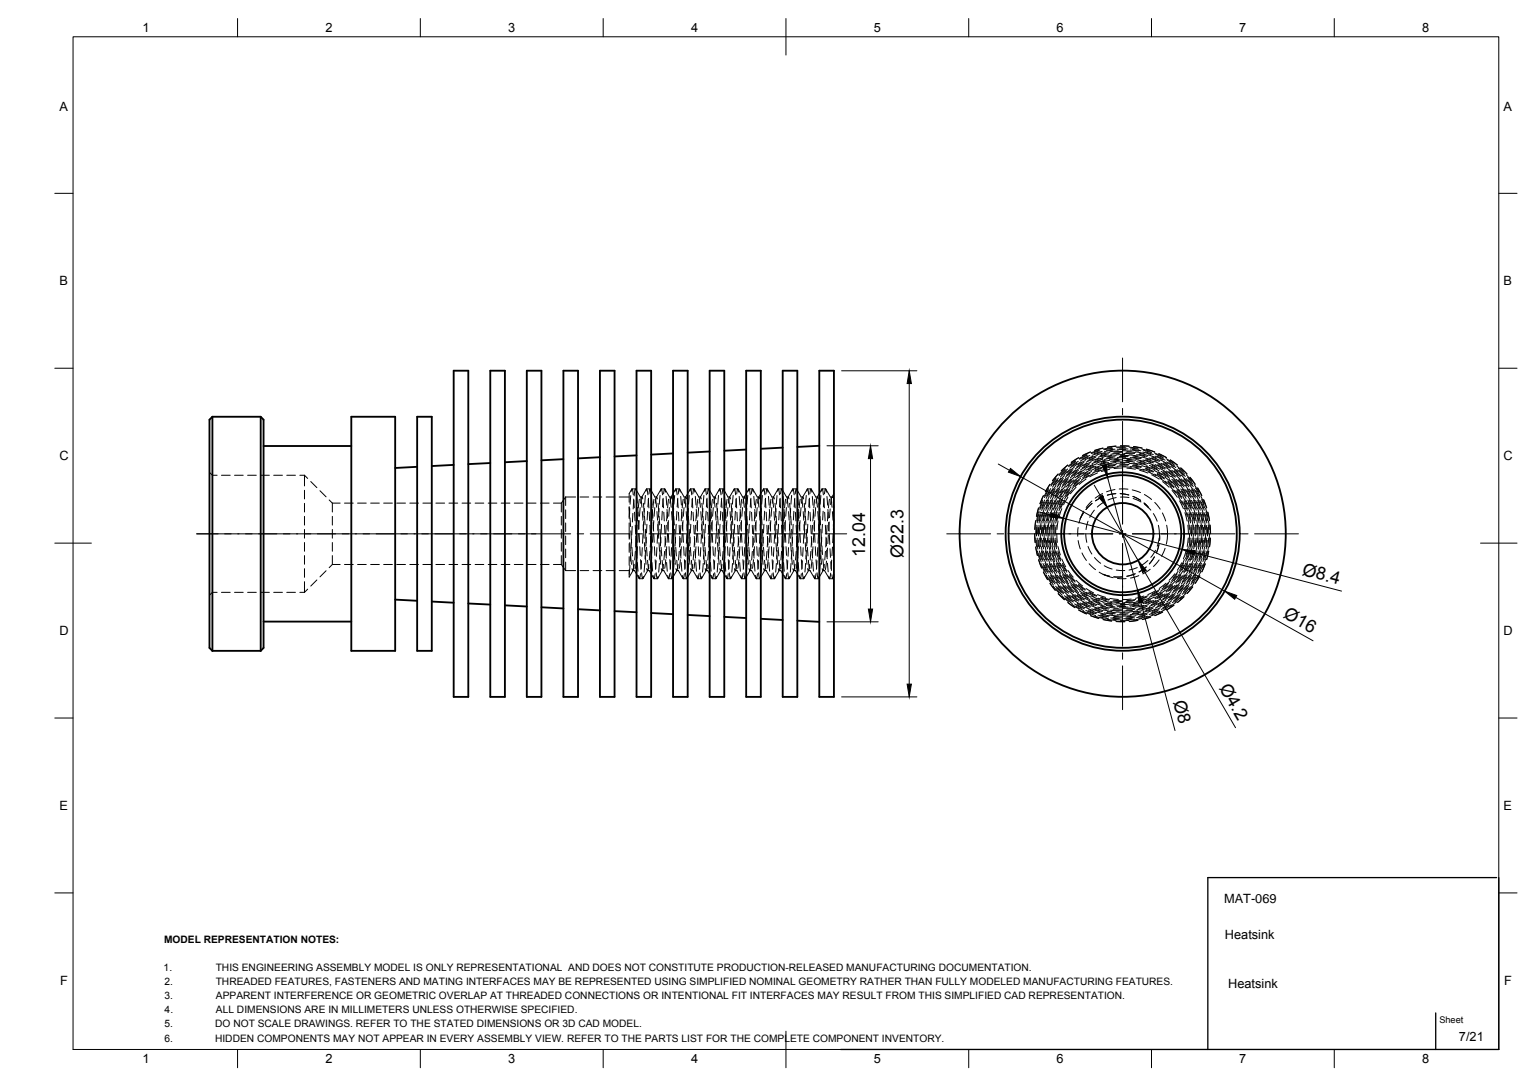
ISO-10303-21;
HEADER;
/* Generated by software containing ST-Developer
 * from STEP Tools, Inc. (www.steptools.com) 
 */

FILE_DESCRIPTION(
/* description */ ('CAx-IF Rec.Pracs.---Representation and Presentation of Product Manufa
cturing Information (PMI)---4.0---2014-10-13'),
/* implementation_level */ '2;1');

FILE_NAME(
/* name */ 'Heatsink.step',
/* time_stamp */ '2026-10-24T15:08:39-07:00',
/* author */ (''),
/* organization */ (''),
/* preprocessor_version */ 'ST-DEVELOPER v20.2',
/* originating_system */ 'Autodesk Translation Framework v15.17.0.0',
/* authorisation */ '');

FILE_SCHEMA (('AP242_MANAGED_MODEL_BASED_3D_ENGINEERING_MIM_LF { 1 0 10303 442 2 1 4 }'));
ENDSEC;

DATA;
#10=MECHANICAL_DESIGN_GEOMETRIC_PRESENTATION_REPRESENTATION('',(#824),#50081);
#94=B_SPLINE_SURFACE_WITH_KNOTS('',3,3,((#16932,#16933,#16934,#16935,#16936,
#16937,#16938,#16939,#16940,#16941,#16942,#16943,#16944,#16945,#16946,#16947,
#16948,#16949,#16950,#16951,#16952,#16953,#16954,#16955,#16956,#16957,#16958,
#16959,#16960,#16961,#16962,#16963,#16964,#16965,#16966,#16967,#16968,#16969,
#16970,#16971,#16972,#16973,#16974,#16975,#16976,#16977,#16978,#16979,#16980,
#16981,#16982,#16983,#16984,#16985,#16986,#16987,#16988,#16989,#16990,#16991,
#16992,#16993,#16994,#16995,#16996,#16997,#16998,#16999,#17000,#17001,#17002,
#17003,#17004,#17005,#17006,#17007,#17008,#17009,#17010,#17011,#17012,#17013,
#17014,#17015,#17016,#17017,#17018,#17019,#17020,#17021,#17022,#17023,#17024),
(#17025,#17026,#17027,#17028,#17029,#17030,#17031,#17032,#17033,#17034,
#17035,#17036,#17037,#17038,#17039,#17040,#17041,#17042,#17043,#17044,#17045,
#17046,#17047,#17048,#17049,#17050,#17051,#17052,#17053,#17054,#17055,#17056,
#17057,#17058,#17059,#17060,#17061,#17062,#17063,#17064,#17065,#17066,#17067,
#17068,#17069,#17070,#17071,#17072,#17073,#17074,#17075,#17076,#17077,#17078,
#17079,#17080,#17081,#17082,#17083,#17084,#17085,#17086,#17087,#17088,#17089,
#17090,#17091,#17092,#17093,#17094,#17095,#17096,#17097,#17098,#17099,#17100,
#17101,#17102,#17103,#17104,#17105,#17106,#17107,#17108,#17109,#17110,#17111,
#17112,#17113,#17114,#17115,#17116,#17117),(#17118,#17119,#17120,#17121,
#17122,#17123,#17124,#17125,#17126,#17127,#17128,#17129,#17130,#17131,#17132,
#17133,#17134,#17135,#17136,#17137,#17138,#17139,#17140,#17141,#17142,#17143,
#17144,#17145,#17146,#17147,#17148,#17149,#17150,#17151,#17152,#17153,#17154,
#17155,#17156,#17157,#17158,#17159,#17160,#17161,#17162,#17163,#17164,#17165,
#17166,#17167,#17168,#17169,#17170,#17171,#17172,#17173,#17174,#17175,#17176,
#17177,#17178,#17179,#17180,#17181,#17182,#17183,#17184,#17185,#17186,#17187,
#17188,#17189,#17190,#17191,#17192,#17193,#17194,#17195,#17196,#17197,#17198,
#17199,#17200,#17201,#17202,#17203,#17204,#17205,#17206,#17207,#17208,#17209,
#17210),(#17211,#17212,#17213,#17214,#17215,#17216,#17217,#17218,#17219,
#17220,#17221,#17222,#17223,#17224,#17225,#17226,#17227,#17228,#17229,#17230,
#17231,#17232,#17233,#17234,#17235,#17236,#17237,#17238,#17239,#17240,#17241,
#17242,#17243,#17244,#17245,#17246,#17247,#17248,#17249,#17250,#17251,#17252,
#17253,#17254,#17255,#17256,#17257,#17258,#17259,#17260,#17261,#17262,#17263,
#17264,#17265,#17266,#17267,#17268,#17269,#17270,#17271,#17272,#17273,#17274,
#17275,#17276,#17277,#17278,#17279,#17280,#17281,#17282,#17283,#17284,#17285,
#17286,#17287,#17288,#17289,#17290,#17291,#17292,#17293,#17294,#17295,#17296,
#17297,#17298,#17299,#17300,#17301,#17302,#17303)),.UNSPECIFIED.,.F.,.F.,
 .F.,(4,4),(4,1,1,1,1,1,1,1,1,1,1,1,1,1,1,1,1,1,1,1,1,1,1,1,1,1,1,1,1,1,
1,1,1,1,1,1,1,1,1,1,1,1,1,1,1,1,1,1,1,1,1,1,1,1,1,1,1,1,1,1,1,1,1,1,1,1,
1,1,1,1,1,1,1,1,1,1,1,1,1,1,1,1,1,1,1,1,1,1,1,1,4),(-0.000398919436546387,
0.0651101464894062),(10.2099830649134,11.2099710040949,12.2097658840232,
13.2095607639514,14.2093556438797,15.2091505238079,16.2089454037362,17.2087402836644,
18.2085351635927,19.208330043521,20.2081249234492,21.2079198033775,22.2077146833057,
23.207509563234,24.2073044431622,25.2070993230905,26.2068942030187,27.206689082947,
28.2064839628752,29.2062788428035,30.2060737227317,31.20586860266,32.2056634825882,
33.2054583625165,34.2052532424447,35.205048122373,36.2048430023012,37.2046378822295,
38.2044327621577,39.204227642086,40.2040225220142,41.2038174019425,42.2036122818707,
43.203407161799,44.2032020417273,45.2029969216555,46.2027918015838,47.202586681512,
48.2023815614403,49.2021764413685,50.2019713212968,51.201766201225,52.2015610811533,
53.2013559610815,54.2011508410098,55.200945720938,56.2007406008663,57.2005354807945,
58.2003303607228,59.200125240651,60.1999201205793,61.1997150005075,62.1995098804358,
63.199304760364,64.1990996402923,65.1988945202205,66.1986894001488,67.1984842800771,
68.1982791600053,69.1980740399336,70.1978689198618,71.1976637997901,72.1974586797183,
73.1972535596466,74.1970484395748,75.1968433195031,76.1966381994313,77.1964330793596,
78.1962279592878,79.1960228392161,80.1958177191443,81.1956125990726,82.1954074790008,
83.1952023589291,84.1949972388573,85.1947921187856,86.1945869987138,87.1943818786421,
88.1941767585704,89.1939716384986,90.1937665184269,91.1935613983551,92.1933562782833,
93.1931511582116,94.1929460381399,95.1927409180681,96.1925357979964,97.1923306779246,
98.1921255578529,99.1919204377811,100.192067891578),.UNSPECIFIED.);
#95=B_SPLINE_SURFACE_WITH_KNOTS('',3,3,((#17371,#17372,#17373,#17374,#17375,
#17376,#17377,#17378,#17379,#17380,#17381,#17382,#17383,#17384,#17385,#17386,
#17387,#17388,#17389,#17390,#17391,#17392,#17393,#17394,#17395,#17396,#17397,
#17398,#17399,#17400,#17401,#17402,#17403,#17404,#17405,#17406,#17407,#17408,
#17409,#17410,#17411,#17412,#17413,#17414,#17415,#17416,#17417,#17418,#17419,
#17420,#17421,#17422,#17423,#17424,#17425,#17426,#17427,#17428,#17429,#17430,
#17431,#17432,#17433,#17434,#17435,#17436,#17437,#17438,#17439,#17440,#17441,
#17442,#17443,#17444,#17445,#17446,#17447,#17448,#17449,#17450,#17451,#17452,
#17453,#17454,#17455,#17456,#17457,#17458,#17459,#17460,#17461,#17462,#17463),
(#17464,#17465,#17466,#17467,#17468,#17469,#17470,#17471,#17472,#17473,
#17474,#17475,#17476,#17477,#17478,#17479,#17480,#17481,#17482,#17483,#17484,
#17485,#17486,#17487,#17488,#17489,#17490,#17491,#17492,#17493,#17494,#17495,
#17496,#17497,#17498,#17499,#17500,#17501,#17502,#17503,#17504,#17505,#17506,
#17507,#17508,#17509,#17510,#17511,#17512,#17513,#17514,#17515,#17516,#17517,
#17518,#17519,#17520,#17521,#17522,#17523,#17524,#17525,#17526,#17527,#17528,
#17529,#17530,#17531,#17532,#17533,#17534,#17535,#17536,#17537,#17538,#17539,
#17540,#17541,#17542,#17543,#17544,#17545,#17546,#17547,#17548,#17549,#17550,
#17551,#17552,#17553,#17554,#17555,#17556),(#17557,#17558,#17559,#17560,
#17561,#17562,#17563,#17564,#17565,#17566,#17567,#17568,#17569,#17570,#17571,
#17572,#17573,#17574,#17575,#17576,#17577,#17578,#17579,#17580,#17581,#17582,
#17583,#17584,#17585,#17586,#17587,#17588,#17589,#17590,#17591,#17592,#17593,
#17594,#17595,#17596,#17597,#17598,#17599,#17600,#17601,#17602,#17603,#17604,
#17605,#17606,#17607,#17608,#17609,#17610,#17611,#17612,#17613,#17614,#17615,
#17616,#17617,#17618,#17619,#17620,#17621,#17622,#17623,#17624,#17625,#17626,
#17627,#17628,#17629,#17630,#17631,#17632,#17633,#17634,#17635,#17636,#17637,
#17638,#17639,#17640,#17641,#17642,#17643,#17644,#17645,#17646,#17647,#17648,
#17649),(#17650,#17651,#17652,#17653,#17654,#17655,#17656,#17657,#17658,
#17659,#17660,#17661,#17662,#17663,#17664,#17665,#17666,#17667,#17668,#17669,
#17670,#17671,#17672,#17673,#17674,#17675,#17676,#17677,#17678,#17679,#17680,
#17681,#17682,#17683,#17684,#17685,#17686,#17687,#17688,#17689,#17690,#17691,
#17692,#17693,#17694,#17695,#17696,#17697,#17698,#17699,#17700,#17701,#17702,
#17703,#17704,#17705,#17706,#17707,#17708,#17709,#17710,#17711,#17712,#17713,
#17714,#17715,#17716,#17717,#17718,#17719,#17720,#17721,#17722,#17723,#17724,
#17725,#17726,#17727,#17728,#17729,#17730,#17731,#17732,#17733,#17734,#17735,
#17736,#17737,#17738,#17739,#17740,#17741,#17742)),.UNSPECIFIED.,.F.,.F.,
 .F.,(4,4),(4,1,1,1,1,1,1,1,1,1,1,1,1,1,1,1,1,1,1,1,1,1,1,1,1,1,1,1,1,1,
1,1,1,1,1,1,1,1,1,1,1,1,1,1,1,1,1,1,1,1,1,1,1,1,1,1,1,1,1,1,1,1,1,1,1,1,
1,1,1,1,1,1,1,1,1,1,1,1,1,1,1,1,1,1,1,1,1,1,1,1,4),(-0.00100526872732246,
0.0646023829588572),(13.6909080459636,14.6908132548486,15.6906081347769,
16.6904030147051,17.6901978946334,18.6899927745616,19.6897876544899,20.6895825344181,
21.6893774143464,22.6891722942746,23.6889671742029,24.6887620541311,25.6885569340594,
26.6883518139876,27.6881466939159,28.6879415738441,29.6877364537724,30.6875313337007,
31.6873262136289,32.6871210935572,33.6869159734854,34.6867108534137,35.6865057333419,
36.6863006132702,37.6860954931984,38.6858903731267,39.6856852530549,40.6854801329832,
41.6852750129114,42.6850698928397,43.6848647727679,44.6846596526962,45.6844545326244,
46.6842494125527,47.6840442924809,48.6838391724092,49.6836340523375,50.6834289322657,
51.683223812194,52.6830186921222,53.6828135720505,54.6826084519787,55.682403331907,
56.6821982118352,57.6819930917635,58.6817879716917,59.68158285162,60.6813777315482,
61.6811726114765,62.6809674914047,63.680762371333,64.6805572512612,65.6803521311895,
66.6801470111178,67.679941891046,68.6797367709743,69.6795316509025,70.6793265308308,
71.679121410759,72.6789162906873,73.6787111706155,74.6785060505438,75.678300930472,
76.6780958104003,77.6778906903285,78.6776855702568,79.677480450185,80.6772753301133,
81.6770702100415,82.6768650899698,83.676659969898,84.6764548498263,85.6762497297545,
86.6760446096828,87.6758394896111,88.6756343695393,89.6754292494676,90.6752241293958,
91.6750190093241,92.6748138892523,93.6746087691806,94.6744036491088,95.6741985290371,
96.6739934089653,97.6737882888936,98.6735831688218,99.6733780487501,100.673172928678,
101.672967808607,102.672762688535,103.67278623601),.UNSPECIFIED.);
#141=B_SPLINE_CURVE_WITH_KNOTS('',3,(#13868,#13869,#13870,#13871,#13872,
#13873,#13874,#13875,#13876,#13877,#13878,#13879,#13880,#13881,#13882,#13883,
#13884,#13885,#13886,#13887,#13888,#13889,#13890,#13891,#13892,#13893,#13894,
#13895,#13896,#13897,#13898,#13899,#13900,#13901,#13902,#13903,#13904,#13905,
#13906,#13907,#13908,#13909,#13910,#13911,#13912,#13913,#13914,#13915,#13916,
#13917,#13918,#13919,#13920,#13921,#13922,#13923,#13924,#13925,#13926,#13927,
#13928,#13929,#13930,#13931,#13932,#13933,#13934),.UNSPECIFIED.,.F.,.F.,
(4,3,3,3,3,3,3,3,3,3,3,3,3,3,3,3,3,3,3,3,3,3,4),(1.25156093680116E-6,0.0883500955934641,
0.103030521980099,0.125,0.211544670578705,0.25,0.26221619397553,0.334021572169558,
0.375,0.421693572098901,0.485226135902788,0.5,0.5625,0.577874060665358,
0.625,0.710303391755808,0.734738255635071,0.75,0.836904432795506,0.875,
0.895553090245324,0.965961016411946,0.99999868984544),.UNSPECIFIED.);
#142=B_SPLINE_CURVE_WITH_KNOTS('',3,(#13936,#13937,#13938,#13939,#13940,
#13941,#13942,#13943,#13944,#13945,#13946,#13947,#13948,#13949,#13950,#13951,
#13952,#13953,#13954,#13955,#13956,#13957,#13958,#13959,#13960,#13961,#13962,
#13963,#13964,#13965,#13966,#13967,#13968,#13969,#13970,#13971,#13972,#13973,
#13974,#13975,#13976,#13977,#13978,#13979,#13980,#13981,#13982,#13983,#13984),
 .UNSPECIFIED.,.F.,.F.,(4,3,3,3,3,3,3,3,3,3,3,3,3,3,3,3,4),(0.,0.0880924990179859,
0.125,0.211469534154412,0.25,0.336789345136967,0.375,0.461773033582195,
0.5,0.586773033582203,0.625,0.711789345136965,0.75,0.836469534154423,0.875,
0.963092499017944,1.),.UNSPECIFIED.);
#143=B_SPLINE_CURVE_WITH_KNOTS('',3,(#13986,#13987,#13988,#13989,#13990,
#13991,#13992,#13993,#13994,#13995,#13996,#13997,#13998,#13999,#14000,#14001,
#14002,#14003,#14004,#14005,#14006,#14007,#14008,#14009,#14010,#14011,#14012,
#14013,#14014,#14015,#14016,#14017,#14018,#14019,#14020,#14021,#14022,#14023,
#14024,#14025,#14026,#14027,#14028,#14029,#14030,#14031,#14032,#14033,#14034),
 .UNSPECIFIED.,.F.,.F.,(4,3,3,3,3,3,3,3,3,3,3,3,3,3,3,3,4),(0.,0.0881024108360804,
0.125,0.211479598204264,0.25,0.336799405951737,0.375,0.461783076602685,
0.5,0.586783076602703,0.625,0.711799405951738,0.75,0.836479598204259,0.875,
0.963102410836136,1.),.UNSPECIFIED.);
#144=B_SPLINE_CURVE_WITH_KNOTS('',3,(#14036,#14037,#14038,#14039,#14040,
#14041,#14042,#14043,#14044,#14045,#14046,#14047,#14048,#14049,#14050,#14051,
#14052,#14053,#14054,#14055,#14056,#14057,#14058,#14059,#14060,#14061,#14062,
#14063,#14064,#14065,#14066,#14067,#14068,#14069,#14070,#14071,#14072,#14073,
#14074,#14075,#14076,#14077,#14078,#14079,#14080,#14081,#14082,#14083,#14084),
 .UNSPECIFIED.,.F.,.F.,(4,3,3,3,3,3,3,3,3,3,3,3,3,3,3,3,4),(0.,0.0880833098674038,
0.125,0.211460203849926,0.25,0.336780017823431,0.375,0.461763722773403,
0.5,0.586763722773395,0.625,0.71178001782344,0.75,0.836460203849939,0.875,
0.963083309867389,1.),.UNSPECIFIED.);
#145=B_SPLINE_CURVE_WITH_KNOTS('',3,(#14086,#14087,#14088,#14089,#14090,
#14091,#14092,#14093,#14094,#14095,#14096,#14097,#14098,#14099,#14100,#14101,
#14102,#14103,#14104,#14105,#14106,#14107,#14108,#14109,#14110,#14111,#14112,
#14113,#14114,#14115,#14116,#14117,#14118,#14119,#14120,#14121,#14122,#14123,
#14124,#14125,#14126,#14127,#14128,#14129,#14130,#14131,#14132,#14133,#14134),
 .UNSPECIFIED.,.F.,.F.,(4,3,3,3,3,3,3,3,3,3,3,3,3,3,3,3,4),(1.38656343410957E-7,
0.0880826036576598,0.125,0.211459358145887,0.25,0.336779172390087,0.375,
0.461762878836428,0.5,0.586762878836416,0.625,0.711779172390097,0.75,0.836459358145886,
0.875,0.963082476958599,1.),.UNSPECIFIED.);
#146=B_SPLINE_CURVE_WITH_KNOTS('',3,(#14136,#14137,#14138,#14139,#14140,
#14141,#14142,#14143,#14144,#14145,#14146,#14147,#14148,#14149,#14150,#14151,
#14152,#14153,#14154,#14155,#14156,#14157,#14158,#14159,#14160,#14161,#14162,
#14163,#14164,#14165,#14166,#14167,#14168,#14169,#14170,#14171,#14172,#14173,
#14174,#14175,#14176,#14177,#14178,#14179,#14180,#14181,#14182,#14183,#14184),
 .UNSPECIFIED.,.F.,.F.,(4,3,3,3,3,3,3,3,3,3,3,3,3,3,3,3,4),(0.,0.0881011169934676,
0.125,0.211478284491326,0.25,0.336798092661633,0.375,0.461781765634862,
0.5,0.586781765634871,0.625,0.711798092661628,0.75,0.836478284491337,0.875,
0.963101116993472,1.),.UNSPECIFIED.);
#147=B_SPLINE_CURVE_WITH_KNOTS('',3,(#14186,#14187,#14188,#14189,#14190,
#14191,#14192,#14193,#14194,#14195,#14196,#14197,#14198,#14199,#14200,#14201,
#14202,#14203,#14204,#14205,#14206,#14207,#14208,#14209,#14210,#14211,#14212,
#14213,#14214,#14215,#14216,#14217,#14218,#14219,#14220,#14221,#14222,#14223,
#14224,#14225,#14226,#14227,#14228,#14229,#14230,#14231,#14232,#14233,#14234),
 .UNSPECIFIED.,.F.,.F.,(4,3,3,3,3,3,3,3,3,3,3,3,3,3,3,3,4),(0.,0.0880934980383074,
0.125,0.211470548519371,0.25,0.336790359176268,0.375,0.461774045827613,
0.5,0.586774045827619,0.625,0.711790359176272,0.75,0.836470548519377,0.875,
0.963093498038292,1.),.UNSPECIFIED.);
#148=B_SPLINE_CURVE_WITH_KNOTS('',3,(#14236,#14237,#14238,#14239,#14240,
#14241,#14242,#14243,#14244,#14245,#14246,#14247,#14248,#14249,#14250,#14251,
#14252,#14253,#14254,#14255,#14256,#14257,#14258,#14259,#14260,#14261,#14262,
#14263,#14264,#14265,#14266,#14267,#14268,#14269,#14270,#14271,#14272,#14273,
#14274,#14275,#14276,#14277,#14278,#14279,#14280,#14281,#14282,#14283,#14284),
 .UNSPECIFIED.,.F.,.F.,(4,3,3,3,3,3,3,3,3,3,3,3,3,3,3,3,4),(1.23038810336374E-6,
0.0880827430507262,0.125,0.211461811736442,0.25,0.336784839496599,0.375,
0.461710040665769,0.5,0.586886602165314,0.625,0.711701462151024,0.75,0.836461636546894,
0.875,0.963080200121549,0.999998752114935),.UNSPECIFIED.);
#149=B_SPLINE_CURVE_WITH_KNOTS('',3,(#14286,#14287,#14288,#14289,#14290,
#14291,#14292,#14293,#14294,#14295,#14296,#14297,#14298,#14299,#14300,#14301,
#14302,#14303,#14304,#14305,#14306,#14307,#14308,#14309,#14310,#14311,#14312,
#14313,#14314,#14315,#14316,#14317,#14318,#14319,#14320,#14321,#14322,#14323,
#14324,#14325,#14326,#14327,#14328,#14329,#14330,#14331,#14332,#14333,#14334),
 .UNSPECIFIED.,.F.,.F.,(4,3,3,3,3,3,3,3,3,3,3,3,3,3,3,3,4),(0.,0.0880920072316036,
0.125,0.211469034814287,0.25,0.336788845957097,0.375,0.46177253528545,0.5,
0.586772535285452,0.625,0.711788845957101,0.75,0.836469034814284,0.875,
0.963092007231635,1.),.UNSPECIFIED.);
#150=B_SPLINE_CURVE_WITH_KNOTS('',3,(#14336,#14337,#14338,#14339,#14340,
#14341,#14342,#14343,#14344,#14345,#14346,#14347,#14348,#14349,#14350,#14351,
#14352,#14353,#14354,#14355,#14356,#14357,#14358,#14359,#14360,#14361,#14362,
#14363,#14364,#14365,#14366,#14367,#14368,#14369,#14370,#14371,#14372,#14373,
#14374,#14375,#14376,#14377,#14378,#14379,#14380,#14381,#14382,#14383,#14384),
 .UNSPECIFIED.,.F.,.F.,(4,3,3,3,3,3,3,3,3,3,3,3,3,3,3,3,4),(0.,0.0881029814297449,
0.125,0.211480177560658,0.25,0.33679998512162,0.375,0.461783654748482,0.5,
0.586783654748484,0.625,0.711799985121625,0.75,0.836480177560661,0.875,
0.963102981429744,1.),.UNSPECIFIED.);
#151=B_SPLINE_CURVE_WITH_KNOTS('',3,(#14386,#14387,#14388,#14389,#14390,
#14391,#14392),.UNSPECIFIED.,.F.,.F.,(4,1,1,1,4),(0.,0.25,0.5,0.75,1.),
 .UNSPECIFIED.);
#152=B_SPLINE_CURVE_WITH_KNOTS('',3,(#14396,#14397,#14398,#14399,#14400,
#14401,#14402,#14403,#14404,#14405,#14406,#14407,#14408,#14409,#14410,#14411,
#14412,#14413,#14414,#14415,#14416,#14417,#14418,#14419,#14420,#14421,#14422,
#14423,#14424,#14425,#14426,#14427,#14428,#14429,#14430,#14431,#14432),
 .UNSPECIFIED.,.F.,.F.,(4,3,3,3,3,3,3,3,3,3,3,3,4),(0.,0.125,0.23032997709698,
0.25,0.375,0.46468733129745,0.5,0.625,0.699111355030774,0.75,0.875,0.933549171352441,
1.),.UNSPECIFIED.);
#153=B_SPLINE_CURVE_WITH_KNOTS('',3,(#14434,#14435,#14436,#14437,#14438,
#14439,#14440,#14441,#14442,#14443,#14444,#14445,#14446,#14447,#14448,#14449,
#14450,#14451,#14452,#14453,#14454,#14455,#14456,#14457,#14458,#14459,#14460,
#14461,#14462,#14463,#14464,#14465,#14466,#14467,#14468,#14469,#14470,#14471,
#14472,#14473,#14474,#14475,#14476,#14477,#14478,#14479,#14480,#14481,#14482),
 .UNSPECIFIED.,.F.,.F.,(4,3,3,3,3,3,3,3,3,3,3,3,3,3,3,3,4),(7.72207807885717E-7,
0.0880871484364614,0.125,0.211463406241229,0.25,0.336781091047344,0.375,
0.461774857659637,0.5,0.586773708011755,0.625,0.711753540165089,0.75,0.836456686852539,
0.875,0.963077282795441,0.999999115125707),.UNSPECIFIED.);
#154=B_SPLINE_CURVE_WITH_KNOTS('',3,(#14484,#14485,#14486,#14487,#14488,
#14489,#14490,#14491,#14492,#14493,#14494,#14495,#14496,#14497,#14498,#14499,
#14500,#14501,#14502,#14503,#14504,#14505,#14506,#14507,#14508,#14509,#14510,
#14511,#14512,#14513,#14514,#14515,#14516,#14517,#14518,#14519,#14520,#14521,
#14522,#14523,#14524,#14525,#14526,#14527,#14528,#14529,#14530,#14531,#14532),
 .UNSPECIFIED.,.F.,.F.,(4,3,3,3,3,3,3,3,3,3,3,3,3,3,3,3,4),(0.,0.088088017626471,
0.125,0.211464983927167,0.25,0.336784796369337,0.375,0.461768492862693,
0.5,0.586768492862716,0.625,0.711784796369325,0.75,0.836464983927168,0.875,
0.96308801762646,1.),.UNSPECIFIED.);
#155=B_SPLINE_CURVE_WITH_KNOTS('',3,(#14534,#14535,#14536,#14537,#14538,
#14539,#14540,#14541,#14542,#14543,#14544,#14545,#14546,#14547,#14548,#14549,
#14550,#14551,#14552,#14553,#14554,#14555,#14556,#14557,#14558,#14559,#14560,
#14561,#14562,#14563,#14564,#14565,#14566,#14567,#14568,#14569,#14570,#14571,
#14572,#14573,#14574,#14575,#14576,#14577,#14578,#14579,#14580,#14581,#14582),
 .UNSPECIFIED.,.F.,.F.,(4,3,3,3,3,3,3,3,3,3,3,3,3,3,3,3,4),(0.,0.0881042788052708,
0.125,0.211481494860136,0.25,0.336801301996907,0.375,0.461784969295354,
0.5,0.586784969295344,0.625,0.711801301996906,0.75,0.836481494860131,0.875,
0.963104278805279,1.),.UNSPECIFIED.);
#156=B_SPLINE_CURVE_WITH_KNOTS('',3,(#14584,#14585,#14586,#14587,#14588,
#14589,#14590,#14591,#14592,#14593,#14594,#14595,#14596,#14597,#14598,#14599,
#14600,#14601,#14602,#14603,#14604,#14605,#14606,#14607,#14608,#14609,#14610,
#14611,#14612,#14613,#14614,#14615,#14616,#14617,#14618,#14619,#14620,#14621,
#14622,#14623,#14624,#14625,#14626,#14627,#14628,#14629,#14630,#14631,#14632),
 .UNSPECIFIED.,.F.,.F.,(4,3,3,3,3,3,3,3,3,3,3,3,3,3,3,3,4),(0.,0.0880886602034345,
0.125,0.211465636374609,0.25,0.336785448607603,0.375,0.461769143946861,
0.5,0.586769143946859,0.625,0.711785448607598,0.75,0.83646563637461,0.875,
0.963088660203419,1.),.UNSPECIFIED.);
#157=B_SPLINE_CURVE_WITH_KNOTS('',3,(#14634,#14635,#14636,#14637,#14638,
#14639,#14640,#14641,#14642,#14643,#14644,#14645,#14646,#14647,#14648,#14649,
#14650,#14651,#14652,#14653,#14654,#14655,#14656,#14657,#14658,#14659,#14660,
#14661,#14662,#14663,#14664,#14665,#14666,#14667,#14668,#14669,#14670,#14671,
#14672,#14673,#14674,#14675,#14676,#14677,#14678,#14679,#14680,#14681,#14682,
#14683,#14684,#14685,#14686,#14687,#14688,#14689,#14690,#14691,#14692,#14693,
#14694,#14695,#14696,#14697,#14698,#14699,#14700,#14701,#14702,#14703,#14704,
#14705,#14706,#14707,#14708,#14709),.UNSPECIFIED.,.F.,.F.,(4,3,3,3,3,3,
3,3,3,3,3,3,3,3,3,3,3,3,3,3,3,3,3,3,3,4),(9.70948605131889E-7,0.0875075598981359,
0.125,0.211923873410919,0.25,0.3125,0.375,0.40625,0.4375,0.46875,0.484375,
0.4921875,0.5,0.5078125,0.515625,0.53125,0.5625,0.59375,0.625,0.6875,0.75,
0.8125,0.875,0.9375,0.995806240197456,0.999999425592883),.UNSPECIFIED.);
#158=B_SPLINE_CURVE_WITH_KNOTS('',3,(#14711,#14712,#14713,#14714,#14715,
#14716,#14717,#14718,#14719,#14720,#14721,#14722,#14723,#14724,#14725,#14726,
#14727,#14728,#14729,#14730,#14731,#14732,#14733,#14734,#14735,#14736,#14737,
#14738,#14739,#14740,#14741,#14742,#14743,#14744,#14745,#14746,#14747,#14748,
#14749,#14750,#14751,#14752,#14753,#14754,#14755,#14756,#14757,#14758,#14759),
 .UNSPECIFIED.,.F.,.F.,(4,3,3,3,3,3,3,3,3,3,3,3,3,3,3,3,4),(0.,0.088095309895002,
0.125,0.211472388204989,0.25,0.336792198271045,0.375,0.461775881669146,
0.5,0.586775881669135,0.625,0.711792198271046,0.75,0.836472388204994,0.875,
0.963095309894954,1.),.UNSPECIFIED.);
#159=B_SPLINE_CURVE_WITH_KNOTS('',3,(#14761,#14762,#14763,#14764,#14765,
#14766,#14767,#14768,#14769,#14770,#14771,#14772,#14773,#14774,#14775,#14776,
#14777,#14778,#14779,#14780,#14781,#14782,#14783,#14784,#14785,#14786,#14787,
#14788,#14789,#14790,#14791,#14792,#14793,#14794,#14795,#14796,#14797,#14798,
#14799,#14800,#14801,#14802,#14803,#14804,#14805,#14806,#14807,#14808,#14809),
 .UNSPECIFIED.,.F.,.F.,(4,3,3,3,3,3,3,3,3,3,3,3,3,3,3,3,4),(0.,0.088096458191059,
0.125,0.211473554137782,0.25,0.336793363829213,0.375,0.461777045165672,
0.5,0.586777045165651,0.625,0.711793363829219,0.75,0.836473554137771,0.875,
0.963096458191102,1.),.UNSPECIFIED.);
#160=B_SPLINE_CURVE_WITH_KNOTS('',3,(#14811,#14812,#14813,#14814,#14815,
#14816,#14817,#14818,#14819,#14820,#14821,#14822,#14823,#14824,#14825,#14826,
#14827,#14828,#14829,#14830,#14831,#14832,#14833,#14834,#14835,#14836,#14837,
#14838,#14839,#14840,#14841,#14842,#14843,#14844,#14845,#14846,#14847,#14848,
#14849,#14850,#14851,#14852,#14853,#14854,#14855,#14856,#14857,#14858,#14859),
 .UNSPECIFIED.,.F.,.F.,(4,3,3,3,3,3,3,3,3,3,3,3,3,3,3,3,4),(6.48233978329073E-7,
0.088087481714971,0.125,0.211463563406532,0.25,0.336780768905252,0.375,
0.461780695889845,0.5,0.586763634796104,0.625,0.711758226647009,0.75,0.836456256382313,
0.875,0.963077038983795,0.9999992074512),.UNSPECIFIED.);
#161=B_SPLINE_CURVE_WITH_KNOTS('',3,(#14861,#14862,#14863,#14864,#14865,
#14866,#14867,#14868,#14869,#14870,#14871,#14872,#14873,#14874,#14875,#14876,
#14877,#14878,#14879,#14880,#14881,#14882,#14883,#14884,#14885,#14886,#14887,
#14888,#14889,#14890,#14891,#14892,#14893,#14894,#14895,#14896,#14897,#14898,
#14899,#14900,#14901,#14902,#14903,#14904,#14905,#14906,#14907,#14908,#14909),
 .UNSPECIFIED.,.F.,.F.,(4,3,3,3,3,3,3,3,3,3,3,3,3,3,3,3,4),(0.,0.0880873565129711,
0.125,0.211464312658339,0.25,0.33678412531568,0.375,0.461767822996489,0.5,
0.586767822996495,0.625,0.711784125315678,0.75,0.836464312658332,0.875,
0.963087356512997,1.),.UNSPECIFIED.);
#162=B_SPLINE_CURVE_WITH_KNOTS('',3,(#14911,#14912,#14913,#14914,#14915,
#14916,#14917,#14918,#14919,#14920,#14921,#14922,#14923,#14924,#14925,#14926,
#14927,#14928,#14929,#14930,#14931,#14932,#14933,#14934,#14935,#14936,#14937,
#14938,#14939,#14940,#14941,#14942,#14943,#14944,#14945,#14946,#14947,#14948,
#14949,#14950,#14951,#14952,#14953,#14954,#14955,#14956,#14957,#14958,#14959),
 .UNSPECIFIED.,.F.,.F.,(4,3,3,3,3,3,3,3,3,3,3,3,3,3,3,3,4),(0.,0.0881042076361416,
0.125,0.211481422598089,0.25,0.336801229758134,0.375,0.461784897184286,
0.5,0.586784897184306,0.625,0.71180122975812,0.75,0.836481422598088,0.875,
0.963104207636176,1.),.UNSPECIFIED.);
#163=B_SPLINE_CURVE_WITH_KNOTS('',3,(#14961,#14962,#14963,#14964,#14965,
#14966,#14967,#14968,#14969,#14970,#14971,#14972,#14973,#14974,#14975,#14976,
#14977,#14978,#14979,#14980,#14981,#14982,#14983,#14984,#14985,#14986,#14987,
#14988,#14989,#14990,#14991,#14992,#14993,#14994,#14995,#14996,#14997,#14998,
#14999,#15000,#15001,#15002,#15003,#15004,#15005,#15006,#15007,#15008,#15009),
 .UNSPECIFIED.,.F.,.F.,(4,3,3,3,3,3,3,3,3,3,3,3,3,3,3,3,4),(0.,0.0880892870445733,
0.125,0.21146627284444,0.25,0.336786084873347,0.375,0.461769779086792,0.5,
0.586769779086777,0.625,0.711786084873348,0.75,0.836466272844441,0.875,
0.963089287044564,1.),.UNSPECIFIED.);
#164=B_SPLINE_CURVE_WITH_KNOTS('',3,(#15011,#15012,#15013,#15014,#15015,
#15016,#15017,#15018,#15019,#15020,#15021,#15022,#15023,#15024,#15025,#15026,
#15027,#15028,#15029,#15030,#15031,#15032,#15033,#15034,#15035,#15036,#15037,
#15038,#15039,#15040,#15041,#15042,#15043,#15044,#15045,#15046,#15047,#15048,
#15049,#15050,#15051,#15052,#15053,#15054,#15055,#15056,#15057,#15058,#15059,
#15060,#15061,#15062,#15063,#15064,#15065,#15066,#15067,#15068,#15069,#15070,
#15071,#15072,#15073,#15074,#15075,#15076,#15077,#15078,#15079,#15080,#15081,
#15082,#15083),.UNSPECIFIED.,.F.,.F.,(4,3,3,3,3,3,3,3,3,3,3,3,3,3,3,3,3,
3,3,3,3,3,3,3,4),(1.04553770632841E-6,0.0875080165836233,0.125,0.211924214406689,
0.25,0.3125,0.375,0.40625,0.4375,0.46875,0.484375,0.4921875,0.5,0.5078125,
0.515625,0.53125,0.5625,0.59375,0.625,0.6875,0.75,0.8125,0.875,0.9375,0.999999334390892),
 .UNSPECIFIED.);
#165=B_SPLINE_CURVE_WITH_KNOTS('',3,(#15085,#15086,#15087,#15088,#15089,
#15090,#15091,#15092,#15093,#15094,#15095,#15096,#15097,#15098,#15099,#15100,
#15101,#15102,#15103,#15104,#15105,#15106,#15107,#15108,#15109,#15110,#15111,
#15112,#15113,#15114,#15115,#15116,#15117,#15118,#15119,#15120,#15121,#15122,
#15123,#15124,#15125,#15126,#15127,#15128,#15129,#15130,#15131,#15132,#15133),
 .UNSPECIFIED.,.F.,.F.,(4,3,3,3,3,3,3,3,3,3,3,3,3,3,3,3,4),(0.,0.0880950608203889,
0.125,0.211472135304815,0.25,0.33679194545211,0.375,0.461775629297404,0.5,
0.58677562929742,0.625,0.711791945452102,0.75,0.836472135304814,0.875,0.963095060820362,
1.),.UNSPECIFIED.);
#166=B_SPLINE_CURVE_WITH_KNOTS('',3,(#15135,#15136,#15137,#15138,#15139,
#15140,#15141,#15142,#15143,#15144,#15145,#15146,#15147,#15148,#15149,#15150,
#15151,#15152,#15153),.UNSPECIFIED.,.F.,.F.,(4,3,3,3,3,3,4),(0.,0.00857368461051335,
0.25,0.5,0.504408674649204,0.75,1.),.UNSPECIFIED.);
#167=B_SPLINE_CURVE_WITH_KNOTS('',3,(#15157,#15158,#15159,#15160,#15161,
#15162,#15163,#15164,#15165,#15166,#15167,#15168,#15169,#15170,#15171,#15172,
#15173,#15174,#15175,#15176,#15177,#15178,#15179,#15180,#15181,#15182,#15183,
#15184,#15185,#15186,#15187,#15188,#15189,#15190),.UNSPECIFIED.,.F.,.F.,
(4,3,3,3,3,3,3,3,3,3,3,4),(0.,0.158394062068541,0.25,0.282388204951903,
0.404806937739057,0.5,0.569551910301168,0.654806937739066,0.75,0.856807890509175,
0.908394062068542,1.),.UNSPECIFIED.);
#168=B_SPLINE_CURVE_WITH_KNOTS('',3,(#15192,#15193,#15194,#15195,#15196,
#15197,#15198,#15199,#15200,#15201,#15202,#15203,#15204,#15205,#15206,#15207,
#15208,#15209,#15210,#15211,#15212,#15213,#15214,#15215,#15216,#15217,#15218,
#15219,#15220,#15221,#15222,#15223,#15224,#15225,#15226,#15227,#15228,#15229,
#15230,#15231,#15232,#15233,#15234,#15235,#15236,#15237,#15238,#15239,#15240),
 .UNSPECIFIED.,.F.,.F.,(4,3,3,3,3,3,3,3,3,3,3,3,3,3,3,3,4),(3.26471858241762E-8,
0.0880825316349779,0.125,0.21145938337219,0.25,0.336779197608326,0.375,
0.461762904010005,0.5,0.586762904010012,0.625,0.711779197608325,0.75,0.836459383372186,
0.875,0.963082501803219,1.),.UNSPECIFIED.);
#169=B_SPLINE_CURVE_WITH_KNOTS('',3,(#15242,#15243,#15244,#15245,#15246,
#15247,#15248,#15249,#15250,#15251,#15252,#15253,#15254,#15255,#15256,#15257,
#15258,#15259,#15260,#15261,#15262,#15263,#15264,#15265,#15266,#15267,#15268,
#15269,#15270,#15271,#15272,#15273,#15274,#15275,#15276,#15277,#15278,#15279,
#15280,#15281,#15282,#15283,#15284,#15285,#15286,#15287,#15288,#15289,#15290),
 .UNSPECIFIED.,.F.,.F.,(4,3,3,3,3,3,3,3,3,3,3,3,3,3,3,3,4),(0.,0.0881017307290489,
0.125,0.211478907652486,0.25,0.336798715622224,0.375,0.461782387493885,
0.5,0.586782387493868,0.625,0.711798715622233,0.75,0.836478907652487,0.875,
0.963101730729054,1.),.UNSPECIFIED.);
#170=B_SPLINE_CURVE_WITH_KNOTS('',3,(#15291,#15292,#15293,#15294,#15295,
#15296,#15297,#15298,#15299,#15300,#15301,#15302,#15303,#15304,#15305,#15306,
#15307,#15308,#15309,#15310,#15311,#15312,#15313,#15314,#15315,#15316,#15317,
#15318,#15319,#15320,#15321,#15322,#15323,#15324,#15325,#15326,#15327,#15328,
#15329,#15330,#15331,#15332,#15333,#15334,#15335,#15336,#15337,#15338,#15339),
 .UNSPECIFIED.,.F.,.F.,(4,3,3,3,3,3,3,3,3,3,3,3,3,3,3,3,4),(0.,0.0880930729141991,
0.125,0.211470116865539,0.25,0.336789927661028,0.375,0.461773615075734,
0.5,0.586773615075741,0.625,0.711789927661028,0.75,0.836470116865545,0.875,
0.963093072914204,1.),.UNSPECIFIED.);
#171=B_SPLINE_CURVE_WITH_KNOTS('',3,(#15343,#15344,#15345,#15346,#15347,
#15348,#15349,#15350,#15351,#15352,#15353,#15354,#15355,#15356,#15357,#15358,
#15359,#15360,#15361,#15362,#15363,#15364,#15365,#15366,#15367,#15368,#15369,
#15370,#15371,#15372,#15373,#15374,#15375,#15376,#15377,#15378,#15379,#15380,
#15381,#15382,#15383,#15384,#15385,#15386,#15387,#15388,#15389,#15390,#15391,
#15392,#15393,#15394,#15395,#15396,#15397,#15398,#15399,#15400,#15401,#15402,
#15403,#15404,#15405,#15406,#15407,#15408,#15409,#15410,#15411,#15412,#15413,
#15414,#15415,#15416,#15417,#15418),.UNSPECIFIED.,.F.,.F.,(4,3,3,3,3,3,
3,3,3,3,3,3,3,3,3,3,3,3,3,3,3,3,3,3,3,4),(7.93458957479051E-7,0.0919827770270099,
0.125,0.21636947259665,0.25,0.3125,0.375,0.40625,0.4375,0.46875,0.484375,
0.4921875,0.5,0.5078125,0.515625,0.53125,0.5625,0.59375,0.625,0.6875,0.75,
0.8125,0.875,0.9375,0.992573279862854,0.999999611514097),.UNSPECIFIED.);
#172=B_SPLINE_CURVE_WITH_KNOTS('',3,(#15420,#15421,#15422,#15423,#15424,
#15425,#15426,#15427,#15428,#15429,#15430,#15431,#15432,#15433,#15434,#15435,
#15436,#15437,#15438,#15439,#15440,#15441,#15442,#15443,#15444,#15445,#15446,
#15447,#15448,#15449,#15450,#15451,#15452,#15453,#15454,#15455,#15456,#15457,
#15458,#15459,#15460,#15461,#15462,#15463,#15464,#15465,#15466,#15467,#15468),
 .UNSPECIFIED.,.F.,.F.,(4,3,3,3,3,3,3,3,3,3,3,3,3,3,3,3,4),(0.,0.0926028564089548,
0.125,0.215896935943174,0.25,0.341233104859871,0.375,0.466215951447718,
0.5,0.591215951447998,0.625,0.716233104860131,0.75,0.840896935943215,0.875,
0.967602856408858,1.),.UNSPECIFIED.);
#173=B_SPLINE_CURVE_WITH_KNOTS('',3,(#15470,#15471,#15472,#15473,#15474,
#15475,#15476,#15477,#15478,#15479,#15480,#15481,#15482,#15483,#15484,#15485,
#15486,#15487,#15488,#15489,#15490,#15491,#15492,#15493,#15494,#15495,#15496,
#15497,#15498,#15499,#15500,#15501,#15502,#15503,#15504,#15505,#15506,#15507,
#15508,#15509,#15510,#15511,#15512,#15513,#15514,#15515,#15516,#15517,#15518),
 .UNSPECIFIED.,.F.,.F.,(4,3,3,3,3,3,3,3,3,3,3,3,3,3,3,3,4),(0.,0.0926016482516165,
0.125,0.215895709229479,0.25,0.341231878540584,0.375,0.466214727297818,
0.5,0.591214727297569,0.625,0.716231878540515,0.75,0.840895709229348,0.875,
0.967601648251421,1.),.UNSPECIFIED.);
#174=B_SPLINE_CURVE_WITH_KNOTS('',3,(#15520,#15521,#15522,#15523,#15524,
#15525,#15526,#15527,#15528,#15529,#15530,#15531,#15532,#15533,#15534,#15535,
#15536,#15537,#15538,#15539,#15540,#15541,#15542,#15543,#15544,#15545,#15546,
#15547,#15548,#15549,#15550,#15551,#15552,#15553),.UNSPECIFIED.,.F.,.F.,
(4,2,2,2,2,2,2,2,2,2,2,2,2,2,2,2,4),(8.60008680714194E-7,0.0925922496141415,
0.125,0.215885936189025,0.25,0.341220868711526,0.375,0.466201529424218,
0.5,0.59123334097936,0.625,0.71618155918904,0.75,0.84088010118624,0.875,
0.967583301320753,0.99999903411916),.UNSPECIFIED.);
#175=B_SPLINE_CURVE_WITH_KNOTS('',3,(#15555,#15556,#15557,#15558,#15559,
#15560,#15561,#15562,#15563,#15564,#15565,#15566,#15567,#15568,#15569,#15570,
#15571,#15572,#15573,#15574,#15575,#15576,#15577,#15578,#15579,#15580,#15581,
#15582,#15583,#15584,#15585,#15586,#15587,#15588,#15589,#15590,#15591,#15592,
#15593,#15594,#15595,#15596,#15597,#15598,#15599,#15600,#15601,#15602,#15603),
 .UNSPECIFIED.,.F.,.F.,(4,3,3,3,3,3,3,3,3,3,3,3,3,3,3,3,4),(0.,0.0925946446316686,
0.125,0.215888598034351,0.25,0.341224769627743,0.375,0.466207630961137,
0.5,0.591207630961336,0.625,0.716224769627659,0.75,0.840888598034289,0.875,
0.967594644631377,1.),.UNSPECIFIED.);
#176=B_SPLINE_CURVE_WITH_KNOTS('',3,(#15605,#15606,#15607,#15608,#15609,
#15610,#15611,#15612,#15613,#15614,#15615,#15616,#15617,#15618,#15619,#15620,
#15621,#15622,#15623,#15624,#15625,#15626,#15627,#15628,#15629,#15630,#15631,
#15632,#15633,#15634,#15635,#15636,#15637,#15638,#15639,#15640,#15641,#15642,
#15643,#15644,#15645,#15646,#15647,#15648,#15649,#15650,#15651,#15652,#15653),
 .UNSPECIFIED.,.F.,.F.,(4,3,3,3,3,3,3,3,3,3,3,3,3,3,3,3,4),(0.,0.0926110770714553,
0.125,0.215905282857406,0.25,0.341241449089134,0.375,0.466224280920412,
0.5,0.591224280920756,0.625,0.716241449088887,0.75,0.840905282857528,0.875,
0.967611077071527,1.),.UNSPECIFIED.);
#177=B_SPLINE_CURVE_WITH_KNOTS('',3,(#15655,#15656,#15657,#15658,#15659,
#15660,#15661,#15662,#15663,#15664,#15665,#15666,#15667,#15668,#15669,#15670,
#15671,#15672,#15673,#15674,#15675,#15676,#15677,#15678,#15679,#15680,#15681,
#15682,#15683,#15684,#15685,#15686,#15687,#15688,#15689,#15690,#15691,#15692,
#15693,#15694,#15695,#15696,#15697,#15698,#15699,#15700,#15701,#15702,#15703),
 .UNSPECIFIED.,.F.,.F.,(4,3,3,3,3,3,3,3,3,3,3,3,3,3,3,3,4),(0.,0.0925939685908668,
0.125,0.215887911608834,0.25,0.341224083422187,0.375,0.466206945970056,
0.5,0.591206945970017,0.625,0.716224083422156,0.75,0.840887911608889,0.875,
0.967593968591154,1.),.UNSPECIFIED.);
#178=B_SPLINE_CURVE_WITH_KNOTS('',3,(#15705,#15706,#15707,#15708,#15709,
#15710,#15711,#15712,#15713,#15714,#15715,#15716,#15717,#15718,#15719,#15720,
#15721,#15722,#15723,#15724,#15725,#15726,#15727,#15728,#15729,#15730,#15731,
#15732,#15733,#15734,#15735,#15736,#15737,#15738,#15739,#15740,#15741,#15742,
#15743,#15744,#15745,#15746,#15747,#15748,#15749,#15750,#15751,#15752,#15753,
#15754,#15755,#15756,#15757,#15758,#15759,#15760,#15761,#15762,#15763,#15764,
#15765,#15766,#15767,#15768,#15769,#15770,#15771,#15772,#15773,#15774,#15775,
#15776,#15777,#15778,#15779,#15780),.UNSPECIFIED.,.F.,.F.,(4,3,3,3,3,3,
3,3,3,3,3,3,3,3,3,3,3,3,3,3,3,3,3,3,3,4),(8.85984697358488E-7,0.0919833162888678,
0.125,0.216369876637167,0.25,0.3125,0.375,0.40625,0.4375,0.46875,0.484375,
0.4921875,0.5,0.5078125,0.515625,0.53125,0.5625,0.59375,0.625,0.6875,0.75,
0.8125,0.875,0.9375,0.995501429491965,0.999999512663293),.UNSPECIFIED.);
#179=B_SPLINE_CURVE_WITH_KNOTS('',3,(#15782,#15783,#15784,#15785,#15786,
#15787,#15788,#15789,#15790,#15791,#15792,#15793,#15794,#15795,#15796,#15797,
#15798,#15799,#15800,#15801,#15802,#15803,#15804,#15805,#15806,#15807,#15808,
#15809,#15810,#15811,#15812,#15813,#15814,#15815,#15816,#15817,#15818,#15819,
#15820,#15821,#15822,#15823,#15824,#15825,#15826,#15827,#15828,#15829,#15830),
 .UNSPECIFIED.,.F.,.F.,(4,3,3,3,3,3,3,3,3,3,3,3,3,3,3,3,4),(0.,0.0926016640197792,
0.125,0.215895725240053,0.25,0.341231894546074,0.375,0.466214743274479,
0.5,0.591214743274513,0.625,0.71623189454608,0.75,0.840895725240135,0.875,
0.96760166401992,0.99999999999941),.UNSPECIFIED.);
#180=B_SPLINE_CURVE_WITH_KNOTS('',3,(#15834,#15835,#15836,#15837,#15838,
#15839,#15840),.UNSPECIFIED.,.F.,.F.,(4,3,4),(3.02475966928685E-5,0.761300445681502,
0.999991310305325),.UNSPECIFIED.);
#181=B_SPLINE_CURVE_WITH_KNOTS('',3,(#15842,#15843,#15844,#15845,#15846,
#15847,#15848,#15849,#15850,#15851,#15852,#15853,#15854,#15855,#15856,#15857,
#15858,#15859,#15860,#15861,#15862,#15863,#15864,#15865,#15866,#15867,#15868,
#15869,#15870,#15871,#15872,#15873,#15874,#15875,#15876,#15877,#15878,#15879,
#15880,#15881,#15882,#15883,#15884,#15885,#15886,#15887,#15888,#15889,#15890),
 .UNSPECIFIED.,.F.,.F.,(4,3,3,3,3,3,3,3,3,3,3,3,3,3,3,3,4),(0.,0.0926097133311401,
0.125,0.215903898174036,0.25,0.341240064851683,0.375,0.466222899130803,
0.5,0.591222899130775,0.625,0.716240064851504,0.75,0.840903898174011,0.875,
0.967609713331501,1.),.UNSPECIFIED.);
#182=B_SPLINE_CURVE_WITH_KNOTS('',3,(#15892,#15893,#15894,#15895,#15896,
#15897,#15898,#15899,#15900,#15901,#15902,#15903,#15904,#15905,#15906,#15907,
#15908,#15909,#15910,#15911,#15912,#15913,#15914,#15915,#15916,#15917,#15918,
#15919,#15920,#15921,#15922,#15923,#15924,#15925,#15926,#15927,#15928,#15929,
#15930,#15931,#15932,#15933,#15934,#15935,#15936,#15937,#15938,#15939,#15940),
 .UNSPECIFIED.,.F.,.F.,(4,3,3,3,3,3,3,3,3,3,3,3,3,3,3,3,4),(0.,0.0925981673177476,
0.125,0.215892174830268,0.25,0.3412283452762,0.375,0.466211200283384,0.5,
0.591211200283569,0.625,0.716228345276186,0.75,0.840892174830337,0.875,
0.967598167317428,1.),.UNSPECIFIED.);
#183=B_SPLINE_CURVE_WITH_KNOTS('',3,(#15942,#15943,#15944,#15945,#15946,
#15947,#15948,#15949,#15950,#15951,#15952,#15953,#15954,#15955,#15956,#15957,
#15958,#15959,#15960,#15961,#15962,#15963,#15964,#15965,#15966,#15967,#15968,
#15969,#15970,#15971,#15972,#15973,#15974,#15975,#15976,#15977,#15978,#15979,
#15980,#15981,#15982,#15983,#15984,#15985,#15986,#15987,#15988,#15989,#15990,
#15991,#15992,#15993),.UNSPECIFIED.,.F.,.F.,(4,3,3,3,3,3,3,3,3,3,3,3,3,
3,3,3,3,4),(1.25053720846655E-6,0.0929545115982379,0.125,0.215420114878467,
0.25,0.339746875247112,0.375,0.4375,0.496741821459526,0.5,0.5625,0.625,
0.722152298803526,0.75,0.8373366708814,0.875,0.959989006508124,0.999998883500357),
 .UNSPECIFIED.);
#184=B_SPLINE_CURVE_WITH_KNOTS('',3,(#15995,#15996,#15997,#15998,#15999,
#16000,#16001,#16002,#16003,#16004,#16005,#16006,#16007,#16008,#16009,#16010,
#16011,#16012,#16013,#16014,#16015,#16016,#16017,#16018,#16019,#16020,#16021,
#16022,#16023,#16024,#16025,#16026,#16027,#16028,#16029,#16030,#16031,#16032,
#16033,#16034,#16035,#16036,#16037,#16038,#16039,#16040,#16041,#16042,#16043),
 .UNSPECIFIED.,.F.,.F.,(4,3,3,3,3,3,3,3,3,3,3,3,3,3,3,3,4),(0.,0.09259973745462,
0.125,0.215893769083908,0.25,0.341229939018056,0.375,0.466212791205734,
0.5,0.591212791205995,0.625,0.716229939018014,0.75,0.840893769083763,0.875,
0.967599737454784,1.),.UNSPECIFIED.);
#185=B_SPLINE_CURVE_WITH_KNOTS('',3,(#16045,#16046,#16047,#16048,#16049,
#16050,#16051,#16052,#16053,#16054,#16055,#16056,#16057,#16058,#16059,#16060,
#16061,#16062,#16063,#16064,#16065,#16066,#16067,#16068,#16069,#16070,#16071,
#16072,#16073,#16074,#16075,#16076,#16077,#16078,#16079,#16080,#16081,#16082,
#16083,#16084,#16085,#16086,#16087,#16088,#16089,#16090,#16091,#16092,#16093),
 .UNSPECIFIED.,.F.,.F.,(4,3,3,3,3,3,3,3,3,3,3,3,3,3,3,3,4),(0.,0.0926077535236005,
0.125,0.215901908268581,0.25,0.341238075586479,0.375,0.4662209133831,0.5,
0.591220913383166,0.625,0.716238075586483,0.75,0.840901908268568,0.875,
0.967607753523283,1.),.UNSPECIFIED.);
#186=B_SPLINE_CURVE_WITH_KNOTS('',3,(#16095,#16096,#16097,#16098,#16099,
#16100,#16101,#16102,#16103,#16104,#16105,#16106,#16107,#16108,#16109,#16110,
#16111,#16112,#16113,#16114,#16115,#16116,#16117,#16118,#16119,#16120,#16121,
#16122,#16123,#16124,#16125,#16126,#16127,#16128,#16129,#16130,#16131,#16132,
#16133,#16134,#16135,#16136,#16137,#16138,#16139,#16140,#16141,#16142,#16143),
 .UNSPECIFIED.,.F.,.F.,(4,3,3,3,3,3,3,3,3,3,3,3,3,3,3,3,4),(0.,0.0925881405225714,
0.125,0.21588199401248,0.25,0.341218167721451,0.375,0.466201040738566,0.5,
0.591201040738367,0.625,0.716218167721304,0.75,0.840881994012549,0.875,
0.967588139527948,0.999999861566054),.UNSPECIFIED.);
#187=B_SPLINE_CURVE_WITH_KNOTS('',3,(#16145,#16146,#16147,#16148,#16149,
#16150,#16151,#16152,#16153,#16154,#16155,#16156,#16157,#16158,#16159,#16160,
#16161,#16162,#16163,#16164,#16165,#16166,#16167,#16168,#16169,#16170,#16171,
#16172,#16173,#16174,#16175,#16176,#16177,#16178,#16179,#16180,#16181,#16182,
#16183,#16184,#16185,#16186,#16187,#16188,#16189,#16190,#16191,#16192,#16193),
 .UNSPECIFIED.,.F.,.F.,(4,3,3,3,3,3,3,3,3,3,3,3,3,3,3,3,4),(0.,0.0925890173961925,
0.125,0.215882884356336,0.25,0.34121905778002,0.375,0.46620192922203,0.5,
0.591201929222098,0.625,0.716219057780218,0.75,0.840882884356031,0.875,
0.967589017395721,1.),.UNSPECIFIED.);
#188=B_SPLINE_CURVE_WITH_KNOTS('',3,(#16195,#16196,#16197,#16198,#16199,
#16200,#16201,#16202,#16203,#16204,#16205,#16206,#16207,#16208,#16209,#16210,
#16211,#16212,#16213,#16214,#16215,#16216,#16217,#16218,#16219,#16220,#16221,
#16222,#16223,#16224,#16225,#16226,#16227,#16228,#16229,#16230,#16231,#16232,
#16233,#16234,#16235,#16236,#16237,#16238,#16239,#16240,#16241,#16242,#16243),
 .UNSPECIFIED.,.F.,.F.,(4,3,3,3,3,3,3,3,3,3,3,3,3,3,3,3,4),(0.,0.0926091135500264,
0.125,0.215903289181841,0.25,0.341239456055151,0.375,0.466222291411168,
0.5,0.59122229141116,0.625,0.716239456055371,0.75,0.840903289181801,0.875,
0.967609113549421,1.),.UNSPECIFIED.);
#189=B_SPLINE_CURVE_WITH_KNOTS('',3,(#16245,#16246,#16247,#16248,#16249,
#16250,#16251,#16252,#16253,#16254,#16255,#16256,#16257,#16258,#16259,#16260,
#16261,#16262,#16263,#16264,#16265,#16266,#16267,#16268,#16269,#16270,#16271,
#16272,#16273,#16274,#16275,#16276,#16277,#16278,#16279,#16280,#16281,#16282,
#16283,#16284,#16285,#16286,#16287,#16288,#16289,#16290,#16291,#16292,#16293),
 .UNSPECIFIED.,.F.,.F.,(4,3,3,3,3,3,3,3,3,3,3,3,3,3,3,3,4),(0.,0.0925986851494203,
0.125,0.215892700615775,0.25,0.341228870892842,0.375,0.466211724970258,
0.5,0.59121172497034,0.625,0.716228870892888,0.75,0.840892700615926,0.875,
0.967598685149769,1.),.UNSPECIFIED.);
#190=B_SPLINE_CURVE_WITH_KNOTS('',3,(#16295,#16296,#16297,#16298,#16299,
#16300,#16301,#16302,#16303,#16304,#16305,#16306,#16307,#16308,#16309,#16310,
#16311,#16312,#16313,#16314,#16315,#16316,#16317,#16318,#16319,#16320,#16321,
#16322,#16323,#16324,#16325,#16326,#16327,#16328,#16329,#16330,#16331,#16332,
#16333,#16334,#16335,#16336,#16337,#16338,#16339,#16340),.UNSPECIFIED.,
 .F.,.F.,(4,3,3,3,3,3,3,3,3,3,3,3,3,3,3,4),(1.25824916392832E-6,0.0923454433051621,
0.125,0.216129877093308,0.25,0.342613529803912,0.375,0.457998148773538,
0.5,0.625,0.714780278674796,0.75,0.839601858305807,0.875,0.964995303736524,
0.999998796399913),.UNSPECIFIED.);
#191=B_SPLINE_CURVE_WITH_KNOTS('',3,(#16342,#16343,#16344,#16345,#16346,
#16347,#16348,#16349,#16350,#16351,#16352,#16353,#16354,#16355,#16356,#16357,
#16358,#16359,#16360,#16361,#16362,#16363,#16364,#16365,#16366,#16367,#16368,
#16369,#16370,#16371,#16372,#16373,#16374,#16375,#16376,#16377,#16378,#16379,
#16380,#16381,#16382,#16383,#16384,#16385,#16386,#16387,#16388,#16389,#16390),
 .UNSPECIFIED.,.F.,.F.,(4,3,3,3,3,3,3,3,3,3,3,3,3,3,3,3,4),(0.,0.0925992895932416,
0.125,0.215893314343291,0.25,0.341229484423304,0.375,0.46621233741587,0.5,
0.591212337415676,0.625,0.716229484423541,0.75,0.840893314343279,0.875,
0.967599289593344,1.),.UNSPECIFIED.);
#192=B_SPLINE_CURVE_WITH_KNOTS('',3,(#16392,#16393,#16394,#16395,#16396,
#16397,#16398,#16399,#16400,#16401,#16402,#16403,#16404,#16405,#16406,#16407,
#16408,#16409,#16410,#16411,#16412,#16413,#16414,#16415,#16416,#16417,#16418,
#16419,#16420,#16421,#16422,#16423,#16424,#16425,#16426,#16427,#16428,#16429,
#16430,#16431,#16432,#16433,#16434,#16435,#16436,#16437,#16438,#16439,#16440),
 .UNSPECIFIED.,.F.,.F.,(4,3,3,3,3,3,3,3,3,3,3,3,3,3,3,3,4),(0.,0.0926083986537193,
0.125,0.215902563306285,0.25,0.341238730413271,0.375,0.466221567052477,
0.5,0.59122156705239,0.625,0.716238730413398,0.75,0.840902563306212,0.875,
0.967608398653425,1.),.UNSPECIFIED.);
#193=B_SPLINE_CURVE_WITH_KNOTS('',3,(#16442,#16443,#16444,#16445,#16446,
#16447,#16448,#16449,#16450,#16451,#16452,#16453,#16454,#16455,#16456,#16457,
#16458,#16459,#16460,#16461,#16462,#16463,#16464,#16465,#16466,#16467,#16468,
#16469,#16470,#16471,#16472,#16473,#16474,#16475,#16476,#16477,#16478,#16479,
#16480,#16481,#16482,#16483,#16484,#16485,#16486,#16487,#16488,#16489,#16490),
 .UNSPECIFIED.,.F.,.F.,(4,3,3,3,3,3,3,3,3,3,3,3,3,3,3,3,4),(0.,0.0925881676381304,
0.125,0.215882021544404,0.25,0.341218195244346,0.375,0.466201068212794,
0.5,0.591201068212782,0.625,0.716218195244376,0.75,0.840882021544444,0.875,
0.96758816740381,0.999999967401505),.UNSPECIFIED.);
#194=B_SPLINE_CURVE_WITH_KNOTS('',3,(#16492,#16493,#16494,#16495,#16496,
#16497,#16498,#16499,#16500,#16501,#16502,#16503,#16504,#16505,#16506,#16507,
#16508,#16509,#16510,#16511,#16512,#16513,#16514,#16515,#16516,#16517,#16518,
#16519,#16520,#16521,#16522,#16523,#16524,#16525,#16526,#16527,#16528,#16529,
#16530,#16531,#16532,#16533,#16534,#16535,#16536,#16537,#16538,#16539,#16540),
 .UNSPECIFIED.,.F.,.F.,(4,3,3,3,3,3,3,3,3,3,3,3,3,3,3,3,4),(0.,0.106287359337513,
0.125,0.229771416343439,0.25,0.355096911466,0.375,0.480061767793933,0.5,
0.605061767794126,0.625,0.730096911465622,0.75,0.854771416343529,0.875,
0.981287359338472,0.999999999999949),.UNSPECIFIED.);
#195=B_SPLINE_CURVE_WITH_KNOTS('',3,(#16544,#16545,#16546,#16547,#16548,
#16549,#16550,#16551,#16552,#16553,#16554,#16555,#16556,#16557,#16558,#16559,
#16560,#16561,#16562,#16563,#16564,#16565,#16566,#16567,#16568,#16569,#16570,
#16571,#16572,#16573,#16574,#16575,#16576,#16577,#16578,#16579,#16580,#16581,
#16582,#16583,#16584,#16585,#16586,#16587,#16588,#16589,#16590,#16591,#16592),
 .UNSPECIFIED.,.F.,.F.,(4,3,3,3,3,3,3,3,3,3,3,3,3,3,3,3,4),(4.5000019854714E-7,
0.0926018329307898,0.125,0.215895443114202,0.25,0.341231612510821,0.375,
0.466214461738461,0.5,0.591214461738094,0.625,0.716231612510757,0.75,0.840895443114331,
0.875,0.967601386161383,1.),.UNSPECIFIED.);
#196=B_SPLINE_CURVE_WITH_KNOTS('',3,(#16594,#16595,#16596,#16597,#16598,
#16599,#16600,#16601,#16602,#16603,#16604,#16605,#16606,#16607,#16608,#16609,
#16610,#16611,#16612,#16613,#16614,#16615,#16616,#16617,#16618,#16619,#16620,
#16621,#16622,#16623,#16624,#16625,#16626,#16627),.UNSPECIFIED.,.F.,.F.,
(4,2,2,2,2,2,2,2,2,2,2,2,2,2,2,2,4),(9.46277652146847E-7,0.0925916484161767,
0.125,0.215885706168785,0.25,0.34122139386794,0.375,0.466192349791288,0.5,
0.591249283254599,0.625,0.716174174210448,0.75,0.840880794969292,0.875,
0.967583711036726,0.99999896009837),.UNSPECIFIED.);
#197=B_SPLINE_CURVE_WITH_KNOTS('',3,(#16629,#16630,#16631,#16632,#16633,
#16634,#16635,#16636,#16637,#16638,#16639,#16640,#16641,#16642,#16643,#16644,
#16645,#16646,#16647,#16648,#16649,#16650,#16651,#16652,#16653,#16654,#16655,
#16656,#16657,#16658,#16659,#16660,#16661,#16662,#16663,#16664,#16665,#16666,
#16667,#16668,#16669,#16670,#16671,#16672,#16673,#16674,#16675,#16676,#16677),
 .UNSPECIFIED.,.F.,.F.,(4,3,3,3,3,3,3,3,3,3,3,3,3,3,3,3,4),(0.,0.0925953041831434,
0.125,0.215889267717039,0.25,0.341225439095757,0.375,0.466208299244986,
0.5,0.591208299244716,0.625,0.716225439095638,0.75,0.840889267717158,0.875,
0.96759530418352,1.),.UNSPECIFIED.);
#198=B_SPLINE_CURVE_WITH_KNOTS('',3,(#16679,#16680,#16681,#16682,#16683,
#16684,#16685,#16686,#16687,#16688,#16689,#16690,#16691,#16692,#16693,#16694,
#16695,#16696,#16697,#16698,#16699,#16700,#16701,#16702,#16703,#16704,#16705,
#16706,#16707,#16708,#16709,#16710,#16711,#16712,#16713,#16714,#16715,#16716,
#16717,#16718,#16719,#16720,#16721,#16722,#16723,#16724,#16725,#16726,#16727),
 .UNSPECIFIED.,.F.,.F.,(4,3,3,3,3,3,3,3,3,3,3,3,3,3,3,3,4),(0.,0.0926110022616626,
0.125,0.215905206898781,0.25,0.341241373155053,0.375,0.466224205121077,
0.5,0.591224205120857,0.625,0.716241373154821,0.75,0.840905206898693,0.875,
0.967611002261608,1.),.UNSPECIFIED.);
#199=B_SPLINE_CURVE_WITH_KNOTS('',3,(#16728,#16729,#16730,#16731,#16732,
#16733,#16734,#16735,#16736,#16737,#16738,#16739,#16740,#16741,#16742,#16743,
#16744,#16745,#16746,#16747,#16748,#16749,#16750,#16751,#16752,#16753,#16754,
#16755,#16756,#16757,#16758,#16759,#16760,#16761,#16762,#16763,#16764,#16765,
#16766,#16767,#16768,#16769,#16770,#16771,#16772,#16773,#16774,#16775,#16776),
 .UNSPECIFIED.,.F.,.F.,(4,3,3,3,3,3,3,3,3,3,3,3,3,3,3,3,4),(0.,0.0925932731175236,
0.125,0.215887205452251,0.25,0.34122337749192,0.375,0.466206241288816,0.5,
0.591206241289337,0.625,0.716223377492011,0.75,0.84088720545214,0.875,0.967593273117083,
1.),.UNSPECIFIED.);
#200=B_SPLINE_CURVE_WITH_KNOTS('',3,(#16822,#16823,#16824,#16825,#16826,
#16827,#16828,#16829,#16830,#16831,#16832,#16833,#16834,#16835,#16836,#16837,
#16838,#16839,#16840,#16841,#16842,#16843,#16844,#16845,#16846,#16847,#16848,
#16849,#16850,#16851,#16852,#16853,#16854,#16855,#16856,#16857,#16858,#16859,
#16860,#16861,#16862,#16863,#16864,#16865,#16866,#16867,#16868,#16869,#16870,
#16871,#16872,#16873,#16874,#16875,#16876),.UNSPECIFIED.,.F.,.F.,(4,3,3,
3,3,3,3,3,3,3,3,3,3,3,3,3,3,3,4),(-0.569248610399452,-0.543571759198363,
-0.510395599541255,-0.504799388975929,-0.45563601739013,-0.442602338909788,
-0.358452201979706,-0.343831278006888,-0.337469726455479,-0.308533410217098,
-0.30096067569989,-0.233918536086011,-0.22808143434137,-0.139754810098741,
-0.122954682021969,-0.117884022561589,-0.113367531001717,-0.00535378548456125,
-6.56921400347513E-5),.UNSPECIFIED.);
#201=B_SPLINE_CURVE_WITH_KNOTS('',3,(#16877,#16878,#16879,#16880,#16881,
#16882,#16883,#16884,#16885,#16886,#16887,#16888,#16889,#16890,#16891,#16892,
#16893,#16894,#16895,#16896,#16897,#16898,#16899,#16900,#16901,#16902,#16903,
#16904,#16905,#16906,#16907,#16908,#16909,#16910,#16911,#16912,#16913,#16914,
#16915,#16916,#16917,#16918,#16919,#16920,#16921,#16922,#16923,#16924,#16925,
#16926,#16927,#16928,#16929,#16930,#16931),.UNSPECIFIED.,.F.,.F.,(4,3,3,
3,3,3,3,3,3,3,3,3,3,3,3,3,3,3,4),(-0.566847306048063,-0.536663225899598,
-0.497463681658886,-0.490486608162161,-0.423989019112076,-0.41889779448436,
-0.317015916859763,-0.311568571461078,-0.307442392923327,-0.279475887950007,
-0.27234718303655,-0.21391709050398,-0.20477719839138,-0.200645503382732,
-0.117724865987957,-0.103391697089455,-0.0995431702903938,-0.00440105423172584,
0.),.UNSPECIFIED.);
#202=B_SPLINE_CURVE_WITH_KNOTS('',3,(#17304,#17305,#17306,#17307,#17308,
#17309,#17310,#17311,#17312,#17313,#17314,#17315,#17316,#17317,#17318,#17319,
#17320,#17321,#17322,#17323,#17324,#17325,#17326,#17327,#17328,#17329,#17330,
#17331,#17332,#17333,#17334,#17335,#17336,#17337,#17338,#17339,#17340,#17341,
#17342,#17343,#17344,#17345,#17346,#17347,#17348,#17349,#17350,#17351,#17352,
#17353,#17354,#17355,#17356,#17357,#17358,#17359,#17360,#17361,#17362,#17363,
#17364,#17365,#17366,#17367,#17368,#17369,#17370),.UNSPECIFIED.,.F.,.F.,
(4,3,3,3,3,3,3,3,3,3,3,3,3,3,3,3,3,3,3,3,3,3,4),(0.,0.0902263235284944,
0.0965695032982788,0.102693117565567,0.185183726670681,0.195784092223982,
0.201956945222684,0.206397101465053,0.235002111145181,0.263505425073497,
0.267460741436352,0.295373658448176,0.306667851934945,0.311356021489761,
0.402390498589277,0.414121393711446,0.422114271443368,0.426853739956178,
0.483056044923388,0.493852365850745,0.499811702366216,0.561514407519245,
0.566789965462338),.UNSPECIFIED.);
#203=B_SPLINE_CURVE_WITH_KNOTS('',3,(#17743,#17744,#17745,#17746,#17747,
#17748,#17749,#17750,#17751,#17752,#17753,#17754,#17755,#17756,#17757,#17758,
#17759,#17760,#17761,#17762,#17763,#17764,#17765,#17766,#17767,#17768,#17769,
#17770,#17771,#17772,#17773,#17774,#17775,#17776,#17777,#17778,#17779,#17780,
#17781,#17782,#17783,#17784,#17785,#17786,#17787,#17788,#17789,#17790,#17791,
#17792,#17793,#17794,#17795,#17796,#17797,#17798,#17799,#17800,#17801,#17802,
#17803,#17804,#17805,#17806),.UNSPECIFIED.,.F.,.F.,(4,3,3,3,3,3,3,3,3,3,
3,3,3,3,3,3,3,3,3,3,3,4),(0.,0.0297263173547245,0.115411427535913,0.120694019406524,
0.150458483605126,0.209056395204914,0.221568856508229,0.228760022478968,
0.23414409783388,0.290594481715472,0.296053478345246,0.325007652648377,
0.335794721522812,0.340099498092156,0.344569097461082,0.428539652510242,
0.441342004070912,0.446282536720056,0.507885976399662,0.513324701408156,
0.56483218923889,0.569248610399433),.UNSPECIFIED.);
#613=CONICAL_SURFACE('',#10273,0.0041,0.785398163397448);
#614=CONICAL_SURFACE('',#10281,0.0079,0.785398163397448);
#615=CONICAL_SURFACE('',#10288,0.0079,0.785398163397448);
#616=CONICAL_SURFACE('',#10289,0.00305,0.785398163397448);
#617=CONICAL_SURFACE('',#10296,0.0023,0.950546840812075);
#618=CONICAL_SURFACE('',#10351,0.0045,0.0523598775598298);
#619=CONICAL_SURFACE('',#10353,0.0045,0.0523598775598298);
#620=CONICAL_SURFACE('',#10354,0.0045,0.0523598775598298);
#621=CONICAL_SURFACE('',#10355,0.0045,0.0523598775598298);
#622=CONICAL_SURFACE('',#10356,0.0045,0.0523598775598298);
#623=CONICAL_SURFACE('',#10357,0.0045,0.0523598775598298);
#624=CONICAL_SURFACE('',#10358,0.0045,0.0523598775598298);
#625=CONICAL_SURFACE('',#10360,0.0045,0.0523598775598298);
#626=CONICAL_SURFACE('',#10363,0.0045,0.0523598775598298);
#627=CONICAL_SURFACE('',#10366,0.0045,0.0523598775598298);
#628=CONICAL_SURFACE('',#10369,0.0045,0.0523598775598298);
#629=CONICAL_SURFACE('',#10372,0.0045,0.0523598775598298);
#712=FACE_BOUND('',#1723,.T.);
#713=FACE_BOUND('',#1726,.T.);
#714=FACE_BOUND('',#1731,.T.);
#715=FACE_BOUND('',#1740,.T.);
#716=FACE_BOUND('',#1742,.T.);
#717=FACE_BOUND('',#1744,.T.);
#718=FACE_BOUND('',#1746,.T.);
#719=FACE_BOUND('',#1748,.T.);
#720=FACE_BOUND('',#1750,.T.);
#721=FACE_BOUND('',#1752,.T.);
#722=FACE_BOUND('',#1754,.T.);
#723=FACE_BOUND('',#1756,.T.);
#724=FACE_BOUND('',#1758,.T.);
#725=FACE_BOUND('',#1760,.T.);
#726=FACE_BOUND('',#1762,.T.);
#727=FACE_BOUND('',#1764,.T.);
#728=FACE_BOUND('',#1766,.T.);
#729=FACE_BOUND('',#1768,.T.);
#730=FACE_BOUND('',#1785,.T.);
#731=FACE_BOUND('',#1792,.T.);
#732=FACE_BOUND('',#1795,.T.);
#733=FACE_BOUND('',#1797,.T.);
#734=FACE_BOUND('',#1800,.T.);
#735=FACE_BOUND('',#1802,.T.);
#736=FACE_BOUND('',#1805,.T.);
#737=FACE_BOUND('',#1807,.T.);
#738=FACE_BOUND('',#1810,.T.);
#739=FACE_BOUND('',#1812,.T.);
#740=FACE_BOUND('',#1815,.T.);
#784=SHAPE_REPRESENTATION_RELATIONSHIP('SRR','None',#50152,#804);
#804=ADVANCED_BREP_SHAPE_REPRESENTATION('',(#844),#50065);
#824=STYLED_ITEM('',(#50261),#844);
#844=MANIFOLD_SOLID_BREP('Body1',#9869);
#912=PLANE('',#10276);
#913=PLANE('',#10286);
#914=PLANE('',#10295);
#915=PLANE('',#10297);
#916=PLANE('',#10300);
#917=PLANE('',#10303);
#918=PLANE('',#10306);
#919=PLANE('',#10309);
#920=PLANE('',#10312);
#921=PLANE('',#10315);
#922=PLANE('',#10318);
#923=PLANE('',#10321);
#924=PLANE('',#10324);
#925=PLANE('',#10327);
#926=PLANE('',#10330);
#927=PLANE('',#10333);
#928=PLANE('',#10336);
#929=PLANE('',#10339);
#930=PLANE('',#10359);
#931=PLANE('',#10373);
#932=PLANE('',#10377);
#933=PLANE('',#10378);
#934=PLANE('',#10382);
#935=PLANE('',#10383);
#936=PLANE('',#10387);
#937=PLANE('',#10388);
#938=PLANE('',#10392);
#939=PLANE('',#10393);
#940=PLANE('',#10398);
#1178=FACE_OUTER_BOUND('',#1721,.T.);
#1179=FACE_OUTER_BOUND('',#1722,.T.);
#1180=FACE_OUTER_BOUND('',#1724,.T.);
#1181=FACE_OUTER_BOUND('',#1725,.T.);
#1182=FACE_OUTER_BOUND('',#1727,.T.);
#1183=FACE_OUTER_BOUND('',#1728,.T.);
#1184=FACE_OUTER_BOUND('',#1729,.T.);
#1185=FACE_OUTER_BOUND('',#1730,.T.);
#1186=FACE_OUTER_BOUND('',#1732,.T.);
#1187=FACE_OUTER_BOUND('',#1733,.T.);
#1188=FACE_OUTER_BOUND('',#1734,.T.);
#1189=FACE_OUTER_BOUND('',#1735,.T.);
#1190=FACE_OUTER_BOUND('',#1736,.T.);
#1191=FACE_OUTER_BOUND('',#1737,.T.);
#1192=FACE_OUTER_BOUND('',#1738,.T.);
#1193=FACE_OUTER_BOUND('',#1739,.T.);
#1194=FACE_OUTER_BOUND('',#1741,.T.);
#1195=FACE_OUTER_BOUND('',#1743,.T.);
#1196=FACE_OUTER_BOUND('',#1745,.T.);
#1197=FACE_OUTER_BOUND('',#1747,.T.);
#1198=FACE_OUTER_BOUND('',#1749,.T.);
#1199=FACE_OUTER_BOUND('',#1751,.T.);
#1200=FACE_OUTER_BOUND('',#1753,.T.);
#1201=FACE_OUTER_BOUND('',#1755,.T.);
#1202=FACE_OUTER_BOUND('',#1757,.T.);
#1203=FACE_OUTER_BOUND('',#1759,.T.);
#1204=FACE_OUTER_BOUND('',#1761,.T.);
#1205=FACE_OUTER_BOUND('',#1763,.T.);
#1206=FACE_OUTER_BOUND('',#1765,.T.);
#1207=FACE_OUTER_BOUND('',#1767,.T.);
#1208=FACE_OUTER_BOUND('',#1769,.T.);
#1209=FACE_OUTER_BOUND('',#1770,.T.);
#1210=FACE_OUTER_BOUND('',#1771,.T.);
#1211=FACE_OUTER_BOUND('',#1772,.T.);
#1212=FACE_OUTER_BOUND('',#1773,.T.);
#1213=FACE_OUTER_BOUND('',#1774,.T.);
#1214=FACE_OUTER_BOUND('',#1775,.T.);
#1215=FACE_OUTER_BOUND('',#1776,.T.);
#1216=FACE_OUTER_BOUND('',#1777,.T.);
#1217=FACE_OUTER_BOUND('',#1778,.T.);
#1218=FACE_OUTER_BOUND('',#1779,.T.);
#1219=FACE_OUTER_BOUND('',#1780,.T.);
#1220=FACE_OUTER_BOUND('',#1781,.T.);
#1221=FACE_OUTER_BOUND('',#1782,.T.);
#1222=FACE_OUTER_BOUND('',#1783,.T.);
#1223=FACE_OUTER_BOUND('',#1784,.T.);
#1224=FACE_OUTER_BOUND('',#1786,.T.);
#1225=FACE_OUTER_BOUND('',#1787,.T.);
#1226=FACE_OUTER_BOUND('',#1788,.T.);
#1227=FACE_OUTER_BOUND('',#1789,.T.);
#1228=FACE_OUTER_BOUND('',#1790,.T.);
#1229=FACE_OUTER_BOUND('',#1791,.T.);
#1230=FACE_OUTER_BOUND('',#1793,.T.);
#1231=FACE_OUTER_BOUND('',#1794,.T.);
#1232=FACE_OUTER_BOUND('',#1796,.T.);
#1233=FACE_OUTER_BOUND('',#1798,.T.);
#1234=FACE_OUTER_BOUND('',#1799,.T.);
#1235=FACE_OUTER_BOUND('',#1801,.T.);
#1236=FACE_OUTER_BOUND('',#1803,.T.);
#1237=FACE_OUTER_BOUND('',#1804,.T.);
#1238=FACE_OUTER_BOUND('',#1806,.T.);
#1239=FACE_OUTER_BOUND('',#1808,.T.);
#1240=FACE_OUTER_BOUND('',#1809,.T.);
#1241=FACE_OUTER_BOUND('',#1811,.T.);
#1242=FACE_OUTER_BOUND('',#1813,.T.);
#1243=FACE_OUTER_BOUND('',#1814,.T.);
#1244=FACE_OUTER_BOUND('',#1816,.T.);
#1721=EDGE_LOOP('',(#6582,#6583,#6584,#6585,#6586,#6587,#6588,#6589,#6590,
#6591,#6592,#6593,#6594,#6595,#6596,#6597,#6598,#6599,#6600,#6601,#6602,
#6603,#6604,#6605,#6606,#6607,#6608,#6609,#6610,#6611,#6612,#6613));
#1722=EDGE_LOOP('',(#6614,#6615,#6616,#6617,#6618,#6619,#6620,#6621,#6622,
#6623,#6624,#6625,#6626,#6627,#6628,#6629,#6630,#6631,#6632,#6633,#6634,
#6635,#6636,#6637,#6638,#6639,#6640,#6641,#6642,#6643,#6644));
#1723=EDGE_LOOP('',(#6645));
#1724=EDGE_LOOP('',(#6646,#6647,#6648,#6649));
#1725=EDGE_LOOP('',(#6650));
#1726=EDGE_LOOP('',(#6651));
#1727=EDGE_LOOP('',(#6652,#6653,#6654,#6655,#6656));
#1728=EDGE_LOOP('',(#6657,#6658,#6659,#6660));
#1729=EDGE_LOOP('',(#6661,#6662,#6663,#6664));
#1730=EDGE_LOOP('',(#6665));
#1731=EDGE_LOOP('',(#6666));
#1732=EDGE_LOOP('',(#6667,#6668,#6669,#6670));
#1733=EDGE_LOOP('',(#6671,#6672,#6673,#6674,#6675,#6676));
#1734=EDGE_LOOP('',(#6677,#6678,#6679,#6680,#6681,#6682));
#1735=EDGE_LOOP('',(#6683,#6684,#6685,#6686));
#1736=EDGE_LOOP('',(#6687,#6688,#6689,#6690,#6691,#6692,#6693,#6694,#6695,
#6696,#6697,#6698,#6699,#6700,#6701,#6702,#6703,#6704,#6705,#6706,#6707,
#6708,#6709,#6710,#6711,#6712,#6713,#6714,#6715,#6716,#6717,#6718));
#1737=EDGE_LOOP('',(#6719,#6720,#6721,#6722,#6723,#6724,#6725,#6726,#6727,
#6728,#6729,#6730,#6731,#6732,#6733,#6734,#6735,#6736,#6737,#6738,#6739,
#6740,#6741,#6742,#6743,#6744,#6745,#6746,#6747,#6748,#6749));
#1738=EDGE_LOOP('',(#6750,#6751,#6752,#6753,#6754));
#1739=EDGE_LOOP('',(#6755));
#1740=EDGE_LOOP('',(#6756));
#1741=EDGE_LOOP('',(#6757));
#1742=EDGE_LOOP('',(#6758));
#1743=EDGE_LOOP('',(#6759));
#1744=EDGE_LOOP('',(#6760));
#1745=EDGE_LOOP('',(#6761));
#1746=EDGE_LOOP('',(#6762));
#1747=EDGE_LOOP('',(#6763));
#1748=EDGE_LOOP('',(#6764));
#1749=EDGE_LOOP('',(#6765));
#1750=EDGE_LOOP('',(#6766));
#1751=EDGE_LOOP('',(#6767));
#1752=EDGE_LOOP('',(#6768));
#1753=EDGE_LOOP('',(#6769));
#1754=EDGE_LOOP('',(#6770));
#1755=EDGE_LOOP('',(#6771));
#1756=EDGE_LOOP('',(#6772));
#1757=EDGE_LOOP('',(#6773));
#1758=EDGE_LOOP('',(#6774));
#1759=EDGE_LOOP('',(#6775));
#1760=EDGE_LOOP('',(#6776));
#1761=EDGE_LOOP('',(#6777));
#1762=EDGE_LOOP('',(#6778));
#1763=EDGE_LOOP('',(#6779));
#1764=EDGE_LOOP('',(#6780));
#1765=EDGE_LOOP('',(#6781));
#1766=EDGE_LOOP('',(#6782));
#1767=EDGE_LOOP('',(#6783));
#1768=EDGE_LOOP('',(#6784));
#1769=EDGE_LOOP('',(#6785,#6786,#6787,#6788));
#1770=EDGE_LOOP('',(#6789,#6790,#6791,#6792));
#1771=EDGE_LOOP('',(#6793,#6794,#6795,#6796));
#1772=EDGE_LOOP('',(#6797,#6798,#6799,#6800));
#1773=EDGE_LOOP('',(#6801,#6802,#6803,#6804));
#1774=EDGE_LOOP('',(#6805,#6806,#6807,#6808));
#1775=EDGE_LOOP('',(#6809,#6810,#6811,#6812));
#1776=EDGE_LOOP('',(#6813,#6814,#6815,#6816));
#1777=EDGE_LOOP('',(#6817,#6818,#6819,#6820));
#1778=EDGE_LOOP('',(#6821,#6822,#6823,#6824));
#1779=EDGE_LOOP('',(#6825,#6826,#6827,#6828));
#1780=EDGE_LOOP('',(#6829,#6830,#6831,#6832));
#1781=EDGE_LOOP('',(#6833,#6834,#6835,#6836));
#1782=EDGE_LOOP('',(#6837,#6838,#6839,#6840));
#1783=EDGE_LOOP('',(#6841,#6842,#6843,#6844));
#1784=EDGE_LOOP('',(#6845));
#1785=EDGE_LOOP('',(#6846,#6847,#6848,#6849));
#1786=EDGE_LOOP('',(#6850,#6851,#6852,#6853));
#1787=EDGE_LOOP('',(#6854,#6855,#6856,#6857));
#1788=EDGE_LOOP('',(#6858,#6859,#6860,#6861));
#1789=EDGE_LOOP('',(#6862,#6863,#6864,#6865));
#1790=EDGE_LOOP('',(#6866,#6867,#6868,#6869));
#1791=EDGE_LOOP('',(#6870));
#1792=EDGE_LOOP('',(#6871));
#1793=EDGE_LOOP('',(#6872,#6873,#6874,#6875));
#1794=EDGE_LOOP('',(#6876));
#1795=EDGE_LOOP('',(#6877));
#1796=EDGE_LOOP('',(#6878));
#1797=EDGE_LOOP('',(#6879));
#1798=EDGE_LOOP('',(#6880,#6881,#6882,#6883));
#1799=EDGE_LOOP('',(#6884));
#1800=EDGE_LOOP('',(#6885));
#1801=EDGE_LOOP('',(#6886));
#1802=EDGE_LOOP('',(#6887));
#1803=EDGE_LOOP('',(#6888,#6889,#6890,#6891));
#1804=EDGE_LOOP('',(#6892));
#1805=EDGE_LOOP('',(#6893));
#1806=EDGE_LOOP('',(#6894));
#1807=EDGE_LOOP('',(#6895));
#1808=EDGE_LOOP('',(#6896,#6897,#6898,#6899));
#1809=EDGE_LOOP('',(#6900));
#1810=EDGE_LOOP('',(#6901));
#1811=EDGE_LOOP('',(#6902));
#1812=EDGE_LOOP('',(#6903));
#1813=EDGE_LOOP('',(#6904,#6905,#6906,#6907));
#1814=EDGE_LOOP('',(#6908));
#1815=EDGE_LOOP('',(#6909));
#1816=EDGE_LOOP('',(#6910,#6911,#6912,#6913));
#2331=LINE('',#16783,#2909);
#2332=LINE('',#16790,#2910);
#2333=LINE('',#16798,#2911);
#2334=LINE('',#16802,#2912);
#2335=LINE('',#16808,#2913);
#2336=LINE('',#16813,#2914);
#2337=LINE('',#16817,#2915);
#2338=LINE('',#17808,#2916);
#2339=LINE('',#17887,#2917);
#2340=LINE('',#17889,#2918);
#2341=LINE('',#17891,#2919);
#2342=LINE('',#17893,#2920);
#2343=LINE('',#17895,#2921);
#2344=LINE('',#17897,#2922);
#2345=LINE('',#17899,#2923);
#2346=LINE('',#17901,#2924);
#2347=LINE('',#17904,#2925);
#2348=LINE('',#17907,#2926);
#2349=LINE('',#17909,#2927);
#2350=LINE('',#17911,#2928);
#2351=LINE('',#17913,#2929);
#2352=LINE('',#17915,#2930);
#2353=LINE('',#17917,#2931);
#2354=LINE('',#17923,#2932);
#2355=LINE('',#17929,#2933);
#2356=LINE('',#17935,#2934);
#2357=LINE('',#17941,#2935);
#2358=LINE('',#17944,#2936);
#2359=LINE('',#17951,#2937);
#2360=LINE('',#17959,#2938);
#2361=LINE('',#17967,#2939);
#2362=LINE('',#17975,#2940);
#2363=LINE('',#17985,#2941);
#2364=LINE('',#17988,#2942);
#2909=VECTOR('',#11461,0.0041);
#2910=VECTOR('',#11470,0.004);
#2911=VECTOR('',#11479,0.0079);
#2912=VECTOR('',#11484,0.008);
#2913=VECTOR('',#11493,0.0079);
#2914=VECTOR('',#11498,0.00305);
#2915=VECTOR('',#11503,0.0021);
#2916=VECTOR('',#11512,0.0023);
#2917=VECTOR('',#11607,0.01115);
#2918=VECTOR('',#11610,0.01115);
#2919=VECTOR('',#11613,0.01115);
#2920=VECTOR('',#11616,0.01115);
#2921=VECTOR('',#11619,0.01115);
#2922=VECTOR('',#11622,0.01115);
#2923=VECTOR('',#11625,0.01115);
#2924=VECTOR('',#11628,0.01115);
#2925=VECTOR('',#11631,0.0045);
#2926=VECTOR('',#11636,0.0045);
#2927=VECTOR('',#11639,0.0045);
#2928=VECTOR('',#11642,0.0045);
#2929=VECTOR('',#11645,0.0045);
#2930=VECTOR('',#11648,0.0045);
#2931=VECTOR('',#11651,0.0045);
#2932=VECTOR('',#11658,0.0045);
#2933=VECTOR('',#11665,0.0045);
#2934=VECTOR('',#11672,0.0045);
#2935=VECTOR('',#11679,0.0045);
#2936=VECTOR('',#11684,0.0045);
#2937=VECTOR('',#11693,0.01115);
#2938=VECTOR('',#11704,0.01115);
#2939=VECTOR('',#11715,0.01115);
#2940=VECTOR('',#11726,0.008);
#2941=VECTOR('',#11739,0.008);
#2942=VECTOR('',#11744,0.006);
#3461=CIRCLE('',#10267,0.00307350000001);
#3462=CIRCLE('',#10268,0.00307350000001);
#3463=CIRCLE('',#10270,0.00251750000001);
#3464=CIRCLE('',#10271,0.00251750000001);
#3465=CIRCLE('',#10272,0.00251750000001);
#3466=CIRCLE('',#10274,0.00400000000001);
#3467=CIRCLE('',#10275,0.00420000000001);
#3468=CIRCLE('',#10277,0.00780000000001);
#3469=CIRCLE('',#10279,0.00400000000001);
#3470=CIRCLE('',#10280,0.00400000000001);
#3471=CIRCLE('',#10282,0.00800000000001);
#3472=CIRCLE('',#10283,0.00780000000001);
#3473=CIRCLE('',#10285,0.00800000000001);
#3474=CIRCLE('',#10287,0.00600000000001);
#3475=CIRCLE('',#10290,0.00210000000001);
#3476=CIRCLE('',#10291,0.00210000000001);
#3477=CIRCLE('',#10293,0.00210000000001);
#3478=CIRCLE('',#10294,0.00210000000001);
#3479=CIRCLE('',#10298,0.01115000000001);
#3480=CIRCLE('',#10299,0.0060198255992182);
#3481=CIRCLE('',#10301,0.01115000000001);
#3482=CIRCLE('',#10302,0.00588880615101059);
#3483=CIRCLE('',#10304,0.01115000000001);
#3484=CIRCLE('',#10305,0.00594121393029363);
#3485=CIRCLE('',#10307,0.01115000000001);
#3486=CIRCLE('',#10308,0.00575778670280299);
#3487=CIRCLE('',#10310,0.01115000000001);
#3488=CIRCLE('',#10311,0.00581019448208603);
#3489=CIRCLE('',#10313,0.01115000000001);
#3490=CIRCLE('',#10314,0.00562676725459539);
#3491=CIRCLE('',#10316,0.01115000000001);
#3492=CIRCLE('',#10317,0.00567917503387843);
#3493=CIRCLE('',#10319,0.01115000000001);
#3494=CIRCLE('',#10320,0.00549574780638778);
#3495=CIRCLE('',#10322,0.01115000000001);
#3496=CIRCLE('',#10323,0.00554815558567082);
#3497=CIRCLE('',#10325,0.01115000000001);
#3498=CIRCLE('',#10326,0.00536472835818018);
#3499=CIRCLE('',#10328,0.01115000000001);
#3500=CIRCLE('',#10329,0.00541713613746322);
#3501=CIRCLE('',#10331,0.01115000000001);
#3502=CIRCLE('',#10332,0.00523370890997258);
#3503=CIRCLE('',#10334,0.01115000000001);
#3504=CIRCLE('',#10335,0.00528611668925562);
#3505=CIRCLE('',#10337,0.01115000000001);
#3506=CIRCLE('',#10338,0.00515509724104802);
#3507=CIRCLE('',#10340,0.01115000000001);
#3508=CIRCLE('',#10341,0.00510268946176497);
#3509=CIRCLE('',#10343,0.01115000000001);
#3510=CIRCLE('',#10352,0.00502407779284041);
#3511=CIRCLE('',#10361,0.00470963111714216);
#3512=CIRCLE('',#10362,0.0046310194482176);
#3513=CIRCLE('',#10364,0.00457861166893456);
#3514=CIRCLE('',#10365,0.00450000000001);
#3515=CIRCLE('',#10367,0.00484065056534977);
#3516=CIRCLE('',#10368,0.00476203889642521);
#3517=CIRCLE('',#10370,0.00497167001355737);
#3518=CIRCLE('',#10371,0.00489305834463281);
#3519=CIRCLE('',#10374,0.01115000000001);
#3520=CIRCLE('',#10376,0.01115000000001);
#3521=CIRCLE('',#10379,0.01115000000001);
#3522=CIRCLE('',#10381,0.01115000000001);
#3523=CIRCLE('',#10384,0.01115000000001);
#3524=CIRCLE('',#10386,0.01115000000001);
#3525=CIRCLE('',#10389,0.00800000000001);
#3526=CIRCLE('',#10391,0.00800000000001);
#3527=CIRCLE('',#10394,0.00800000000001);
#3528=CIRCLE('',#10395,0.00600000000001);
#3529=CIRCLE('',#10397,0.00800000000001);
#3882=VERTEX_POINT('',#13866);
#3883=VERTEX_POINT('',#13867);
#3884=VERTEX_POINT('',#13935);
#3885=VERTEX_POINT('',#13985);
#3886=VERTEX_POINT('',#14035);
#3887=VERTEX_POINT('',#14085);
#3888=VERTEX_POINT('',#14135);
#3889=VERTEX_POINT('',#14185);
#3890=VERTEX_POINT('',#14235);
#3891=VERTEX_POINT('',#14285);
#3892=VERTEX_POINT('',#14335);
#3893=VERTEX_POINT('',#14385);
#3894=VERTEX_POINT('',#14393);
#3895=VERTEX_POINT('',#14395);
#3896=VERTEX_POINT('',#14433);
#3897=VERTEX_POINT('',#14483);
#3898=VERTEX_POINT('',#14533);
#3899=VERTEX_POINT('',#14583);
#3900=VERTEX_POINT('',#14633);
#3901=VERTEX_POINT('',#14710);
#3902=VERTEX_POINT('',#14760);
#3903=VERTEX_POINT('',#14810);
#3904=VERTEX_POINT('',#14860);
#3905=VERTEX_POINT('',#14910);
#3906=VERTEX_POINT('',#14960);
#3907=VERTEX_POINT('',#15010);
#3908=VERTEX_POINT('',#15084);
#3909=VERTEX_POINT('',#15134);
#3910=VERTEX_POINT('',#15154);
#3911=VERTEX_POINT('',#15156);
#3912=VERTEX_POINT('',#15191);
#3913=VERTEX_POINT('',#15241);
#3914=VERTEX_POINT('',#15341);
#3915=VERTEX_POINT('',#15342);
#3916=VERTEX_POINT('',#15419);
#3917=VERTEX_POINT('',#15469);
#3918=VERTEX_POINT('',#15519);
#3919=VERTEX_POINT('',#15554);
#3920=VERTEX_POINT('',#15604);
#3921=VERTEX_POINT('',#15654);
#3922=VERTEX_POINT('',#15704);
#3923=VERTEX_POINT('',#15781);
#3924=VERTEX_POINT('',#15831);
#3925=VERTEX_POINT('',#15833);
#3926=VERTEX_POINT('',#15841);
#3927=VERTEX_POINT('',#15891);
#3928=VERTEX_POINT('',#15941);
#3929=VERTEX_POINT('',#15994);
#3930=VERTEX_POINT('',#16044);
#3931=VERTEX_POINT('',#16094);
#3932=VERTEX_POINT('',#16144);
#3933=VERTEX_POINT('',#16194);
#3934=VERTEX_POINT('',#16244);
#3935=VERTEX_POINT('',#16294);
#3936=VERTEX_POINT('',#16341);
#3937=VERTEX_POINT('',#16391);
#3938=VERTEX_POINT('',#16441);
#3939=VERTEX_POINT('',#16491);
#3940=VERTEX_POINT('',#16541);
#3941=VERTEX_POINT('',#16543);
#3942=VERTEX_POINT('',#16593);
#3943=VERTEX_POINT('',#16628);
#3944=VERTEX_POINT('',#16678);
#3945=VERTEX_POINT('',#16777);
#3946=VERTEX_POINT('',#16780);
#3947=VERTEX_POINT('',#16782);
#3948=VERTEX_POINT('',#16786);
#3949=VERTEX_POINT('',#16789);
#3950=VERTEX_POINT('',#16791);
#3951=VERTEX_POINT('',#16795);
#3952=VERTEX_POINT('',#16797);
#3953=VERTEX_POINT('',#16801);
#3954=VERTEX_POINT('',#16805);
#3955=VERTEX_POINT('',#16810);
#3956=VERTEX_POINT('',#16811);
#3957=VERTEX_POINT('',#16816);
#3958=VERTEX_POINT('',#16818);
#3959=VERTEX_POINT('',#17810);
#3960=VERTEX_POINT('',#17812);
#3961=VERTEX_POINT('',#17815);
#3962=VERTEX_POINT('',#17817);
#3963=VERTEX_POINT('',#17820);
#3964=VERTEX_POINT('',#17822);
#3965=VERTEX_POINT('',#17825);
#3966=VERTEX_POINT('',#17827);
#3967=VERTEX_POINT('',#17830);
#3968=VERTEX_POINT('',#17832);
#3969=VERTEX_POINT('',#17835);
#3970=VERTEX_POINT('',#17837);
#3971=VERTEX_POINT('',#17840);
#3972=VERTEX_POINT('',#17842);
#3973=VERTEX_POINT('',#17845);
#3974=VERTEX_POINT('',#17847);
#3975=VERTEX_POINT('',#17850);
#3976=VERTEX_POINT('',#17852);
#3977=VERTEX_POINT('',#17855);
#3978=VERTEX_POINT('',#17857);
#3979=VERTEX_POINT('',#17860);
#3980=VERTEX_POINT('',#17862);
#3981=VERTEX_POINT('',#17865);
#3982=VERTEX_POINT('',#17867);
#3983=VERTEX_POINT('',#17870);
#3984=VERTEX_POINT('',#17872);
#3985=VERTEX_POINT('',#17875);
#3986=VERTEX_POINT('',#17877);
#3987=VERTEX_POINT('',#17880);
#3988=VERTEX_POINT('',#17882);
#3989=VERTEX_POINT('',#17885);
#3990=VERTEX_POINT('',#17903);
#3991=VERTEX_POINT('',#17920);
#3992=VERTEX_POINT('',#17922);
#3993=VERTEX_POINT('',#17926);
#3994=VERTEX_POINT('',#17928);
#3995=VERTEX_POINT('',#17932);
#3996=VERTEX_POINT('',#17934);
#3997=VERTEX_POINT('',#17938);
#3998=VERTEX_POINT('',#17940);
#3999=VERTEX_POINT('',#17946);
#4000=VERTEX_POINT('',#17949);
#4001=VERTEX_POINT('',#17954);
#4002=VERTEX_POINT('',#17957);
#4003=VERTEX_POINT('',#17962);
#4004=VERTEX_POINT('',#17965);
#4005=VERTEX_POINT('',#17970);
#4006=VERTEX_POINT('',#17973);
#4007=VERTEX_POINT('',#17978);
#4008=VERTEX_POINT('',#17980);
#4009=VERTEX_POINT('',#17983);
#4944=EDGE_CURVE('',#3882,#3883,#141,.T.);
#4945=EDGE_CURVE('',#3883,#3884,#142,.T.);
#4946=EDGE_CURVE('',#3884,#3885,#143,.T.);
#4947=EDGE_CURVE('',#3885,#3886,#144,.T.);
#4948=EDGE_CURVE('',#3886,#3887,#145,.T.);
#4949=EDGE_CURVE('',#3887,#3888,#146,.T.);
#4950=EDGE_CURVE('',#3888,#3889,#147,.T.);
#4951=EDGE_CURVE('',#3889,#3890,#148,.T.);
#4952=EDGE_CURVE('',#3890,#3891,#149,.T.);
#4953=EDGE_CURVE('',#3891,#3892,#150,.T.);
#4954=EDGE_CURVE('',#3892,#3893,#151,.T.);
#4955=EDGE_CURVE('',#3894,#3893,#3461,.T.);
#4956=EDGE_CURVE('',#3895,#3894,#152,.F.);
#4957=EDGE_CURVE('',#3896,#3895,#153,.F.);
#4958=EDGE_CURVE('',#3897,#3896,#154,.F.);
#4959=EDGE_CURVE('',#3898,#3897,#155,.F.);
#4960=EDGE_CURVE('',#3899,#3898,#156,.F.);
#4961=EDGE_CURVE('',#3900,#3899,#157,.F.);
#4962=EDGE_CURVE('',#3901,#3900,#158,.F.);
#4963=EDGE_CURVE('',#3902,#3901,#159,.F.);
#4964=EDGE_CURVE('',#3903,#3902,#160,.F.);
#4965=EDGE_CURVE('',#3904,#3903,#161,.F.);
#4966=EDGE_CURVE('',#3905,#3904,#162,.F.);
#4967=EDGE_CURVE('',#3906,#3905,#163,.F.);
#4968=EDGE_CURVE('',#3907,#3906,#164,.F.);
#4969=EDGE_CURVE('',#3908,#3907,#165,.F.);
#4970=EDGE_CURVE('',#3909,#3908,#166,.F.);
#4971=EDGE_CURVE('',#3910,#3909,#3462,.T.);
#4972=EDGE_CURVE('',#3910,#3911,#167,.T.);
#4973=EDGE_CURVE('',#3911,#3912,#168,.T.);
#4974=EDGE_CURVE('',#3912,#3913,#169,.T.);
#4975=EDGE_CURVE('',#3913,#3882,#170,.T.);
#4976=EDGE_CURVE('',#3914,#3915,#171,.T.);
#4977=EDGE_CURVE('',#3915,#3916,#172,.T.);
#4978=EDGE_CURVE('',#3916,#3917,#173,.T.);
#4979=EDGE_CURVE('',#3917,#3918,#174,.T.);
#4980=EDGE_CURVE('',#3918,#3919,#175,.T.);
#4981=EDGE_CURVE('',#3919,#3920,#176,.T.);
#4982=EDGE_CURVE('',#3920,#3921,#177,.T.);
#4983=EDGE_CURVE('',#3921,#3922,#178,.T.);
#4984=EDGE_CURVE('',#3922,#3923,#179,.T.);
#4985=EDGE_CURVE('',#3923,#3924,#3463,.T.);
#4986=EDGE_CURVE('',#3924,#3925,#180,.T.);
#4987=EDGE_CURVE('',#3925,#3926,#181,.T.);
#4988=EDGE_CURVE('',#3926,#3927,#182,.T.);
#4989=EDGE_CURVE('',#3927,#3928,#183,.T.);
#4990=EDGE_CURVE('',#3928,#3929,#184,.T.);
#4991=EDGE_CURVE('',#3929,#3930,#185,.T.);
#4992=EDGE_CURVE('',#3930,#3931,#186,.T.);
#4993=EDGE_CURVE('',#3931,#3932,#187,.T.);
#4994=EDGE_CURVE('',#3932,#3933,#188,.T.);
#4995=EDGE_CURVE('',#3933,#3934,#189,.T.);
#4996=EDGE_CURVE('',#3934,#3935,#190,.T.);
#4997=EDGE_CURVE('',#3935,#3936,#191,.T.);
#4998=EDGE_CURVE('',#3936,#3937,#192,.T.);
#4999=EDGE_CURVE('',#3937,#3938,#193,.T.);
#5000=EDGE_CURVE('',#3938,#3939,#194,.T.);
#5001=EDGE_CURVE('',#3940,#3939,#3464,.T.);
#5002=EDGE_CURVE('',#3940,#3941,#195,.T.);
#5003=EDGE_CURVE('',#3941,#3942,#196,.T.);
#5004=EDGE_CURVE('',#3942,#3943,#197,.T.);
#5005=EDGE_CURVE('',#3943,#3944,#198,.T.);
#5006=EDGE_CURVE('',#3944,#3914,#199,.T.);
#5007=EDGE_CURVE('',#3945,#3945,#3465,.T.);
#5008=EDGE_CURVE('',#3946,#3946,#3466,.T.);
#5009=EDGE_CURVE('',#3946,#3947,#2331,.T.);
#5010=EDGE_CURVE('',#3947,#3947,#3467,.T.);
#5011=EDGE_CURVE('',#3948,#3948,#3468,.T.);
#5012=EDGE_CURVE('',#3946,#3949,#2332,.T.);
#5013=EDGE_CURVE('',#3949,#3950,#3469,.T.);
#5014=EDGE_CURVE('',#3950,#3949,#3470,.T.);
#5015=EDGE_CURVE('',#3951,#3951,#3471,.T.);
#5016=EDGE_CURVE('',#3951,#3952,#2333,.T.);
#5017=EDGE_CURVE('',#3952,#3952,#3472,.T.);
#5018=EDGE_CURVE('',#3951,#3953,#2334,.T.);
#5019=EDGE_CURVE('',#3953,#3953,#3473,.T.);
#5020=EDGE_CURVE('',#3954,#3954,#3474,.T.);
#5021=EDGE_CURVE('',#3953,#3948,#2335,.T.);
#5022=EDGE_CURVE('',#3955,#3956,#3475,.T.);
#5023=EDGE_CURVE('',#3956,#3950,#2336,.T.);
#5024=EDGE_CURVE('',#3956,#3955,#3476,.T.);
#5025=EDGE_CURVE('',#3955,#3957,#2337,.T.);
#5026=EDGE_CURVE('',#3958,#3957,#3477,.T.);
#5027=EDGE_CURVE('',#3957,#3958,#3478,.T.);
#5028=EDGE_CURVE('',#3923,#3894,#200,.T.);
#5029=EDGE_CURVE('',#3893,#3924,#201,.T.);
#5030=EDGE_CURVE('',#3939,#3910,#202,.T.);
#5031=EDGE_CURVE('',#3909,#3940,#203,.T.);
#5032=EDGE_CURVE('',#3958,#3945,#2338,.T.);
#5033=EDGE_CURVE('',#3959,#3959,#3479,.T.);
#5034=EDGE_CURVE('',#3960,#3960,#3480,.T.);
#5035=EDGE_CURVE('',#3961,#3961,#3481,.T.);
#5036=EDGE_CURVE('',#3962,#3962,#3482,.T.);
#5037=EDGE_CURVE('',#3963,#3963,#3483,.T.);
#5038=EDGE_CURVE('',#3964,#3964,#3484,.T.);
#5039=EDGE_CURVE('',#3965,#3965,#3485,.T.);
#5040=EDGE_CURVE('',#3966,#3966,#3486,.T.);
#5041=EDGE_CURVE('',#3967,#3967,#3487,.T.);
#5042=EDGE_CURVE('',#3968,#3968,#3488,.T.);
#5043=EDGE_CURVE('',#3969,#3969,#3489,.T.);
#5044=EDGE_CURVE('',#3970,#3970,#3490,.T.);
#5045=EDGE_CURVE('',#3971,#3971,#3491,.T.);
#5046=EDGE_CURVE('',#3972,#3972,#3492,.T.);
#5047=EDGE_CURVE('',#3973,#3973,#3493,.T.);
#5048=EDGE_CURVE('',#3974,#3974,#3494,.T.);
#5049=EDGE_CURVE('',#3975,#3975,#3495,.T.);
#5050=EDGE_CURVE('',#3976,#3976,#3496,.T.);
#5051=EDGE_CURVE('',#3977,#3977,#3497,.T.);
#5052=EDGE_CURVE('',#3978,#3978,#3498,.T.);
#5053=EDGE_CURVE('',#3979,#3979,#3499,.T.);
#5054=EDGE_CURVE('',#3980,#3980,#3500,.T.);
#5055=EDGE_CURVE('',#3981,#3981,#3501,.T.);
#5056=EDGE_CURVE('',#3982,#3982,#3502,.T.);
#5057=EDGE_CURVE('',#3983,#3983,#3503,.T.);
#5058=EDGE_CURVE('',#3984,#3984,#3504,.T.);
#5059=EDGE_CURVE('',#3985,#3985,#3505,.T.);
#5060=EDGE_CURVE('',#3986,#3986,#3506,.T.);
#5061=EDGE_CURVE('',#3987,#3987,#3507,.T.);
#5062=EDGE_CURVE('',#3988,#3988,#3508,.T.);
#5063=EDGE_CURVE('',#3989,#3989,#3509,.T.);
#5064=EDGE_CURVE('',#3989,#3959,#2339,.T.);
#5065=EDGE_CURVE('',#3963,#3961,#2340,.T.);
#5066=EDGE_CURVE('',#3967,#3965,#2341,.T.);
#5067=EDGE_CURVE('',#3971,#3969,#2342,.T.);
#5068=EDGE_CURVE('',#3975,#3973,#2343,.T.);
#5069=EDGE_CURVE('',#3979,#3977,#2344,.T.);
#5070=EDGE_CURVE('',#3983,#3981,#2345,.T.);
#5071=EDGE_CURVE('',#3985,#3987,#2346,.T.);
#5072=EDGE_CURVE('',#3988,#3990,#2347,.T.);
#5073=EDGE_CURVE('',#3990,#3990,#3510,.T.);
#5074=EDGE_CURVE('',#3978,#3984,#2348,.T.);
#5075=EDGE_CURVE('',#3974,#3980,#2349,.T.);
#5076=EDGE_CURVE('',#3970,#3976,#2350,.T.);
#5077=EDGE_CURVE('',#3966,#3972,#2351,.T.);
#5078=EDGE_CURVE('',#3962,#3968,#2352,.T.);
#5079=EDGE_CURVE('',#3960,#3964,#2353,.T.);
#5080=EDGE_CURVE('',#3991,#3991,#3511,.T.);
#5081=EDGE_CURVE('',#3991,#3992,#2354,.T.);
#5082=EDGE_CURVE('',#3992,#3992,#3512,.T.);
#5083=EDGE_CURVE('',#3993,#3993,#3513,.T.);
#5084=EDGE_CURVE('',#3993,#3994,#2355,.T.);
#5085=EDGE_CURVE('',#3994,#3994,#3514,.T.);
#5086=EDGE_CURVE('',#3995,#3995,#3515,.T.);
#5087=EDGE_CURVE('',#3995,#3996,#2356,.T.);
#5088=EDGE_CURVE('',#3996,#3996,#3516,.T.);
#5089=EDGE_CURVE('',#3997,#3997,#3517,.T.);
#5090=EDGE_CURVE('',#3997,#3998,#2357,.T.);
#5091=EDGE_CURVE('',#3998,#3998,#3518,.T.);
#5092=EDGE_CURVE('',#3982,#3986,#2358,.T.);
#5093=EDGE_CURVE('',#3999,#3999,#3519,.T.);
#5094=EDGE_CURVE('',#4000,#4000,#3520,.T.);
#5095=EDGE_CURVE('',#4000,#3999,#2359,.T.);
#5096=EDGE_CURVE('',#4001,#4001,#3521,.T.);
#5097=EDGE_CURVE('',#4002,#4002,#3522,.T.);
#5098=EDGE_CURVE('',#4002,#4001,#2360,.T.);
#5099=EDGE_CURVE('',#4003,#4003,#3523,.T.);
#5100=EDGE_CURVE('',#4004,#4004,#3524,.T.);
#5101=EDGE_CURVE('',#4004,#4003,#2361,.T.);
#5102=EDGE_CURVE('',#4005,#4005,#3525,.T.);
#5103=EDGE_CURVE('',#4006,#4006,#3526,.T.);
#5104=EDGE_CURVE('',#4006,#4005,#2362,.T.);
#5105=EDGE_CURVE('',#4007,#4007,#3527,.T.);
#5106=EDGE_CURVE('',#4008,#4008,#3528,.T.);
#5107=EDGE_CURVE('',#4009,#4009,#3529,.T.);
#5108=EDGE_CURVE('',#4009,#4007,#2363,.T.);
#5109=EDGE_CURVE('',#4008,#3954,#2364,.T.);
#6582=ORIENTED_EDGE('',*,*,#4944,.T.);
#6583=ORIENTED_EDGE('',*,*,#4945,.T.);
#6584=ORIENTED_EDGE('',*,*,#4946,.T.);
#6585=ORIENTED_EDGE('',*,*,#4947,.T.);
#6586=ORIENTED_EDGE('',*,*,#4948,.T.);
#6587=ORIENTED_EDGE('',*,*,#4949,.T.);
#6588=ORIENTED_EDGE('',*,*,#4950,.T.);
#6589=ORIENTED_EDGE('',*,*,#4951,.T.);
#6590=ORIENTED_EDGE('',*,*,#4952,.T.);
#6591=ORIENTED_EDGE('',*,*,#4953,.T.);
#6592=ORIENTED_EDGE('',*,*,#4954,.T.);
#6593=ORIENTED_EDGE('',*,*,#4955,.F.);
#6594=ORIENTED_EDGE('',*,*,#4956,.F.);
#6595=ORIENTED_EDGE('',*,*,#4957,.F.);
#6596=ORIENTED_EDGE('',*,*,#4958,.F.);
#6597=ORIENTED_EDGE('',*,*,#4959,.F.);
#6598=ORIENTED_EDGE('',*,*,#4960,.F.);
#6599=ORIENTED_EDGE('',*,*,#4961,.F.);
#6600=ORIENTED_EDGE('',*,*,#4962,.F.);
#6601=ORIENTED_EDGE('',*,*,#4963,.F.);
#6602=ORIENTED_EDGE('',*,*,#4964,.F.);
#6603=ORIENTED_EDGE('',*,*,#4965,.F.);
#6604=ORIENTED_EDGE('',*,*,#4966,.F.);
#6605=ORIENTED_EDGE('',*,*,#4967,.F.);
#6606=ORIENTED_EDGE('',*,*,#4968,.F.);
#6607=ORIENTED_EDGE('',*,*,#4969,.F.);
#6608=ORIENTED_EDGE('',*,*,#4970,.F.);
#6609=ORIENTED_EDGE('',*,*,#4971,.F.);
#6610=ORIENTED_EDGE('',*,*,#4972,.T.);
#6611=ORIENTED_EDGE('',*,*,#4973,.T.);
#6612=ORIENTED_EDGE('',*,*,#4974,.T.);
#6613=ORIENTED_EDGE('',*,*,#4975,.T.);
#6614=ORIENTED_EDGE('',*,*,#4976,.T.);
#6615=ORIENTED_EDGE('',*,*,#4977,.T.);
#6616=ORIENTED_EDGE('',*,*,#4978,.T.);
#6617=ORIENTED_EDGE('',*,*,#4979,.T.);
#6618=ORIENTED_EDGE('',*,*,#4980,.T.);
#6619=ORIENTED_EDGE('',*,*,#4981,.T.);
#6620=ORIENTED_EDGE('',*,*,#4982,.T.);
#6621=ORIENTED_EDGE('',*,*,#4983,.T.);
#6622=ORIENTED_EDGE('',*,*,#4984,.T.);
#6623=ORIENTED_EDGE('',*,*,#4985,.T.);
#6624=ORIENTED_EDGE('',*,*,#4986,.T.);
#6625=ORIENTED_EDGE('',*,*,#4987,.T.);
#6626=ORIENTED_EDGE('',*,*,#4988,.T.);
#6627=ORIENTED_EDGE('',*,*,#4989,.T.);
#6628=ORIENTED_EDGE('',*,*,#4990,.T.);
#6629=ORIENTED_EDGE('',*,*,#4991,.T.);
#6630=ORIENTED_EDGE('',*,*,#4992,.T.);
#6631=ORIENTED_EDGE('',*,*,#4993,.T.);
#6632=ORIENTED_EDGE('',*,*,#4994,.T.);
#6633=ORIENTED_EDGE('',*,*,#4995,.T.);
#6634=ORIENTED_EDGE('',*,*,#4996,.T.);
#6635=ORIENTED_EDGE('',*,*,#4997,.T.);
#6636=ORIENTED_EDGE('',*,*,#4998,.T.);
#6637=ORIENTED_EDGE('',*,*,#4999,.T.);
#6638=ORIENTED_EDGE('',*,*,#5000,.T.);
#6639=ORIENTED_EDGE('',*,*,#5001,.F.);
#6640=ORIENTED_EDGE('',*,*,#5002,.T.);
#6641=ORIENTED_EDGE('',*,*,#5003,.T.);
#6642=ORIENTED_EDGE('',*,*,#5004,.T.);
#6643=ORIENTED_EDGE('',*,*,#5005,.T.);
#6644=ORIENTED_EDGE('',*,*,#5006,.T.);
#6645=ORIENTED_EDGE('',*,*,#5007,.T.);
#6646=ORIENTED_EDGE('',*,*,#5008,.T.);
#6647=ORIENTED_EDGE('',*,*,#5009,.T.);
#6648=ORIENTED_EDGE('',*,*,#5010,.T.);
#6649=ORIENTED_EDGE('',*,*,#5009,.F.);
#6650=ORIENTED_EDGE('',*,*,#5011,.F.);
#6651=ORIENTED_EDGE('',*,*,#5010,.F.);
#6652=ORIENTED_EDGE('',*,*,#5008,.F.);
#6653=ORIENTED_EDGE('',*,*,#5012,.T.);
#6654=ORIENTED_EDGE('',*,*,#5013,.T.);
#6655=ORIENTED_EDGE('',*,*,#5014,.T.);
#6656=ORIENTED_EDGE('',*,*,#5012,.F.);
#6657=ORIENTED_EDGE('',*,*,#5015,.T.);
#6658=ORIENTED_EDGE('',*,*,#5016,.T.);
#6659=ORIENTED_EDGE('',*,*,#5017,.T.);
#6660=ORIENTED_EDGE('',*,*,#5016,.F.);
#6661=ORIENTED_EDGE('',*,*,#5015,.F.);
#6662=ORIENTED_EDGE('',*,*,#5018,.T.);
#6663=ORIENTED_EDGE('',*,*,#5019,.F.);
#6664=ORIENTED_EDGE('',*,*,#5018,.F.);
#6665=ORIENTED_EDGE('',*,*,#5017,.F.);
#6666=ORIENTED_EDGE('',*,*,#5020,.T.);
#6667=ORIENTED_EDGE('',*,*,#5019,.T.);
#6668=ORIENTED_EDGE('',*,*,#5021,.T.);
#6669=ORIENTED_EDGE('',*,*,#5011,.T.);
#6670=ORIENTED_EDGE('',*,*,#5021,.F.);
#6671=ORIENTED_EDGE('',*,*,#5022,.T.);
#6672=ORIENTED_EDGE('',*,*,#5023,.T.);
#6673=ORIENTED_EDGE('',*,*,#5013,.F.);
#6674=ORIENTED_EDGE('',*,*,#5014,.F.);
#6675=ORIENTED_EDGE('',*,*,#5023,.F.);
#6676=ORIENTED_EDGE('',*,*,#5024,.T.);
#6677=ORIENTED_EDGE('',*,*,#5022,.F.);
#6678=ORIENTED_EDGE('',*,*,#5025,.T.);
#6679=ORIENTED_EDGE('',*,*,#5026,.F.);
#6680=ORIENTED_EDGE('',*,*,#5027,.F.);
#6681=ORIENTED_EDGE('',*,*,#5025,.F.);
#6682=ORIENTED_EDGE('',*,*,#5024,.F.);
#6683=ORIENTED_EDGE('',*,*,#4985,.F.);
#6684=ORIENTED_EDGE('',*,*,#5028,.T.);
#6685=ORIENTED_EDGE('',*,*,#4955,.T.);
#6686=ORIENTED_EDGE('',*,*,#5029,.T.);
#6687=ORIENTED_EDGE('',*,*,#5029,.F.);
#6688=ORIENTED_EDGE('',*,*,#4954,.F.);
#6689=ORIENTED_EDGE('',*,*,#4953,.F.);
#6690=ORIENTED_EDGE('',*,*,#4952,.F.);
#6691=ORIENTED_EDGE('',*,*,#4951,.F.);
#6692=ORIENTED_EDGE('',*,*,#4950,.F.);
#6693=ORIENTED_EDGE('',*,*,#4949,.F.);
#6694=ORIENTED_EDGE('',*,*,#4948,.F.);
#6695=ORIENTED_EDGE('',*,*,#4947,.F.);
#6696=ORIENTED_EDGE('',*,*,#4946,.F.);
#6697=ORIENTED_EDGE('',*,*,#4945,.F.);
#6698=ORIENTED_EDGE('',*,*,#4944,.F.);
#6699=ORIENTED_EDGE('',*,*,#4975,.F.);
#6700=ORIENTED_EDGE('',*,*,#4974,.F.);
#6701=ORIENTED_EDGE('',*,*,#4973,.F.);
#6702=ORIENTED_EDGE('',*,*,#4972,.F.);
#6703=ORIENTED_EDGE('',*,*,#5030,.F.);
#6704=ORIENTED_EDGE('',*,*,#5000,.F.);
#6705=ORIENTED_EDGE('',*,*,#4999,.F.);
#6706=ORIENTED_EDGE('',*,*,#4998,.F.);
#6707=ORIENTED_EDGE('',*,*,#4997,.F.);
#6708=ORIENTED_EDGE('',*,*,#4996,.F.);
#6709=ORIENTED_EDGE('',*,*,#4995,.F.);
#6710=ORIENTED_EDGE('',*,*,#4994,.F.);
#6711=ORIENTED_EDGE('',*,*,#4993,.F.);
#6712=ORIENTED_EDGE('',*,*,#4992,.F.);
#6713=ORIENTED_EDGE('',*,*,#4991,.F.);
#6714=ORIENTED_EDGE('',*,*,#4990,.F.);
#6715=ORIENTED_EDGE('',*,*,#4989,.F.);
#6716=ORIENTED_EDGE('',*,*,#4988,.F.);
#6717=ORIENTED_EDGE('',*,*,#4987,.F.);
#6718=ORIENTED_EDGE('',*,*,#4986,.F.);
#6719=ORIENTED_EDGE('',*,*,#5028,.F.);
#6720=ORIENTED_EDGE('',*,*,#4984,.F.);
#6721=ORIENTED_EDGE('',*,*,#4983,.F.);
#6722=ORIENTED_EDGE('',*,*,#4982,.F.);
#6723=ORIENTED_EDGE('',*,*,#4981,.F.);
#6724=ORIENTED_EDGE('',*,*,#4980,.F.);
#6725=ORIENTED_EDGE('',*,*,#4979,.F.);
#6726=ORIENTED_EDGE('',*,*,#4978,.F.);
#6727=ORIENTED_EDGE('',*,*,#4977,.F.);
#6728=ORIENTED_EDGE('',*,*,#4976,.F.);
#6729=ORIENTED_EDGE('',*,*,#5006,.F.);
#6730=ORIENTED_EDGE('',*,*,#5005,.F.);
#6731=ORIENTED_EDGE('',*,*,#5004,.F.);
#6732=ORIENTED_EDGE('',*,*,#5003,.F.);
#6733=ORIENTED_EDGE('',*,*,#5002,.F.);
#6734=ORIENTED_EDGE('',*,*,#5031,.F.);
#6735=ORIENTED_EDGE('',*,*,#4970,.T.);
#6736=ORIENTED_EDGE('',*,*,#4969,.T.);
#6737=ORIENTED_EDGE('',*,*,#4968,.T.);
#6738=ORIENTED_EDGE('',*,*,#4967,.T.);
#6739=ORIENTED_EDGE('',*,*,#4966,.T.);
#6740=ORIENTED_EDGE('',*,*,#4965,.T.);
#6741=ORIENTED_EDGE('',*,*,#4964,.T.);
#6742=ORIENTED_EDGE('',*,*,#4963,.T.);
#6743=ORIENTED_EDGE('',*,*,#4962,.T.);
#6744=ORIENTED_EDGE('',*,*,#4961,.T.);
#6745=ORIENTED_EDGE('',*,*,#4960,.T.);
#6746=ORIENTED_EDGE('',*,*,#4959,.T.);
#6747=ORIENTED_EDGE('',*,*,#4958,.T.);
#6748=ORIENTED_EDGE('',*,*,#4957,.T.);
#6749=ORIENTED_EDGE('',*,*,#4956,.T.);
#6750=ORIENTED_EDGE('',*,*,#5026,.T.);
#6751=ORIENTED_EDGE('',*,*,#5027,.T.);
#6752=ORIENTED_EDGE('',*,*,#5032,.T.);
#6753=ORIENTED_EDGE('',*,*,#5007,.F.);
#6754=ORIENTED_EDGE('',*,*,#5032,.F.);
#6755=ORIENTED_EDGE('',*,*,#5033,.T.);
#6756=ORIENTED_EDGE('',*,*,#5034,.F.);
#6757=ORIENTED_EDGE('',*,*,#5035,.T.);
#6758=ORIENTED_EDGE('',*,*,#5036,.F.);
#6759=ORIENTED_EDGE('',*,*,#5037,.T.);
#6760=ORIENTED_EDGE('',*,*,#5038,.F.);
#6761=ORIENTED_EDGE('',*,*,#5039,.T.);
#6762=ORIENTED_EDGE('',*,*,#5040,.F.);
#6763=ORIENTED_EDGE('',*,*,#5041,.T.);
#6764=ORIENTED_EDGE('',*,*,#5042,.F.);
#6765=ORIENTED_EDGE('',*,*,#5043,.T.);
#6766=ORIENTED_EDGE('',*,*,#5044,.F.);
#6767=ORIENTED_EDGE('',*,*,#5045,.T.);
#6768=ORIENTED_EDGE('',*,*,#5046,.F.);
#6769=ORIENTED_EDGE('',*,*,#5047,.T.);
#6770=ORIENTED_EDGE('',*,*,#5048,.F.);
#6771=ORIENTED_EDGE('',*,*,#5049,.T.);
#6772=ORIENTED_EDGE('',*,*,#5050,.F.);
#6773=ORIENTED_EDGE('',*,*,#5051,.T.);
#6774=ORIENTED_EDGE('',*,*,#5052,.F.);
#6775=ORIENTED_EDGE('',*,*,#5053,.T.);
#6776=ORIENTED_EDGE('',*,*,#5054,.F.);
#6777=ORIENTED_EDGE('',*,*,#5055,.F.);
#6778=ORIENTED_EDGE('',*,*,#5056,.F.);
#6779=ORIENTED_EDGE('',*,*,#5057,.T.);
#6780=ORIENTED_EDGE('',*,*,#5058,.F.);
#6781=ORIENTED_EDGE('',*,*,#5059,.T.);
#6782=ORIENTED_EDGE('',*,*,#5060,.F.);
#6783=ORIENTED_EDGE('',*,*,#5061,.F.);
#6784=ORIENTED_EDGE('',*,*,#5062,.F.);
#6785=ORIENTED_EDGE('',*,*,#5063,.F.);
#6786=ORIENTED_EDGE('',*,*,#5064,.T.);
#6787=ORIENTED_EDGE('',*,*,#5033,.F.);
#6788=ORIENTED_EDGE('',*,*,#5064,.F.);
#6789=ORIENTED_EDGE('',*,*,#5037,.F.);
#6790=ORIENTED_EDGE('',*,*,#5065,.T.);
#6791=ORIENTED_EDGE('',*,*,#5035,.F.);
#6792=ORIENTED_EDGE('',*,*,#5065,.F.);
#6793=ORIENTED_EDGE('',*,*,#5041,.F.);
#6794=ORIENTED_EDGE('',*,*,#5066,.T.);
#6795=ORIENTED_EDGE('',*,*,#5039,.F.);
#6796=ORIENTED_EDGE('',*,*,#5066,.F.);
#6797=ORIENTED_EDGE('',*,*,#5045,.F.);
#6798=ORIENTED_EDGE('',*,*,#5067,.T.);
#6799=ORIENTED_EDGE('',*,*,#5043,.F.);
#6800=ORIENTED_EDGE('',*,*,#5067,.F.);
#6801=ORIENTED_EDGE('',*,*,#5049,.F.);
#6802=ORIENTED_EDGE('',*,*,#5068,.T.);
#6803=ORIENTED_EDGE('',*,*,#5047,.F.);
#6804=ORIENTED_EDGE('',*,*,#5068,.F.);
#6805=ORIENTED_EDGE('',*,*,#5053,.F.);
#6806=ORIENTED_EDGE('',*,*,#5069,.T.);
#6807=ORIENTED_EDGE('',*,*,#5051,.F.);
#6808=ORIENTED_EDGE('',*,*,#5069,.F.);
#6809=ORIENTED_EDGE('',*,*,#5057,.F.);
#6810=ORIENTED_EDGE('',*,*,#5070,.T.);
#6811=ORIENTED_EDGE('',*,*,#5055,.T.);
#6812=ORIENTED_EDGE('',*,*,#5070,.F.);
#6813=ORIENTED_EDGE('',*,*,#5059,.F.);
#6814=ORIENTED_EDGE('',*,*,#5071,.T.);
#6815=ORIENTED_EDGE('',*,*,#5061,.T.);
#6816=ORIENTED_EDGE('',*,*,#5071,.F.);
#6817=ORIENTED_EDGE('',*,*,#5062,.T.);
#6818=ORIENTED_EDGE('',*,*,#5072,.T.);
#6819=ORIENTED_EDGE('',*,*,#5073,.F.);
#6820=ORIENTED_EDGE('',*,*,#5072,.F.);
#6821=ORIENTED_EDGE('',*,*,#5052,.T.);
#6822=ORIENTED_EDGE('',*,*,#5074,.T.);
#6823=ORIENTED_EDGE('',*,*,#5058,.T.);
#6824=ORIENTED_EDGE('',*,*,#5074,.F.);
#6825=ORIENTED_EDGE('',*,*,#5048,.T.);
#6826=ORIENTED_EDGE('',*,*,#5075,.T.);
#6827=ORIENTED_EDGE('',*,*,#5054,.T.);
#6828=ORIENTED_EDGE('',*,*,#5075,.F.);
#6829=ORIENTED_EDGE('',*,*,#5044,.T.);
#6830=ORIENTED_EDGE('',*,*,#5076,.T.);
#6831=ORIENTED_EDGE('',*,*,#5050,.T.);
#6832=ORIENTED_EDGE('',*,*,#5076,.F.);
#6833=ORIENTED_EDGE('',*,*,#5040,.T.);
#6834=ORIENTED_EDGE('',*,*,#5077,.T.);
#6835=ORIENTED_EDGE('',*,*,#5046,.T.);
#6836=ORIENTED_EDGE('',*,*,#5077,.F.);
#6837=ORIENTED_EDGE('',*,*,#5036,.T.);
#6838=ORIENTED_EDGE('',*,*,#5078,.T.);
#6839=ORIENTED_EDGE('',*,*,#5042,.T.);
#6840=ORIENTED_EDGE('',*,*,#5078,.F.);
#6841=ORIENTED_EDGE('',*,*,#5034,.T.);
#6842=ORIENTED_EDGE('',*,*,#5079,.T.);
#6843=ORIENTED_EDGE('',*,*,#5038,.T.);
#6844=ORIENTED_EDGE('',*,*,#5079,.F.);
#6845=ORIENTED_EDGE('',*,*,#5063,.T.);
#6846=ORIENTED_EDGE('',*,*,#5031,.T.);
#6847=ORIENTED_EDGE('',*,*,#5001,.T.);
#6848=ORIENTED_EDGE('',*,*,#5030,.T.);
#6849=ORIENTED_EDGE('',*,*,#4971,.T.);
#6850=ORIENTED_EDGE('',*,*,#5080,.F.);
#6851=ORIENTED_EDGE('',*,*,#5081,.T.);
#6852=ORIENTED_EDGE('',*,*,#5082,.F.);
#6853=ORIENTED_EDGE('',*,*,#5081,.F.);
#6854=ORIENTED_EDGE('',*,*,#5083,.F.);
#6855=ORIENTED_EDGE('',*,*,#5084,.T.);
#6856=ORIENTED_EDGE('',*,*,#5085,.F.);
#6857=ORIENTED_EDGE('',*,*,#5084,.F.);
#6858=ORIENTED_EDGE('',*,*,#5086,.F.);
#6859=ORIENTED_EDGE('',*,*,#5087,.T.);
#6860=ORIENTED_EDGE('',*,*,#5088,.F.);
#6861=ORIENTED_EDGE('',*,*,#5087,.F.);
#6862=ORIENTED_EDGE('',*,*,#5089,.F.);
#6863=ORIENTED_EDGE('',*,*,#5090,.T.);
#6864=ORIENTED_EDGE('',*,*,#5091,.F.);
#6865=ORIENTED_EDGE('',*,*,#5090,.F.);
#6866=ORIENTED_EDGE('',*,*,#5056,.T.);
#6867=ORIENTED_EDGE('',*,*,#5092,.T.);
#6868=ORIENTED_EDGE('',*,*,#5060,.T.);
#6869=ORIENTED_EDGE('',*,*,#5092,.F.);
#6870=ORIENTED_EDGE('',*,*,#5093,.F.);
#6871=ORIENTED_EDGE('',*,*,#5089,.T.);
#6872=ORIENTED_EDGE('',*,*,#5094,.F.);
#6873=ORIENTED_EDGE('',*,*,#5095,.T.);
#6874=ORIENTED_EDGE('',*,*,#5093,.T.);
#6875=ORIENTED_EDGE('',*,*,#5095,.F.);
#6876=ORIENTED_EDGE('',*,*,#5094,.T.);
#6877=ORIENTED_EDGE('',*,*,#5073,.T.);
#6878=ORIENTED_EDGE('',*,*,#5096,.F.);
#6879=ORIENTED_EDGE('',*,*,#5086,.T.);
#6880=ORIENTED_EDGE('',*,*,#5097,.F.);
#6881=ORIENTED_EDGE('',*,*,#5098,.T.);
#6882=ORIENTED_EDGE('',*,*,#5096,.T.);
#6883=ORIENTED_EDGE('',*,*,#5098,.F.);
#6884=ORIENTED_EDGE('',*,*,#5097,.T.);
#6885=ORIENTED_EDGE('',*,*,#5091,.T.);
#6886=ORIENTED_EDGE('',*,*,#5099,.F.);
#6887=ORIENTED_EDGE('',*,*,#5080,.T.);
#6888=ORIENTED_EDGE('',*,*,#5100,.F.);
#6889=ORIENTED_EDGE('',*,*,#5101,.T.);
#6890=ORIENTED_EDGE('',*,*,#5099,.T.);
#6891=ORIENTED_EDGE('',*,*,#5101,.F.);
#6892=ORIENTED_EDGE('',*,*,#5100,.T.);
#6893=ORIENTED_EDGE('',*,*,#5088,.T.);
#6894=ORIENTED_EDGE('',*,*,#5102,.F.);
#6895=ORIENTED_EDGE('',*,*,#5083,.T.);
#6896=ORIENTED_EDGE('',*,*,#5103,.F.);
#6897=ORIENTED_EDGE('',*,*,#5104,.T.);
#6898=ORIENTED_EDGE('',*,*,#5102,.T.);
#6899=ORIENTED_EDGE('',*,*,#5104,.F.);
#6900=ORIENTED_EDGE('',*,*,#5103,.T.);
#6901=ORIENTED_EDGE('',*,*,#5082,.T.);
#6902=ORIENTED_EDGE('',*,*,#5105,.F.);
#6903=ORIENTED_EDGE('',*,*,#5106,.T.);
#6904=ORIENTED_EDGE('',*,*,#5107,.F.);
#6905=ORIENTED_EDGE('',*,*,#5108,.T.);
#6906=ORIENTED_EDGE('',*,*,#5105,.T.);
#6907=ORIENTED_EDGE('',*,*,#5108,.F.);
#6908=ORIENTED_EDGE('',*,*,#5107,.T.);
#6909=ORIENTED_EDGE('',*,*,#5085,.T.);
#6910=ORIENTED_EDGE('',*,*,#5106,.F.);
#6911=ORIENTED_EDGE('',*,*,#5109,.T.);
#6912=ORIENTED_EDGE('',*,*,#5020,.F.);
#6913=ORIENTED_EDGE('',*,*,#5109,.F.);
#9158=CYLINDRICAL_SURFACE('',#10266,0.0030735);
#9159=CYLINDRICAL_SURFACE('',#10269,0.0025175);
#9160=CYLINDRICAL_SURFACE('',#10278,0.004);
#9161=CYLINDRICAL_SURFACE('',#10284,0.008);
#9162=CYLINDRICAL_SURFACE('',#10292,0.0021);
#9163=CYLINDRICAL_SURFACE('',#10342,0.01115);
#9164=CYLINDRICAL_SURFACE('',#10344,0.01115);
#9165=CYLINDRICAL_SURFACE('',#10345,0.01115);
#9166=CYLINDRICAL_SURFACE('',#10346,0.01115);
#9167=CYLINDRICAL_SURFACE('',#10347,0.01115);
#9168=CYLINDRICAL_SURFACE('',#10348,0.01115);
#9169=CYLINDRICAL_SURFACE('',#10349,0.01115);
#9170=CYLINDRICAL_SURFACE('',#10350,0.01115);
#9171=CYLINDRICAL_SURFACE('',#10375,0.01115);
#9172=CYLINDRICAL_SURFACE('',#10380,0.01115);
#9173=CYLINDRICAL_SURFACE('',#10385,0.01115);
#9174=CYLINDRICAL_SURFACE('',#10390,0.008);
#9175=CYLINDRICAL_SURFACE('',#10396,0.008);
#9176=CYLINDRICAL_SURFACE('',#10399,0.006);
#9400=ADVANCED_FACE('',(#1178),#9158,.F.);
#9401=ADVANCED_FACE('',(#1179,#712),#9159,.F.);
#9402=ADVANCED_FACE('',(#1180),#613,.F.);
#9403=ADVANCED_FACE('',(#1181,#713),#912,.F.);
#9404=ADVANCED_FACE('',(#1182),#9160,.F.);
#9405=ADVANCED_FACE('',(#1183),#614,.T.);
#9406=ADVANCED_FACE('',(#1184),#9161,.T.);
#9407=ADVANCED_FACE('',(#1185,#714),#913,.T.);
#9408=ADVANCED_FACE('',(#1186),#615,.T.);
#9409=ADVANCED_FACE('',(#1187),#616,.F.);
#9410=ADVANCED_FACE('',(#1188),#9162,.F.);
#9411=ADVANCED_FACE('',(#1189),#914,.F.);
#9412=ADVANCED_FACE('',(#1190),#94,.F.);
#9413=ADVANCED_FACE('',(#1191),#95,.F.);
#9414=ADVANCED_FACE('',(#1192),#617,.F.);
#9415=ADVANCED_FACE('',(#1193,#715),#915,.T.);
#9416=ADVANCED_FACE('',(#1194,#716),#916,.T.);
#9417=ADVANCED_FACE('',(#1195,#717),#917,.T.);
#9418=ADVANCED_FACE('',(#1196,#718),#918,.T.);
#9419=ADVANCED_FACE('',(#1197,#719),#919,.T.);
#9420=ADVANCED_FACE('',(#1198,#720),#920,.T.);
#9421=ADVANCED_FACE('',(#1199,#721),#921,.T.);
#9422=ADVANCED_FACE('',(#1200,#722),#922,.T.);
#9423=ADVANCED_FACE('',(#1201,#723),#923,.T.);
#9424=ADVANCED_FACE('',(#1202,#724),#924,.T.);
#9425=ADVANCED_FACE('',(#1203,#725),#925,.T.);
#9426=ADVANCED_FACE('',(#1204,#726),#926,.F.);
#9427=ADVANCED_FACE('',(#1205,#727),#927,.T.);
#9428=ADVANCED_FACE('',(#1206,#728),#928,.T.);
#9429=ADVANCED_FACE('',(#1207,#729),#929,.F.);
#9430=ADVANCED_FACE('',(#1208),#9163,.T.);
#9431=ADVANCED_FACE('',(#1209),#9164,.T.);
#9432=ADVANCED_FACE('',(#1210),#9165,.T.);
#9433=ADVANCED_FACE('',(#1211),#9166,.T.);
#9434=ADVANCED_FACE('',(#1212),#9167,.T.);
#9435=ADVANCED_FACE('',(#1213),#9168,.T.);
#9436=ADVANCED_FACE('',(#1214),#9169,.T.);
#9437=ADVANCED_FACE('',(#1215),#9170,.T.);
#9438=ADVANCED_FACE('',(#1216),#618,.T.);
#9439=ADVANCED_FACE('',(#1217),#619,.T.);
#9440=ADVANCED_FACE('',(#1218),#620,.T.);
#9441=ADVANCED_FACE('',(#1219),#621,.T.);
#9442=ADVANCED_FACE('',(#1220),#622,.T.);
#9443=ADVANCED_FACE('',(#1221),#623,.T.);
#9444=ADVANCED_FACE('',(#1222),#624,.T.);
#9445=ADVANCED_FACE('',(#1223,#730),#930,.T.);
#9446=ADVANCED_FACE('',(#1224),#625,.T.);
#9447=ADVANCED_FACE('',(#1225),#626,.T.);
#9448=ADVANCED_FACE('',(#1226),#627,.T.);
#9449=ADVANCED_FACE('',(#1227),#628,.T.);
#9450=ADVANCED_FACE('',(#1228),#629,.T.);
#9451=ADVANCED_FACE('',(#1229,#731),#931,.F.);
#9452=ADVANCED_FACE('',(#1230),#9171,.T.);
#9453=ADVANCED_FACE('',(#1231,#732),#932,.T.);
#9454=ADVANCED_FACE('',(#1232,#733),#933,.F.);
#9455=ADVANCED_FACE('',(#1233),#9172,.T.);
#9456=ADVANCED_FACE('',(#1234,#734),#934,.T.);
#9457=ADVANCED_FACE('',(#1235,#735),#935,.F.);
#9458=ADVANCED_FACE('',(#1236),#9173,.T.);
#9459=ADVANCED_FACE('',(#1237,#736),#936,.T.);
#9460=ADVANCED_FACE('',(#1238,#737),#937,.F.);
#9461=ADVANCED_FACE('',(#1239),#9174,.T.);
#9462=ADVANCED_FACE('',(#1240,#738),#938,.T.);
#9463=ADVANCED_FACE('',(#1241,#739),#939,.F.);
#9464=ADVANCED_FACE('',(#1242),#9175,.T.);
#9465=ADVANCED_FACE('',(#1243,#740),#940,.T.);
#9466=ADVANCED_FACE('',(#1244),#9176,.T.);
#9869=CLOSED_SHELL('',(#9400,#9401,#9402,#9403,#9404,#9405,#9406,#9407,
#9408,#9409,#9410,#9411,#9412,#9413,#9414,#9415,#9416,#9417,#9418,#9419,
#9420,#9421,#9422,#9423,#9424,#9425,#9426,#9427,#9428,#9429,#9430,#9431,
#9432,#9433,#9434,#9435,#9436,#9437,#9438,#9439,#9440,#9441,#9442,#9443,
#9444,#9445,#9446,#9447,#9448,#9449,#9450,#9451,#9452,#9453,#9454,#9455,
#9456,#9457,#9458,#9459,#9460,#9461,#9462,#9463,#9464,#9465,#9466));
#10265=AXIS2_PLACEMENT_3D('',#13864,#11441,#11442);
#10266=AXIS2_PLACEMENT_3D('',#13865,#11443,#11444);
#10267=AXIS2_PLACEMENT_3D('',#14394,#11445,#11446);
#10268=AXIS2_PLACEMENT_3D('',#15155,#11447,#11448);
#10269=AXIS2_PLACEMENT_3D('',#15340,#11449,#11450);
#10270=AXIS2_PLACEMENT_3D('',#15832,#11451,#11452);
#10271=AXIS2_PLACEMENT_3D('',#16542,#11453,#11454);
#10272=AXIS2_PLACEMENT_3D('',#16778,#11455,#11456);
#10273=AXIS2_PLACEMENT_3D('',#16779,#11457,#11458);
#10274=AXIS2_PLACEMENT_3D('',#16781,#11459,#11460);
#10275=AXIS2_PLACEMENT_3D('',#16784,#11462,#11463);
#10276=AXIS2_PLACEMENT_3D('',#16785,#11464,#11465);
#10277=AXIS2_PLACEMENT_3D('',#16787,#11466,#11467);
#10278=AXIS2_PLACEMENT_3D('',#16788,#11468,#11469);
#10279=AXIS2_PLACEMENT_3D('',#16792,#11471,#11472);
#10280=AXIS2_PLACEMENT_3D('',#16793,#11473,#11474);
#10281=AXIS2_PLACEMENT_3D('',#16794,#11475,#11476);
#10282=AXIS2_PLACEMENT_3D('',#16796,#11477,#11478);
#10283=AXIS2_PLACEMENT_3D('',#16799,#11480,#11481);
#10284=AXIS2_PLACEMENT_3D('',#16800,#11482,#11483);
#10285=AXIS2_PLACEMENT_3D('',#16803,#11485,#11486);
#10286=AXIS2_PLACEMENT_3D('',#16804,#11487,#11488);
#10287=AXIS2_PLACEMENT_3D('',#16806,#11489,#11490);
#10288=AXIS2_PLACEMENT_3D('',#16807,#11491,#11492);
#10289=AXIS2_PLACEMENT_3D('',#16809,#11494,#11495);
#10290=AXIS2_PLACEMENT_3D('',#16812,#11496,#11497);
#10291=AXIS2_PLACEMENT_3D('',#16814,#11499,#11500);
#10292=AXIS2_PLACEMENT_3D('',#16815,#11501,#11502);
#10293=AXIS2_PLACEMENT_3D('',#16819,#11504,#11505);
#10294=AXIS2_PLACEMENT_3D('',#16820,#11506,#11507);
#10295=AXIS2_PLACEMENT_3D('',#16821,#11508,#11509);
#10296=AXIS2_PLACEMENT_3D('',#17807,#11510,#11511);
#10297=AXIS2_PLACEMENT_3D('',#17809,#11513,#11514);
#10298=AXIS2_PLACEMENT_3D('',#17811,#11515,#11516);
#10299=AXIS2_PLACEMENT_3D('',#17813,#11517,#11518);
#10300=AXIS2_PLACEMENT_3D('',#17814,#11519,#11520);
#10301=AXIS2_PLACEMENT_3D('',#17816,#11521,#11522);
#10302=AXIS2_PLACEMENT_3D('',#17818,#11523,#11524);
#10303=AXIS2_PLACEMENT_3D('',#17819,#11525,#11526);
#10304=AXIS2_PLACEMENT_3D('',#17821,#11527,#11528);
#10305=AXIS2_PLACEMENT_3D('',#17823,#11529,#11530);
#10306=AXIS2_PLACEMENT_3D('',#17824,#11531,#11532);
#10307=AXIS2_PLACEMENT_3D('',#17826,#11533,#11534);
#10308=AXIS2_PLACEMENT_3D('',#17828,#11535,#11536);
#10309=AXIS2_PLACEMENT_3D('',#17829,#11537,#11538);
#10310=AXIS2_PLACEMENT_3D('',#17831,#11539,#11540);
#10311=AXIS2_PLACEMENT_3D('',#17833,#11541,#11542);
#10312=AXIS2_PLACEMENT_3D('',#17834,#11543,#11544);
#10313=AXIS2_PLACEMENT_3D('',#17836,#11545,#11546);
#10314=AXIS2_PLACEMENT_3D('',#17838,#11547,#11548);
#10315=AXIS2_PLACEMENT_3D('',#17839,#11549,#11550);
#10316=AXIS2_PLACEMENT_3D('',#17841,#11551,#11552);
#10317=AXIS2_PLACEMENT_3D('',#17843,#11553,#11554);
#10318=AXIS2_PLACEMENT_3D('',#17844,#11555,#11556);
#10319=AXIS2_PLACEMENT_3D('',#17846,#11557,#11558);
#10320=AXIS2_PLACEMENT_3D('',#17848,#11559,#11560);
#10321=AXIS2_PLACEMENT_3D('',#17849,#11561,#11562);
#10322=AXIS2_PLACEMENT_3D('',#17851,#11563,#11564);
#10323=AXIS2_PLACEMENT_3D('',#17853,#11565,#11566);
#10324=AXIS2_PLACEMENT_3D('',#17854,#11567,#11568);
#10325=AXIS2_PLACEMENT_3D('',#17856,#11569,#11570);
#10326=AXIS2_PLACEMENT_3D('',#17858,#11571,#11572);
#10327=AXIS2_PLACEMENT_3D('',#17859,#11573,#11574);
#10328=AXIS2_PLACEMENT_3D('',#17861,#11575,#11576);
#10329=AXIS2_PLACEMENT_3D('',#17863,#11577,#11578);
#10330=AXIS2_PLACEMENT_3D('',#17864,#11579,#11580);
#10331=AXIS2_PLACEMENT_3D('',#17866,#11581,#11582);
#10332=AXIS2_PLACEMENT_3D('',#17868,#11583,#11584);
#10333=AXIS2_PLACEMENT_3D('',#17869,#11585,#11586);
#10334=AXIS2_PLACEMENT_3D('',#17871,#11587,#11588);
#10335=AXIS2_PLACEMENT_3D('',#17873,#11589,#11590);
#10336=AXIS2_PLACEMENT_3D('',#17874,#11591,#11592);
#10337=AXIS2_PLACEMENT_3D('',#17876,#11593,#11594);
#10338=AXIS2_PLACEMENT_3D('',#17878,#11595,#11596);
#10339=AXIS2_PLACEMENT_3D('',#17879,#11597,#11598);
#10340=AXIS2_PLACEMENT_3D('',#17881,#11599,#11600);
#10341=AXIS2_PLACEMENT_3D('',#17883,#11601,#11602);
#10342=AXIS2_PLACEMENT_3D('',#17884,#11603,#11604);
#10343=AXIS2_PLACEMENT_3D('',#17886,#11605,#11606);
#10344=AXIS2_PLACEMENT_3D('',#17888,#11608,#11609);
#10345=AXIS2_PLACEMENT_3D('',#17890,#11611,#11612);
#10346=AXIS2_PLACEMENT_3D('',#17892,#11614,#11615);
#10347=AXIS2_PLACEMENT_3D('',#17894,#11617,#11618);
#10348=AXIS2_PLACEMENT_3D('',#17896,#11620,#11621);
#10349=AXIS2_PLACEMENT_3D('',#17898,#11623,#11624);
#10350=AXIS2_PLACEMENT_3D('',#17900,#11626,#11627);
#10351=AXIS2_PLACEMENT_3D('',#17902,#11629,#11630);
#10352=AXIS2_PLACEMENT_3D('',#17905,#11632,#11633);
#10353=AXIS2_PLACEMENT_3D('',#17906,#11634,#11635);
#10354=AXIS2_PLACEMENT_3D('',#17908,#11637,#11638);
#10355=AXIS2_PLACEMENT_3D('',#17910,#11640,#11641);
#10356=AXIS2_PLACEMENT_3D('',#17912,#11643,#11644);
#10357=AXIS2_PLACEMENT_3D('',#17914,#11646,#11647);
#10358=AXIS2_PLACEMENT_3D('',#17916,#11649,#11650);
#10359=AXIS2_PLACEMENT_3D('',#17918,#11652,#11653);
#10360=AXIS2_PLACEMENT_3D('',#17919,#11654,#11655);
#10361=AXIS2_PLACEMENT_3D('',#17921,#11656,#11657);
#10362=AXIS2_PLACEMENT_3D('',#17924,#11659,#11660);
#10363=AXIS2_PLACEMENT_3D('',#17925,#11661,#11662);
#10364=AXIS2_PLACEMENT_3D('',#17927,#11663,#11664);
#10365=AXIS2_PLACEMENT_3D('',#17930,#11666,#11667);
#10366=AXIS2_PLACEMENT_3D('',#17931,#11668,#11669);
#10367=AXIS2_PLACEMENT_3D('',#17933,#11670,#11671);
#10368=AXIS2_PLACEMENT_3D('',#17936,#11673,#11674);
#10369=AXIS2_PLACEMENT_3D('',#17937,#11675,#11676);
#10370=AXIS2_PLACEMENT_3D('',#17939,#11677,#11678);
#10371=AXIS2_PLACEMENT_3D('',#17942,#11680,#11681);
#10372=AXIS2_PLACEMENT_3D('',#17943,#11682,#11683);
#10373=AXIS2_PLACEMENT_3D('',#17945,#11685,#11686);
#10374=AXIS2_PLACEMENT_3D('',#17947,#11687,#11688);
#10375=AXIS2_PLACEMENT_3D('',#17948,#11689,#11690);
#10376=AXIS2_PLACEMENT_3D('',#17950,#11691,#11692);
#10377=AXIS2_PLACEMENT_3D('',#17952,#11694,#11695);
#10378=AXIS2_PLACEMENT_3D('',#17953,#11696,#11697);
#10379=AXIS2_PLACEMENT_3D('',#17955,#11698,#11699);
#10380=AXIS2_PLACEMENT_3D('',#17956,#11700,#11701);
#10381=AXIS2_PLACEMENT_3D('',#17958,#11702,#11703);
#10382=AXIS2_PLACEMENT_3D('',#17960,#11705,#11706);
#10383=AXIS2_PLACEMENT_3D('',#17961,#11707,#11708);
#10384=AXIS2_PLACEMENT_3D('',#17963,#11709,#11710);
#10385=AXIS2_PLACEMENT_3D('',#17964,#11711,#11712);
#10386=AXIS2_PLACEMENT_3D('',#17966,#11713,#11714);
#10387=AXIS2_PLACEMENT_3D('',#17968,#11716,#11717);
#10388=AXIS2_PLACEMENT_3D('',#17969,#11718,#11719);
#10389=AXIS2_PLACEMENT_3D('',#17971,#11720,#11721);
#10390=AXIS2_PLACEMENT_3D('',#17972,#11722,#11723);
#10391=AXIS2_PLACEMENT_3D('',#17974,#11724,#11725);
#10392=AXIS2_PLACEMENT_3D('',#17976,#11727,#11728);
#10393=AXIS2_PLACEMENT_3D('',#17977,#11729,#11730);
#10394=AXIS2_PLACEMENT_3D('',#17979,#11731,#11732);
#10395=AXIS2_PLACEMENT_3D('',#17981,#11733,#11734);
#10396=AXIS2_PLACEMENT_3D('',#17982,#11735,#11736);
#10397=AXIS2_PLACEMENT_3D('',#17984,#11737,#11738);
#10398=AXIS2_PLACEMENT_3D('',#17986,#11740,#11741);
#10399=AXIS2_PLACEMENT_3D('',#17987,#11742,#11743);
#11441=DIRECTION('axis',(0.,0.,1.));
#11442=DIRECTION('refdir',(1.,0.,0.));
#11443=DIRECTION('center_axis',(-2.37714673961354E-29,1.,6.52256026967277E-16));
#11444=DIRECTION('ref_axis',(-1.,-9.36001528722827E-29,1.07057171707285E-13));
#11445=DIRECTION('center_axis',(-3.25361965184118E-12,-1.,3.25296739583608E-12));
#11446=DIRECTION('ref_axis',(-1.,3.25361965185211E-12,3.36067682355905E-12));
#11447=DIRECTION('center_axis',(3.25361965184118E-12,1.,-3.25296739583608E-12));
#11448=DIRECTION('ref_axis',(-1.,3.25361965185211E-12,3.36067682355905E-12));
#11449=DIRECTION('center_axis',(0.,1.,6.52256026967277E-16));
#11450=DIRECTION('ref_axis',(-1.,0.,0.));
#11451=DIRECTION('center_axis',(0.,-1.,3.9715423814945E-12));
#11452=DIRECTION('ref_axis',(-1.,0.,0.));
#11453=DIRECTION('center_axis',(0.,1.,-3.9715423814945E-12));
#11454=DIRECTION('ref_axis',(-1.,0.,0.));
#11455=DIRECTION('center_axis',(0.,1.,-3.9715423814945E-12));
#11456=DIRECTION('ref_axis',(-1.,0.,0.));
#11457=DIRECTION('center_axis',(0.,1.,1.09634523681734E-15));
#11458=DIRECTION('ref_axis',(-1.,0.,0.));
#11459=DIRECTION('center_axis',(0.,-1.,2.49912569936186E-12));
#11460=DIRECTION('ref_axis',(-1.,0.,0.));
#11461=DIRECTION('',(0.707106781186547,0.707106781186548,6.88637545851563E-16));
#11462=DIRECTION('center_axis',(0.,1.,-2.38007808031482E-12));
#11463=DIRECTION('ref_axis',(-1.,0.,0.));
#11464=DIRECTION('center_axis',(0.,-1.,-8.74300631892309E-16));
#11465=DIRECTION('ref_axis',(0.,-8.74300631892309E-16,1.));
#11466=DIRECTION('center_axis',(0.,-1.,1.28117698141774E-12));
#11467=DIRECTION('ref_axis',(1.,0.,0.));
#11468=DIRECTION('center_axis',(0.,-1.,-8.74300631892318E-16));
#11469=DIRECTION('ref_axis',(-1.,0.,0.));
#11470=DIRECTION('',(0.,-1.,-8.74300631892318E-16));
#11471=DIRECTION('center_axis',(0.,-1.,2.49912569936186E-12));
#11472=DIRECTION('ref_axis',(-1.,0.,0.));
#11473=DIRECTION('center_axis',(0.,-1.,2.49912569936186E-12));
#11474=DIRECTION('ref_axis',(-1.,0.,0.));
#11475=DIRECTION('center_axis',(0.,1.,1.09634523681734E-15));
#11476=DIRECTION('ref_axis',(1.,0.,0.));
#11477=DIRECTION('center_axis',(0.,-1.,1.24912569936654E-12));
#11478=DIRECTION('ref_axis',(1.,0.,0.));
#11479=DIRECTION('',(0.707106781186547,-0.707106781186548,-8.61828757098662E-16));
#11480=DIRECTION('center_axis',(0.,1.,-1.28117698141774E-12));
#11481=DIRECTION('ref_axis',(1.,0.,0.));
#11482=DIRECTION('center_axis',(0.,-1.,-8.74300631892309E-16));
#11483=DIRECTION('ref_axis',(1.,0.,0.));
#11484=DIRECTION('',(0.,1.,8.74300631892309E-16));
#11485=DIRECTION('center_axis',(0.,1.,-1.24912569936654E-12));
#11486=DIRECTION('ref_axis',(1.,0.,0.));
#11487=DIRECTION('center_axis',(0.,-1.,-8.74300631892309E-16));
#11488=DIRECTION('ref_axis',(0.,-8.74300631892309E-16,1.));
#11489=DIRECTION('center_axis',(0.,1.,-1.665792366032E-12));
#11490=DIRECTION('ref_axis',(-1.,0.,0.));
#11491=DIRECTION('center_axis',(0.,-1.,-1.09634523681734E-15));
#11492=DIRECTION('ref_axis',(1.,0.,0.));
#11493=DIRECTION('',(0.707106781186547,0.707106781186548,8.61828757098662E-16));
#11494=DIRECTION('center_axis',(0.,1.,8.74300631892318E-16));
#11495=DIRECTION('ref_axis',(1.,0.,0.));
#11496=DIRECTION('center_axis',(0.,-1.,4.76103046125019E-12));
#11497=DIRECTION('ref_axis',(1.,0.,0.));
#11498=DIRECTION('',(-0.707106781186547,0.707106781186548,7.04819511230291E-16));
#11499=DIRECTION('center_axis',(0.,-1.,4.76103046125019E-12));
#11500=DIRECTION('ref_axis',(1.,0.,0.));
#11501=DIRECTION('center_axis',(0.,-1.,-8.74300631892318E-16));
#11502=DIRECTION('ref_axis',(-1.,0.,0.));
#11503=DIRECTION('',(0.,-1.,-8.74300631892318E-16));
#11504=DIRECTION('center_axis',(0.,1.,-4.76103046125019E-12));
#11505=DIRECTION('ref_axis',(-1.,0.,0.));
#11506=DIRECTION('center_axis',(0.,1.,-4.76103046125019E-12));
#11507=DIRECTION('ref_axis',(-1.,0.,0.));
#11508=DIRECTION('center_axis',(0.,1.,6.52256026967277E-16));
#11509=DIRECTION('ref_axis',(1.,0.,0.));
#11510=DIRECTION('center_axis',(0.,-1.,-6.52256026967277E-16));
#11511=DIRECTION('ref_axis',(1.,0.,0.));
#11512=DIRECTION('',(-0.813733471206735,-0.581238193719097,-4.78769724044094E-16));
#11513=DIRECTION('center_axis',(0.,1.,6.52256026967277E-16));
#11514=DIRECTION('ref_axis',(1.,0.,0.));
#11515=DIRECTION('center_axis',(0.,1.,-8.96208730519314E-13));
#11516=DIRECTION('ref_axis',(1.,0.,0.));
#11517=DIRECTION('center_axis',(0.,1.,-1.66030339217348E-12));
#11518=DIRECTION('ref_axis',(-1.,0.,0.));
#11519=DIRECTION('center_axis',(0.,1.,6.52256026967277E-16));
#11520=DIRECTION('ref_axis',(1.,0.,0.));
#11521=DIRECTION('center_axis',(0.,1.,-8.96208730519314E-13));
#11522=DIRECTION('ref_axis',(1.,0.,0.));
#11523=DIRECTION('center_axis',(0.,1.,-1.69748481005457E-12));
#11524=DIRECTION('ref_axis',(-1.,0.,0.));
#11525=DIRECTION('center_axis',(0.,-1.,-6.52256026967277E-16));
#11526=DIRECTION('ref_axis',(0.,-6.52256026967277E-16,1.));
#11527=DIRECTION('center_axis',(0.,-1.,8.96208730519314E-13));
#11528=DIRECTION('ref_axis',(1.,0.,0.));
#11529=DIRECTION('center_axis',(0.,-1.,1.68250544832888E-12));
#11530=DIRECTION('ref_axis',(-1.,0.,0.));
#11531=DIRECTION('center_axis',(0.,1.,6.52256026967277E-16));
#11532=DIRECTION('ref_axis',(1.,0.,0.));
#11533=DIRECTION('center_axis',(0.,1.,-8.96208730519314E-13));
#11534=DIRECTION('ref_axis',(1.,0.,0.));
#11535=DIRECTION('center_axis',(0.,1.,-1.73612621739787E-12));
#11536=DIRECTION('ref_axis',(-1.,0.,0.));
#11537=DIRECTION('center_axis',(0.,-1.,-6.52256026967277E-16));
#11538=DIRECTION('ref_axis',(0.,-6.52256026967277E-16,1.));
#11539=DIRECTION('center_axis',(0.,-1.,8.96208730519314E-13));
#11540=DIRECTION('ref_axis',(1.,0.,0.));
#11541=DIRECTION('center_axis',(0.,-1.,1.7204605278621E-12));
#11542=DIRECTION('ref_axis',(-1.,0.,0.));
#11543=DIRECTION('center_axis',(0.,1.,6.52256026967277E-16));
#11544=DIRECTION('ref_axis',(1.,0.,0.));
#11545=DIRECTION('center_axis',(0.,1.,-8.96208730519314E-13));
#11546=DIRECTION('ref_axis',(1.,0.,0.));
#11547=DIRECTION('center_axis',(0.,1.,-1.77656715745294E-12));
#11548=DIRECTION('ref_axis',(-1.,0.,0.));
#11549=DIRECTION('center_axis',(0.,-1.,-6.52256026967277E-16));
#11550=DIRECTION('ref_axis',(0.,-6.52256026967277E-16,1.));
#11551=DIRECTION('center_axis',(0.,-1.,8.96208730519314E-13));
#11552=DIRECTION('ref_axis',(1.,0.,0.));
#11553=DIRECTION('center_axis',(0.,-1.,1.76016686652978E-12));
#11554=DIRECTION('ref_axis',(-1.,0.,0.));
#11555=DIRECTION('center_axis',(0.,1.,6.52256026967277E-16));
#11556=DIRECTION('ref_axis',(1.,0.,0.));
#11557=DIRECTION('center_axis',(0.,1.,-8.96208730519314E-13));
#11558=DIRECTION('ref_axis',(1.,0.,0.));
#11559=DIRECTION('center_axis',(0.,1.,-1.81893633360534E-12));
#11560=DIRECTION('ref_axis',(-1.,0.,0.));
#11561=DIRECTION('center_axis',(0.,-1.,-6.52256026967277E-16));
#11562=DIRECTION('ref_axis',(0.,-6.52256026967277E-16,1.));
#11563=DIRECTION('center_axis',(0.,-1.,8.96208730519314E-13));
#11564=DIRECTION('ref_axis',(1.,0.,0.));
#11565=DIRECTION('center_axis',(0.,-1.,1.80174853205239E-12));
#11566=DIRECTION('ref_axis',(-1.,0.,0.));
#11567=DIRECTION('center_axis',(0.,1.,6.52256026967277E-16));
#11568=DIRECTION('ref_axis',(1.,0.,0.));
#11569=DIRECTION('center_axis',(0.,1.,-8.96208730519314E-13));
#11570=DIRECTION('ref_axis',(1.,0.,0.));
#11571=DIRECTION('center_axis',(0.,1.,-1.86337502221387E-12));
#11572=DIRECTION('ref_axis',(-1.,0.,0.));
#11573=DIRECTION('center_axis',(0.,-1.,-6.52256026967277E-16));
#11574=DIRECTION('ref_axis',(0.,-6.52256026967277E-16,1.));
#11575=DIRECTION('center_axis',(0.,-1.,8.96208730519314E-13));
#11576=DIRECTION('ref_axis',(1.,0.,0.));
#11577=DIRECTION('center_axis',(0.,-1.,1.84534159501235E-12));
#11578=DIRECTION('ref_axis',(-1.,0.,0.));
#11579=DIRECTION('center_axis',(0.,-1.,-8.74300631892309E-16));
#11580=DIRECTION('ref_axis',(0.,-8.74300631892309E-16,1.));
#11581=DIRECTION('center_axis',(0.,-1.,8.95986685914389E-13));
#11582=DIRECTION('ref_axis',(-1.,0.,0.));
#11583=DIRECTION('center_axis',(0.,1.,-1.90981660175007E-12));
#11584=DIRECTION('ref_axis',(-1.,0.,0.));
#11585=DIRECTION('center_axis',(0.,-1.,-8.74300631892309E-16));
#11586=DIRECTION('ref_axis',(0.,-8.74300631892309E-16,1.));
#11587=DIRECTION('center_axis',(0.,-1.,8.95986685914389E-13));
#11588=DIRECTION('ref_axis',(-1.,0.,0.));
#11589=DIRECTION('center_axis',(0.,-1.,1.89087357173833E-12));
#11590=DIRECTION('ref_axis',(-1.,0.,0.));
#11591=DIRECTION('center_axis',(0.,-1.,-8.74300631892309E-16));
#11592=DIRECTION('ref_axis',(0.,-8.74300631892309E-16,1.));
#11593=DIRECTION('center_axis',(0.,-1.,8.95986685914389E-13));
#11594=DIRECTION('ref_axis',(-1.,0.,0.));
#11595=DIRECTION('center_axis',(0.,-1.,1.93895331704599E-12));
#11596=DIRECTION('ref_axis',(-1.,0.,0.));
#11597=DIRECTION('center_axis',(0.,-1.,-8.74300631892309E-16));
#11598=DIRECTION('ref_axis',(0.,-8.74300631892309E-16,1.));
#11599=DIRECTION('center_axis',(0.,-1.,8.95986685914389E-13));
#11600=DIRECTION('ref_axis',(-1.,0.,0.));
#11601=DIRECTION('center_axis',(0.,1.,-1.95887654741229E-12));
#11602=DIRECTION('ref_axis',(-1.,0.,0.));
#11603=DIRECTION('center_axis',(0.,-1.,-6.52256026967277E-16));
#11604=DIRECTION('ref_axis',(1.,0.,0.));
#11605=DIRECTION('center_axis',(0.,-1.,8.96208730519314E-13));
#11606=DIRECTION('ref_axis',(1.,0.,0.));
#11607=DIRECTION('',(0.,1.,6.52256026967277E-16));
#11608=DIRECTION('center_axis',(0.,-1.,-6.52256026967277E-16));
#11609=DIRECTION('ref_axis',(1.,0.,0.));
#11610=DIRECTION('',(0.,1.,6.52256026967277E-16));
#11611=DIRECTION('center_axis',(0.,-1.,-6.52256026967277E-16));
#11612=DIRECTION('ref_axis',(1.,0.,0.));
#11613=DIRECTION('',(0.,1.,6.52256026967277E-16));
#11614=DIRECTION('center_axis',(0.,-1.,-6.52256026967277E-16));
#11615=DIRECTION('ref_axis',(1.,0.,0.));
#11616=DIRECTION('',(0.,1.,6.52256026967277E-16));
#11617=DIRECTION('center_axis',(0.,-1.,-6.52256026967277E-16));
#11618=DIRECTION('ref_axis',(1.,0.,0.));
#11619=DIRECTION('',(0.,1.,6.52256026967277E-16));
#11620=DIRECTION('center_axis',(0.,-1.,-6.52256026967277E-16));
#11621=DIRECTION('ref_axis',(1.,0.,0.));
#11622=DIRECTION('',(0.,1.,6.52256026967277E-16));
#11623=DIRECTION('center_axis',(0.,-1.,-8.74300631892309E-16));
#11624=DIRECTION('ref_axis',(-1.,0.,0.));
#11625=DIRECTION('',(0.,1.,8.74300631892309E-16));
#11626=DIRECTION('center_axis',(0.,-1.,-8.74300631892309E-16));
#11627=DIRECTION('ref_axis',(-1.,0.,0.));
#11628=DIRECTION('',(0.,1.,8.74300631892309E-16));
#11629=DIRECTION('center_axis',(0.,-1.,-8.74300631892309E-16));
#11630=DIRECTION('ref_axis',(-1.,0.,0.));
#11631=DIRECTION('',(-0.0523359562429438,0.998629534754574,8.66693127132923E-16));
#11632=DIRECTION('center_axis',(0.,1.,-1.98954073916915E-12));
#11633=DIRECTION('ref_axis',(-1.,0.,0.));
#11634=DIRECTION('center_axis',(0.,-1.,-8.74300631892309E-16));
#11635=DIRECTION('ref_axis',(-1.,0.,0.));
#11636=DIRECTION('',(-0.0523359562429438,0.998629534754574,8.66693127132923E-16));
#11637=DIRECTION('center_axis',(0.,-1.,-8.74300631892309E-16));
#11638=DIRECTION('ref_axis',(-1.,0.,0.));
#11639=DIRECTION('',(-0.0523359562429438,0.998629534754574,8.66693127132923E-16));
#11640=DIRECTION('center_axis',(0.,-1.,-8.74300631892309E-16));
#11641=DIRECTION('ref_axis',(-1.,0.,0.));
#11642=DIRECTION('',(-0.0523359562429438,0.998629534754574,8.66693127132923E-16));
#11643=DIRECTION('center_axis',(0.,-1.,-8.74300631892309E-16));
#11644=DIRECTION('ref_axis',(-1.,0.,0.));
#11645=DIRECTION('',(-0.0523359562429438,0.998629534754574,8.66693127132923E-16));
#11646=DIRECTION('center_axis',(0.,-1.,-8.74300631892309E-16));
#11647=DIRECTION('ref_axis',(-1.,0.,0.));
#11648=DIRECTION('',(-0.0523359562429438,0.998629534754574,8.66693127132923E-16));
#11649=DIRECTION('center_axis',(0.,-1.,-8.74300631892309E-16));
#11650=DIRECTION('ref_axis',(-1.,0.,0.));
#11651=DIRECTION('',(-0.0523359562429438,0.998629534754574,8.66693127132923E-16));
#11652=DIRECTION('center_axis',(0.,-1.,-6.52256026967277E-16));
#11653=DIRECTION('ref_axis',(0.,-6.52256026967277E-16,1.));
#11654=DIRECTION('center_axis',(0.,-1.,-8.74300631892309E-16));
#11655=DIRECTION('ref_axis',(-1.,0.,0.));
#11656=DIRECTION('center_axis',(0.,-1.,2.12243424546674E-12));
#11657=DIRECTION('ref_axis',(-1.,0.,0.));
#11658=DIRECTION('',(-0.0523359562429438,0.998629534754574,8.66693127132923E-16));
#11659=DIRECTION('center_axis',(0.,1.,-2.15847746020963E-12));
#11660=DIRECTION('ref_axis',(-1.,0.,0.));
#11661=DIRECTION('center_axis',(0.,-1.,-8.74300631892309E-16));
#11662=DIRECTION('ref_axis',(-1.,0.,0.));
#11663=DIRECTION('center_axis',(0.,-1.,2.18319386742199E-12));
#11664=DIRECTION('ref_axis',(-1.,0.,0.));
#11665=DIRECTION('',(-0.0523359562429438,0.998629534754574,8.66693127132923E-16));
#11666=DIRECTION('center_axis',(0.,1.,-2.2213479215854E-12));
#11667=DIRECTION('ref_axis',(-1.,0.,0.));
#11668=DIRECTION('center_axis',(0.,-1.,-8.74300631892309E-16));
#11669=DIRECTION('ref_axis',(-1.,0.,0.));
#11670=DIRECTION('center_axis',(0.,-1.,2.0649637236167E-12));
#11671=DIRECTION('ref_axis',(-1.,0.,0.));
#11672=DIRECTION('',(-0.0523359562429438,0.998629534754574,8.66693127132923E-16));
#11673=DIRECTION('center_axis',(0.,1.,-2.09906654771079E-12));
#11674=DIRECTION('ref_axis',(-1.,0.,0.));
#11675=DIRECTION('center_axis',(0.,-1.,-8.74300631892309E-16));
#11676=DIRECTION('ref_axis',(-1.,0.,0.));
#11677=DIRECTION('center_axis',(0.,-1.,2.0105222668657E-12));
#11678=DIRECTION('ref_axis',(-1.,0.,0.));
#11679=DIRECTION('',(-0.0523359562429438,0.998629534754574,8.66693127132923E-16));
#11680=DIRECTION('center_axis',(0.,1.,-2.0428372792574E-12));
#11681=DIRECTION('ref_axis',(-1.,0.,0.));
#11682=DIRECTION('center_axis',(0.,-1.,-8.74300631892309E-16));
#11683=DIRECTION('ref_axis',(-1.,0.,0.));
#11684=DIRECTION('',(-0.0523359562429438,0.998629534754574,8.66693127132923E-16));
#11685=DIRECTION('center_axis',(0.,-1.,-8.74300631892309E-16));
#11686=DIRECTION('ref_axis',(0.,-8.74300631892309E-16,1.));
#11687=DIRECTION('center_axis',(0.,-1.,8.95986685914389E-13));
#11688=DIRECTION('ref_axis',(-1.,0.,0.));
#11689=DIRECTION('center_axis',(0.,-1.,-8.74300631892309E-16));
#11690=DIRECTION('ref_axis',(-1.,0.,0.));
#11691=DIRECTION('center_axis',(0.,-1.,8.95986685914389E-13));
#11692=DIRECTION('ref_axis',(-1.,0.,0.));
#11693=DIRECTION('',(0.,1.,8.74300631892309E-16));
#11694=DIRECTION('center_axis',(0.,-1.,-8.74300631892309E-16));
#11695=DIRECTION('ref_axis',(0.,-8.74300631892309E-16,1.));
#11696=DIRECTION('center_axis',(0.,-1.,-8.74300631892309E-16));
#11697=DIRECTION('ref_axis',(0.,-8.74300631892309E-16,1.));
#11698=DIRECTION('center_axis',(0.,-1.,8.95986685914389E-13));
#11699=DIRECTION('ref_axis',(-1.,0.,0.));
#11700=DIRECTION('center_axis',(0.,-1.,-8.74300631892309E-16));
#11701=DIRECTION('ref_axis',(-1.,0.,0.));
#11702=DIRECTION('center_axis',(0.,-1.,8.95986685914389E-13));
#11703=DIRECTION('ref_axis',(-1.,0.,0.));
#11704=DIRECTION('',(0.,1.,8.74300631892309E-16));
#11705=DIRECTION('center_axis',(0.,-1.,-8.74300631892309E-16));
#11706=DIRECTION('ref_axis',(0.,-8.74300631892309E-16,1.));
#11707=DIRECTION('center_axis',(0.,-1.,-8.74300631892309E-16));
#11708=DIRECTION('ref_axis',(0.,-8.74300631892309E-16,1.));
#11709=DIRECTION('center_axis',(0.,-1.,8.95986685914389E-13));
#11710=DIRECTION('ref_axis',(-1.,0.,0.));
#11711=DIRECTION('center_axis',(0.,-1.,-8.74300631892309E-16));
#11712=DIRECTION('ref_axis',(-1.,0.,0.));
#11713=DIRECTION('center_axis',(0.,-1.,8.95986685914389E-13));
#11714=DIRECTION('ref_axis',(-1.,0.,0.));
#11715=DIRECTION('',(0.,1.,8.74300631892309E-16));
#11716=DIRECTION('center_axis',(0.,-1.,-8.74300631892309E-16));
#11717=DIRECTION('ref_axis',(0.,-8.74300631892309E-16,1.));
#11718=DIRECTION('center_axis',(0.,-1.,-8.74300631892309E-16));
#11719=DIRECTION('ref_axis',(0.,-8.74300631892309E-16,1.));
#11720=DIRECTION('center_axis',(0.,-1.,1.24912569936654E-12));
#11721=DIRECTION('ref_axis',(-1.,0.,0.));
#11722=DIRECTION('center_axis',(0.,-1.,-8.74300631892309E-16));
#11723=DIRECTION('ref_axis',(-1.,0.,0.));
#11724=DIRECTION('center_axis',(0.,-1.,1.24912569936654E-12));
#11725=DIRECTION('ref_axis',(-1.,0.,0.));
#11726=DIRECTION('',(0.,1.,8.74300631892309E-16));
#11727=DIRECTION('center_axis',(0.,-1.,-8.74300631892309E-16));
#11728=DIRECTION('ref_axis',(0.,-8.74300631892309E-16,1.));
#11729=DIRECTION('center_axis',(0.,-1.,-8.74300631892309E-16));
#11730=DIRECTION('ref_axis',(0.,-8.74300631892309E-16,1.));
#11731=DIRECTION('center_axis',(0.,-1.,1.24912569936654E-12));
#11732=DIRECTION('ref_axis',(-1.,0.,0.));
#11733=DIRECTION('center_axis',(0.,-1.,1.665792366032E-12));
#11734=DIRECTION('ref_axis',(-1.,0.,0.));
#11735=DIRECTION('center_axis',(0.,-1.,-8.74300631892309E-16));
#11736=DIRECTION('ref_axis',(-1.,0.,0.));
#11737=DIRECTION('center_axis',(0.,-1.,1.24912569936654E-12));
#11738=DIRECTION('ref_axis',(-1.,0.,0.));
#11739=DIRECTION('',(0.,1.,8.74300631892309E-16));
#11740=DIRECTION('center_axis',(0.,-1.,-8.74300631892309E-16));
#11741=DIRECTION('ref_axis',(0.,-8.74300631892309E-16,1.));
#11742=DIRECTION('center_axis',(0.,-1.,-8.74300631892309E-16));
#11743=DIRECTION('ref_axis',(-1.,0.,0.));
#11744=DIRECTION('',(0.,1.,8.74300631892309E-16));
#13864=CARTESIAN_POINT('',(0.,0.,0.));
#13865=CARTESIAN_POINT('Origin',(0.,-0.0291247811395418,-0.0121758532865581));
#13866=CARTESIAN_POINT('',(0.00307327823453674,-0.0236251335354893,-0.0121742489211595));
#13867=CARTESIAN_POINT('',(0.00307327999164594,-0.0226251873529714,-0.0121774473169523));
#13868=CARTESIAN_POINT('Ctrl Pts',(0.00307266966487839,-0.0236261040574453,
-0.0121759154876736));
#13869=CARTESIAN_POINT('Ctrl Pts',(0.00307016915329888,-0.0235977132371358,
-0.0127445659805958));
#13870=CARTESIAN_POINT('Ctrl Pts',(0.00291138345935846,-0.0235660101645814,
-0.0133130648648865));
#13871=CARTESIAN_POINT('Ctrl Pts',(0.00261246228220724,-0.0235347411284561,
-0.0137968579377696));
#13872=CARTESIAN_POINT('Ctrl Pts',(0.00256279224538186,-0.0235295453300498,
-0.0138772470891003));
#13873=CARTESIAN_POINT('Ctrl Pts',(0.00250945992878158,-0.0235245080538991,
-0.0139553652459075));
#13874=CARTESIAN_POINT('Ctrl Pts',(0.00245251305124659,-0.0235196091447056,
-0.0140307197566707));
#13875=CARTESIAN_POINT('Ctrl Pts',(0.00236729119587557,-0.0235122778537054,
-0.0141434889109384));
#13876=CARTESIAN_POINT('Ctrl Pts',(0.00227396676332056,-0.0235052564434052,
-0.0142500644674973));
#13877=CARTESIAN_POINT('Ctrl Pts',(0.00217394442652592,-0.0234984773627037,
-0.0143496603071668));
#13878=CARTESIAN_POINT('Ctrl Pts',(0.00177992504288088,-0.0234717724357315,
-0.0147419995847498));
#13879=CARTESIAN_POINT('Ctrl Pts',(0.00127516616801139,-0.0234445247812332,
-0.0150239885753106));
#13880=CARTESIAN_POINT('Ctrl Pts',(0.00073465934568833,-0.0234142110768737,
-0.0151592520636632));
#13881=CARTESIAN_POINT('Ctrl Pts',(0.000494490103978782,-0.023400741460786,
-0.0152193551522589));
#13882=CARTESIAN_POINT('Ctrl Pts',(0.000247123644285777,-0.023386522593376,
-0.0152501029941088));
#13883=CARTESIAN_POINT('Ctrl Pts',(1.40972321978975E-7,-0.0233730175728703,
-0.0152504987812254));
#13884=CARTESIAN_POINT('Ctrl Pts',(-7.83185877626713E-5,-0.0233687274015826,
-0.0152506245118397));
#13885=CARTESIAN_POINT('Ctrl Pts',(-0.000156800353640954,-0.0233645659408657,
-0.0152477937223375));
#13886=CARTESIAN_POINT('Ctrl Pts',(-0.000235091041689717,-0.0233605024316512,
-0.0152418357342434));
#13887=CARTESIAN_POINT('Ctrl Pts',(-0.000695274669722541,-0.0233366175934987,
-0.0152068153678981));
#13888=CARTESIAN_POINT('Ctrl Pts',(-0.00115014572941729,-0.0233161169334347,
-0.015062471823434));
#13889=CARTESIAN_POINT('Ctrl Pts',(-0.00154928198099346,-0.0232927539572789,
-0.0148289427165404));
#13890=CARTESIAN_POINT('Ctrl Pts',(-0.00177706402867699,-0.0232794210001052,
-0.0146956705871563));
#13891=CARTESIAN_POINT('Ctrl Pts',(-0.00198730690683751,-0.0232652961508513,
-0.0145337037807864));
#13892=CARTESIAN_POINT('Ctrl Pts',(-0.00217300374575874,-0.023250687363939,
-0.014348841907857));
#13893=CARTESIAN_POINT('Ctrl Pts',(-0.00238459919233331,-0.0232340411312481,
-0.014138197877596));
#13894=CARTESIAN_POINT('Ctrl Pts',(-0.00256713902217867,-0.0232182993007945,
-0.0138989931398254));
#13895=CARTESIAN_POINT('Ctrl Pts',(-0.0027091022637822,-0.023202981860163,
-0.0136364623794192));
#13896=CARTESIAN_POINT('Ctrl Pts',(-0.00290226137111884,-0.023182140527395,
-0.0132792557761064));
#13897=CARTESIAN_POINT('Ctrl Pts',(-0.00302027471933705,-0.0231620848706945,
-0.0128785372613051));
#13898=CARTESIAN_POINT('Ctrl Pts',(-0.00305878637852152,-0.0231416057675226,
-0.0124657293521869));
#13899=CARTESIAN_POINT('Ctrl Pts',(-0.00306774188078499,-0.0231368435563198,
-0.012369734989888));
#13900=CARTESIAN_POINT('Ctrl Pts',(-0.00307226364115996,-0.0231319708591869,
-0.0122729662540278));
#13901=CARTESIAN_POINT('Ctrl Pts',(-0.00307223516061164,-0.0231269651224307,
-0.0121757719601571));
#13902=CARTESIAN_POINT('Ctrl Pts',(-0.00307211467525599,-0.0231057886350063,
-0.0117645969739148));
#13903=CARTESIAN_POINT('Ctrl Pts',(-0.00298797170067459,-0.0230814861616835,
-0.011344231287885));
#13904=CARTESIAN_POINT('Ctrl Pts',(-0.00282463481379235,-0.0230585539910371,
-0.0109620988921809));
#13905=CARTESIAN_POINT('Ctrl Pts',(-0.00278445639446726,-0.0230529130217137,
-0.0108681000660409));
#13906=CARTESIAN_POINT('Ctrl Pts',(-0.0027398227705807,-0.0230475030896191,
-0.0107763253627915));
#13907=CARTESIAN_POINT('Ctrl Pts',(-0.00269066644906558,-0.0230422565180116,
-0.0106872915136893));
#13908=CARTESIAN_POINT('Ctrl Pts',(-0.0025399881165119,-0.0230261742596757,
-0.0104143770337189));
#13909=CARTESIAN_POINT('Ctrl Pts',(-0.00234664362815788,-0.0230116269359496,
-0.0101670750656678));
#13910=CARTESIAN_POINT('Ctrl Pts',(-0.00212290995656839,-0.0229966653588366,
-0.00995470874154361));
#13911=CARTESIAN_POINT('Ctrl Pts',(-0.00171792617680668,-0.0229695831766718,
-0.00957030117326437));
#13912=CARTESIAN_POINT('Ctrl Pts',(-0.00120940308263932,-0.0229397098462347,
-0.00929766716641838));
#13913=CARTESIAN_POINT('Ctrl Pts',(-0.000670241834339137,-0.0229087613604071,
-0.00917583945292269));
#13914=CARTESIAN_POINT('Ctrl Pts',(-0.000515800944709547,-0.0228998962728308,
-0.00914094232240165));
#13915=CARTESIAN_POINT('Ctrl Pts',(-0.000358970911346579,-0.0228912777688333,
-0.00911794398325095));
#13916=CARTESIAN_POINT('Ctrl Pts',(-0.000201812288102591,-0.0228830565703485,
-0.00910763794284517));
#13917=CARTESIAN_POINT('Ctrl Pts',(-0.000103652758974647,-0.0228779217011604,
-0.00910120090456802));
#13918=CARTESIAN_POINT('Ctrl Pts',(-5.36347989276417E-6,-0.0228729418253322,
-0.00909970729402443));
#13919=CARTESIAN_POINT('Ctrl Pts',(9.25541750715132E-5,-0.0228681536676443,
-0.00910282920369337));
#13920=CARTESIAN_POINT('Ctrl Pts',(0.000650123353395021,-0.0228408886238822,
-0.00912060618793129));
#13921=CARTESIAN_POINT('Ctrl Pts',(0.00119953279408264,-0.0228146503881801,
-0.00929613564276958));
#13922=CARTESIAN_POINT('Ctrl Pts',(0.00166459553365405,-0.0227849878508226,
-0.00959380052075975));
#13923=CARTESIAN_POINT('Ctrl Pts',(0.0018684611856092,-0.0227719849331462,
-0.00972428537635481));
#13924=CARTESIAN_POINT('Ctrl Pts',(0.00205606806776706,-0.0227582037588869,
-0.00987855234620668));
#13925=CARTESIAN_POINT('Ctrl Pts',(0.00222231380956152,-0.0227448458698992,
-0.0100517128871323));
#13926=CARTESIAN_POINT('Ctrl Pts',(0.0023120057077202,-0.0227376391023406,
-0.0101451354159391));
#13927=CARTESIAN_POINT('Ctrl Pts',(0.00239582829502692,-0.0227307808936713,
-0.0102438423450844));
#13928=CARTESIAN_POINT('Ctrl Pts',(0.00247270790098799,-0.0227241552630883,
-0.0103475351539342));
#13929=CARTESIAN_POINT('Ctrl Pts',(0.00273607139307683,-0.0227014580967096,
-0.0107027515979027));
#13930=CARTESIAN_POINT('Ctrl Pts',(0.00291787292036907,-0.0226814902703287,
-0.0111174335847037));
#13931=CARTESIAN_POINT('Ctrl Pts',(0.00300723758665274,-0.0226595892781931,
-0.0115466031829495));
#13932=CARTESIAN_POINT('Ctrl Pts',(0.00305043961649606,-0.0226490015665708,
-0.011754078895245));
#13933=CARTESIAN_POINT('Ctrl Pts',(0.00307226150597443,-0.022637922840801,
-0.0119653371521074));
#13934=CARTESIAN_POINT('Ctrl Pts',(0.00307261119196602,-0.0226264261836896,
-0.0121759442462848));
#13935=CARTESIAN_POINT('',(0.00307349983335769,-0.0216248189898234,-0.0121765573521433));
#13936=CARTESIAN_POINT('Ctrl Pts',(0.00307349929150754,-0.0226247811395518,
-0.0121779401748277));
#13937=CARTESIAN_POINT('Ctrl Pts',(0.00307311430164888,-0.0225954191960958,
-0.0127449403707989));
#13938=CARTESIAN_POINT('Ctrl Pts',(0.00291152735071005,-0.0225660572526398,
-0.013311969538757));
#13939=CARTESIAN_POINT('Ctrl Pts',(0.00261308932736971,-0.0225366953091838,
-0.013793928197428));
#13940=CARTESIAN_POINT('Ctrl Pts',(0.0024880548265633,-0.0225243937401624,
-0.0139958510610824));
#13941=CARTESIAN_POINT('Ctrl Pts',(0.00233962293493056,-0.0225120921711411,
-0.0141830137117398));
#13942=CARTESIAN_POINT('Ctrl Pts',(0.00217200314735264,-0.0224997906021197,
-0.0143504347584488));
#13943=CARTESIAN_POINT('Ctrl Pts',(0.00177929151526496,-0.0224709696059985,
-0.0147426807662081));
#13944=CARTESIAN_POINT('Ctrl Pts',(0.0012756988519483,-0.0224421486098772,
-0.0150270336580492));
#13945=CARTESIAN_POINT('Ctrl Pts',(0.000734866705221547,-0.022413327613756,
-0.0151602080200904));
#13946=CARTESIAN_POINT('Ctrl Pts',(0.000493874143373817,-0.0224004850973999,
-0.0152195499635659));
#13947=CARTESIAN_POINT('Ctrl Pts',(0.000245874960503312,-0.0223876425810437,
-0.0152494784326798));
#13948=CARTESIAN_POINT('Ctrl Pts',(-1.5594132469024E-6,-0.0223748000646876,
-0.0152493528909554));
#13949=CARTESIAN_POINT('Ctrl Pts',(-0.000558901941837568,-0.0223458724729755,
-0.0152490701099455));
#13950=CARTESIAN_POINT('Ctrl Pts',(-0.0011180148393364,-0.0223169448812633,
-0.0150928521766949));
#13951=CARTESIAN_POINT('Ctrl Pts',(-0.00159573531068977,-0.0222880172895512,
-0.0148026443075984));
#13952=CARTESIAN_POINT('Ctrl Pts',(-0.00180606080655659,-0.022275281368786,
-0.0146748747904176));
#13953=CARTESIAN_POINT('Ctrl Pts',(-0.00200076576455277,-0.0222625454480207,
-0.0145218188158553));
#13954=CARTESIAN_POINT('Ctrl Pts',(-0.0021742086799485,-0.0222498095272555,
-0.0143482296043347));
#13955=CARTESIAN_POINT('Ctrl Pts',(-0.00256808227296006,-0.0222208873723167,
-0.0139540237857016));
#13956=CARTESIAN_POINT('Ctrl Pts',(-0.0028529831357351,-0.0221919652173779,
-0.0134483316010587));
#13957=CARTESIAN_POINT('Ctrl Pts',(-0.00298564563878129,-0.0221630430624391,
-0.0129054575420462));
#13958=CARTESIAN_POINT('Ctrl Pts',(-0.00304408873843441,-0.0221503017049005,
-0.0126662999654782));
#13959=CARTESIAN_POINT('Ctrl Pts',(-0.00307358224738798,-0.022137560347362,
-0.0124203009577403));
#13960=CARTESIAN_POINT('Ctrl Pts',(-0.0030734998267616,-0.0221248189898234,
-0.0121748213483798));
#13961=CARTESIAN_POINT('Ctrl Pts',(-0.0030733127366404,-0.0220958968348846,
-0.0116175966354908));
#13962=CARTESIAN_POINT('Ctrl Pts',(-0.00291725456535694,-0.0220669746799457,
-0.0110585559437886));
#13963=CARTESIAN_POINT('Ctrl Pts',(-0.00262723032005655,-0.0220380525250069,
-0.0105808413444788));
#13964=CARTESIAN_POINT('Ctrl Pts',(-0.00249946312525238,-0.0220253111674683,
-0.0103703890969173));
#13965=CARTESIAN_POINT('Ctrl Pts',(-0.00234638295676836,-0.0220125698099298,
-0.0101755642197633));
#13966=CARTESIAN_POINT('Ctrl Pts',(-0.00217274942421638,-0.0219998284523912,
-0.0100020174625899));
#13967=CARTESIAN_POINT('Ctrl Pts',(-0.00177853711818865,-0.0219709008606791,
-0.00960800216874991));
#13968=CARTESIAN_POINT('Ctrl Pts',(-0.00127278554717199,-0.0219419732689669,
-0.00932298654933162));
#13969=CARTESIAN_POINT('Ctrl Pts',(-0.000729818611945095,-0.0219130456772548,
-0.00919026003836461));
#13970=CARTESIAN_POINT('Ctrl Pts',(-0.000490767123179356,-0.0219003097564896,
-0.00913182467520187));
#13971=CARTESIAN_POINT('Ctrl Pts',(-0.000244876181528169,-0.0218875738357243,
-0.00910231305287151));
#13972=CARTESIAN_POINT('Ctrl Pts',(5.04463079185754E-7,-0.0218748379149591,
-0.00910235332795764));
#13973=CARTESIAN_POINT('Ctrl Pts',(0.000555793298242175,-0.0218460169188379,
-0.00910244446923611));
#13974=CARTESIAN_POINT('Ctrl Pts',(0.00111307090434215,-0.0218171959227166,
-0.00925735919509966));
#13975=CARTESIAN_POINT('Ctrl Pts',(0.00158968958608715,-0.0217883749265954,
-0.0095453990919586));
#13976=CARTESIAN_POINT('Ctrl Pts',(0.00180206889422062,-0.0217755324102393,
-0.00967374847554921));
#13977=CARTESIAN_POINT('Ctrl Pts',(0.00199858963676925,-0.0217626898938831,
-0.00982783015738682));
#13978=CARTESIAN_POINT('Ctrl Pts',(0.00217346290396063,-0.021749847377527,
-0.010002730819897));
#13979=CARTESIAN_POINT('Ctrl Pts',(0.00257327699341549,-0.021720485434071,
-0.0104026075434791));
#13980=CARTESIAN_POINT('Ctrl Pts',(0.00286066137097504,-0.0216911234906151,
-0.0109168534823359));
#13981=CARTESIAN_POINT('Ctrl Pts',(0.00299114972208898,-0.0216617615471591,
-0.0114691527912653));
#13982=CARTESIAN_POINT('Ctrl Pts',(0.0030458195180486,-0.0216494599781377,
-0.0117005457874222));
#13983=CARTESIAN_POINT('Ctrl Pts',(0.00307349822130347,-0.0216371584091163,
-0.0119382780953225));
#13984=CARTESIAN_POINT('Ctrl Pts',(0.00307349999991385,-0.0216248568400949,
-0.0121758302745233));
#13985=CARTESIAN_POINT('',(0.0030734993528554,-0.0206247116996209,-0.0121744194201276));
#13986=CARTESIAN_POINT('Ctrl Pts',(0.00307349966680153,-0.0216247811395518,
-0.0121772844297633));
#13987=CARTESIAN_POINT('Ctrl Pts',(0.0030732356479493,-0.0215954136692731,
-0.0127442869850705));
#13988=CARTESIAN_POINT('Ctrl Pts',(0.00291176844050567,-0.0215660461989944,
-0.0133113525384645));
#13989=CARTESIAN_POINT('Ctrl Pts',(0.00261343117209257,-0.0215366787287157,
-0.0137933760093459));
#13990=CARTESIAN_POINT('Ctrl Pts',(0.00248848650987813,-0.0215243795323277,
-0.0139952490775987));
#13991=CARTESIAN_POINT('Ctrl Pts',(0.00234015906022308,-0.0215120803359398,
-0.014182378104514));
#13992=CARTESIAN_POINT('Ctrl Pts',(0.002172652235586,-0.0214997811395518,
-0.0143497862462427));
#13993=CARTESIAN_POINT('Ctrl Pts',(0.00178005414938768,-0.021470954606817,
-0.0147421530420382));
#13994=CARTESIAN_POINT('Ctrl Pts',(0.00127654165317278,-0.0214421280740823,
-0.0150266571933579));
#13995=CARTESIAN_POINT('Ctrl Pts',(0.000735744851787406,-0.0214133015413475,
-0.0151599916484757));
#13996=CARTESIAN_POINT('Ctrl Pts',(0.000494859018460462,-0.0214004614074156,
-0.0152193824977743));
#13997=CARTESIAN_POINT('Ctrl Pts',(0.000246963129670334,-0.0213876212734837,
-0.0152493838499329));
#13998=CARTESIAN_POINT('Ctrl Pts',(-3.80074158312444E-7,-0.0213747811395518,
-0.0152493532630578));
#13999=CARTESIAN_POINT('Ctrl Pts',(-0.000557727405901423,-0.0213458480042346,
-0.0152492843405526));
#14000=CARTESIAN_POINT('Ctrl Pts',(-0.00111690398182406,-0.0213169148689173,
-0.0150932784200768));
#14001=CARTESIAN_POINT('Ctrl Pts',(-0.00159473782610428,-0.0212879817336001,
-0.0148032500049834));
#14002=CARTESIAN_POINT('Ctrl Pts',(-0.00180503346704472,-0.0212752482022506,
-0.0146756079131285));
#14003=CARTESIAN_POINT('Ctrl Pts',(-0.00199972987390663,-0.0212625146709012,
-0.0145226923737388));
#14004=CARTESIAN_POINT('Ctrl Pts',(-0.00217318983351514,-0.0212497811395518,
-0.0143492488321288));
#14005=CARTESIAN_POINT('Ctrl Pts',(-0.00256725147934152,-0.0212208534473509,
-0.0139552244842675));
#14006=CARTESIAN_POINT('Ctrl Pts',(-0.00285239027995229,-0.02119192575515,
-0.013449661601223));
#14007=CARTESIAN_POINT('Ctrl Pts',(-0.00298530606556781,-0.0211629980629491,
-0.0129068457248801));
#14008=CARTESIAN_POINT('Ctrl Pts',(-0.00304383858822103,-0.0211502590884833,
-0.0126678042714409));
#14009=CARTESIAN_POINT('Ctrl Pts',(-0.00307344635440524,-0.0211375201140176,
-0.0124219130413494));
#14010=CARTESIAN_POINT('Ctrl Pts',(-0.00307349992675546,-0.0211247811395518,
-0.012176524281491));
#14011=CARTESIAN_POINT('Ctrl Pts',(-0.00307362157897022,-0.0210958534473509,
-0.0116192949272901));
#14012=CARTESIAN_POINT('Ctrl Pts',(-0.00291787070471117,-0.02106692575515,
-0.0110601641731118));
#14013=CARTESIAN_POINT('Ctrl Pts',(-0.00262810741779381,-0.0210379980629491,
-0.0105822869557965));
#14014=CARTESIAN_POINT('Ctrl Pts',(-0.00250050349116459,-0.0210252590884833,
-0.0103718427341533));
#14015=CARTESIAN_POINT('Ctrl Pts',(-0.00234759692874837,-0.0210125201140176,
-0.0101770002697919));
#14016=CARTESIAN_POINT('Ctrl Pts',(-0.00217413860137922,-0.0209997811395518,
-0.0100034068333646));
#14017=CARTESIAN_POINT('Ctrl Pts',(-0.00178017492155852,-0.0209708480042346,
-0.00960913628985804));
#14018=CARTESIAN_POINT('Ctrl Pts',(-0.00127460120093978,-0.0209419148689173,
-0.00932379654364457));
#14019=CARTESIAN_POINT('Ctrl Pts',(-0.0007317150245235,-0.0209129817336001,
-0.00919072424866265));
#14020=CARTESIAN_POINT('Ctrl Pts',(-0.000492789720688787,-0.0209002482022506,
-0.00913215886259882));
#14021=CARTESIAN_POINT('Ctrl Pts',(-0.000247011714850828,-0.0208875146709012,
-0.0091024912033574));
#14022=CARTESIAN_POINT('Ctrl Pts',(-1.72206394589758E-6,-0.0208747811395518,
-0.00910235376898928));
#14023=CARTESIAN_POINT('Ctrl Pts',(0.000553571668584063,-0.020845954606817,
-0.009102042641133));
#14024=CARTESIAN_POINT('Ctrl Pts',(0.00111096533262494,-0.0208171280740823,
-0.0092565562732921));
#14025=CARTESIAN_POINT('Ctrl Pts',(0.00158779473491439,-0.0207883015413475,
-0.00954425488828792));
#14026=CARTESIAN_POINT('Ctrl Pts',(0.00180018772176464,-0.0207754614074156,
-0.00967240379827177));
#14027=CARTESIAN_POINT('Ctrl Pts',(0.00199675249277233,-0.0207626212734837,
-0.00982627724709428));
#14028=CARTESIAN_POINT('Ctrl Pts',(0.00217170281880654,-0.0207497811395518,
-0.0100009718836334));
#14029=CARTESIAN_POINT('Ctrl Pts',(0.00257184260919384,-0.0207204136692731,
-0.0104005268706466));
#14030=CARTESIAN_POINT('Ctrl Pts',(0.00285964364699999,-0.0206910461989944,
-0.0109145426511768));
#14031=CARTESIAN_POINT('Ctrl Pts',(0.00299057826765684,-0.0206616787287157,
-0.0114667384333653));
#14032=CARTESIAN_POINT('Ctrl Pts',(0.00304541413190247,-0.0206493795323277,
-0.0116979999041451));
#14033=CARTESIAN_POINT('Ctrl Pts',(0.00307328449308178,-0.0206370803359398,
-0.0119356176270179));
#14034=CARTESIAN_POINT('Ctrl Pts',(0.00307349874893983,-0.0206247811395518,
-0.0121730801538007));
#14035=CARTESIAN_POINT('',(0.00307349999999997,-0.0196247725843239,-0.0121758528436125));
#14036=CARTESIAN_POINT('Ctrl Pts',(0.00307349999999974,-0.0206246372891225,
-0.0121758545522439));
#14037=CARTESIAN_POINT('Ctrl Pts',(0.00307349976650647,-0.0205952804094407,
-0.0127428527552078));
#14038=CARTESIAN_POINT('Ctrl Pts',(0.00291229877631606,-0.0205659235297588,
-0.0133099896588568));
#14039=CARTESIAN_POINT('Ctrl Pts',(0.00261418979853331,-0.020536566650077,
-0.01379214965395));
#14040=CARTESIAN_POINT('Ctrl Pts',(0.00248924902626763,-0.02052426285686,
-0.0139942282447748));
#14041=CARTESIAN_POINT('Ctrl Pts',(0.00234088438044462,-0.0205119590636431,
-0.0141815521404052));
#14042=CARTESIAN_POINT('Ctrl Pts',(0.00217330663059751,-0.0204996552704261,
-0.0143491320398249));
#14043=CARTESIAN_POINT('Ctrl Pts',(0.00178083356867207,-0.0204708393482553,
-0.0147416101361259));
#14044=CARTESIAN_POINT('Ctrl Pts',(0.00127741589242395,-0.0204420234260845,
-0.0150262640632941));
#14045=CARTESIAN_POINT('Ctrl Pts',(0.000736667807712326,-0.0204132075039136,
-0.0151597639405624));
#14046=CARTESIAN_POINT('Ctrl Pts',(0.00049562834648803,-0.0204003627531857,
-0.015219271758343));
#14047=CARTESIAN_POINT('Ctrl Pts',(0.000247559663784795,-0.0203875180024577,
-0.0152493500093755));
#14048=CARTESIAN_POINT('Ctrl Pts',(4.06901849174428E-8,-0.0203746732517298,
-0.0152493532862887));
#14049=CARTESIAN_POINT('Ctrl Pts',(-0.000557297518273502,-0.0203457507402363,
-0.0152493606649108));
#14050=CARTESIAN_POINT('Ctrl Pts',(-0.00111648816619293,-0.0203168282287427,
-0.015093436186547));
#14051=CARTESIAN_POINT('Ctrl Pts',(-0.00159435775550837,-0.0202879057172492,
-0.0148034806569153));
#14052=CARTESIAN_POINT('Ctrl Pts',(-0.00180482287921371,-0.020275167555844,
-0.0146757773508723));
#14053=CARTESIAN_POINT('Ctrl Pts',(-0.00199966987372288,-0.0202624293944387,
-0.0145227618305072));
#14054=CARTESIAN_POINT('Ctrl Pts',(-0.00217324908559339,-0.0202496912330335,
-0.0143491895840435));
#14055=CARTESIAN_POINT('Ctrl Pts',(-0.00256729371252134,-0.0202207741524419,
-0.0139551607693842));
#14056=CARTESIAN_POINT('Ctrl Pts',(-0.00285241708289534,-0.0201918570718504,
-0.0134495984803389));
#14057=CARTESIAN_POINT('Ctrl Pts',(-0.0029853204821425,-0.0201629399912588,
-0.0129067868463982));
#14058=CARTESIAN_POINT('Ctrl Pts',(-0.00304389025134481,-0.0201501963989516,
-0.0126675728586422));
#14059=CARTESIAN_POINT('Ctrl Pts',(-0.00307349339570498,-0.0201374528066444,
-0.0124214998062665));
#14060=CARTESIAN_POINT('Ctrl Pts',(-0.00307349999888883,-0.0201247092143371,
-0.0121759359326137));
#14061=CARTESIAN_POINT('Ctrl Pts',(-0.00307351498248176,-0.0200957921337456,
-0.0116187154759645));
#14062=CARTESIAN_POINT('Ctrl Pts',(-0.00291766184917668,-0.020066875053154,
-0.0110596216408992));
#14063=CARTESIAN_POINT('Ctrl Pts',(-0.00262781436243296,-0.0200379579725625,
-0.0105818037495013));
#14064=CARTESIAN_POINT('Ctrl Pts',(-0.00250008022998325,-0.0200252143802553,
-0.0103712321329855));
#14065=CARTESIAN_POINT('Ctrl Pts',(-0.0023470098422513,-0.020012470787948,
-0.0101762894566337));
#14066=CARTESIAN_POINT('Ctrl Pts',(-0.00217336596396837,-0.0199997271956408,
-0.0100026338690432));
#14067=CARTESIAN_POINT('Ctrl Pts',(-0.00177926852704949,-0.0199708046841473,
-0.00960850985699746));
#14068=CARTESIAN_POINT('Ctrl Pts',(-0.00127360194940171,-0.0199418821726537,
-0.00932335160670282));
#14069=CARTESIAN_POINT('Ctrl Pts',(-0.000730676576994284,-0.0199129596611602,
-0.00919046989579705));
#14070=CARTESIAN_POINT('Ctrl Pts',(-0.000491559340364625,-0.019900221499755,
-0.0091319456323803));
#14071=CARTESIAN_POINT('Ctrl Pts',(-0.000245589593893761,-0.0198874833383497,
-0.00910236324041321));
#14072=CARTESIAN_POINT('Ctrl Pts',(-1.24601926384675E-7,-0.0198747451769445,
-0.00910235328908382));
#14073=CARTESIAN_POINT('Ctrl Pts',(0.000555159624672213,-0.0198459292547737,
-0.00910233077745721));
#14074=CARTESIAN_POINT('Ctrl Pts',(0.00111246523677488,-0.0198171133326028,
-0.00925712897680344));
#14075=CARTESIAN_POINT('Ctrl Pts',(0.00158914084161407,-0.019788297410432,
-0.00954506754166853));
#14076=CARTESIAN_POINT('Ctrl Pts',(0.00180161987615457,-0.019775452659704,
-0.00967341669075106));
#14077=CARTESIAN_POINT('Ctrl Pts',(0.00199823474569244,-0.0197626079089761,
-0.00982751922627757));
#14078=CARTESIAN_POINT('Ctrl Pts',(0.00217318974903144,-0.0197497631582481,
-0.0100024576565117));
#14079=CARTESIAN_POINT('Ctrl Pts',(0.00257305215909598,-0.0197204062785663,
-0.0104022821884846));
#14080=CARTESIAN_POINT('Ctrl Pts',(0.0028605007836907,-0.0196910493988845,
-0.0109164895181404));
#14081=CARTESIAN_POINT('Ctrl Pts',(0.0029910593252564,-0.0196616925192027,
-0.0114687702908661));
#14082=CARTESIAN_POINT('Ctrl Pts',(0.00304577785513911,-0.0196493887259857,
-0.0117002372757422));
#14083=CARTESIAN_POINT('Ctrl Pts',(0.00307348711766066,-0.0196370849327688,
-0.0119380515063182));
#14084=CARTESIAN_POINT('Ctrl Pts',(0.00307349999548699,-0.0196247811395518,
-0.012175686728761));
#14085=CARTESIAN_POINT('',(0.00307349937524521,-0.0186248572848198,-0.0121772131837633));
#14086=CARTESIAN_POINT('Ctrl Pts',(0.00307349999999997,-0.0196247725843239,
-0.0121758528436125));
#14087=CARTESIAN_POINT('Ctrl Pts',(0.00307350008171438,-0.0195954163064465,
-0.0127428507721285));
#14088=CARTESIAN_POINT('Ctrl Pts',(0.00291229955620968,-0.0195660600285692,
-0.013309987530298));
#14089=CARTESIAN_POINT('Ctrl Pts',(0.00261419109876588,-0.0195367037506918,
-0.0137921475509584));
#14090=CARTESIAN_POINT('Ctrl Pts',(0.00248924695606628,-0.0195243998563183,
-0.0139942319565535));
#14091=CARTESIAN_POINT('Ctrl Pts',(0.00234087759884723,-0.0195120959619448,
-0.0141815608434973));
#14092=CARTESIAN_POINT('Ctrl Pts',(0.00217329417145387,-0.0194997920675713,
-0.0143491444990569));
#14093=CARTESIAN_POINT('Ctrl Pts',(0.00178081915956632,-0.0194709767415835,
-0.0147416200453026));
#14094=CARTESIAN_POINT('Ctrl Pts',(0.00127740025025495,-0.0194421614155956,
-0.0150262710078965));
#14095=CARTESIAN_POINT('Ctrl Pts',(0.000736651773140311,-0.0194133460896077,
-0.0151597678991315));
#14096=CARTESIAN_POINT('Ctrl Pts',(0.000495604489924695,-0.0194005011971331,
-0.015219276273749));
#14097=CARTESIAN_POINT('Ctrl Pts',(0.000247527703741473,-0.0193876563046585,
-0.0152493532008676));
#14098=CARTESIAN_POINT('Ctrl Pts',(1.06400358957003E-9,-0.0193748114121839,
-0.0152493532865579));
#14099=CARTESIAN_POINT('Ctrl Pts',(-0.000557336746359336,-0.0193458894979458,
-0.0152493534795006));
#14100=CARTESIAN_POINT('Ctrl Pts',(-0.00111652506637318,-0.0193169675837076,
-0.0150934220048482));
#14101=CARTESIAN_POINT('Ctrl Pts',(-0.0015943907447657,-0.0192880456694695,
-0.014803460639837));
#14102=CARTESIAN_POINT('Ctrl Pts',(-0.00180486085195263,-0.0192753073652451,
-0.0146757506946925));
#14103=CARTESIAN_POINT('Ctrl Pts',(-0.00199971152818518,-0.0192625690610208,
-0.0145227271382931));
#14104=CARTESIAN_POINT('Ctrl Pts',(-0.00217329266672608,-0.0192498307567964,
-0.0143491460037857));
#14105=CARTESIAN_POINT('Ctrl Pts',(-0.00256732911840163,-0.0192209142729023,
-0.0139551095612665));
#14106=CARTESIAN_POINT('Ctrl Pts',(-0.00285244227892529,-0.0191919977890082,
-0.0134495419197709));
#14107=CARTESIAN_POINT('Ctrl Pts',(-0.00298533489846075,-0.0191630813051141,
-0.0129067279639361));
#14108=CARTESIAN_POINT('Ctrl Pts',(-0.00304390177940186,-0.0191503375705457,
-0.0126675053461888));
#14109=CARTESIAN_POINT('Ctrl Pts',(-0.0030735000793069,-0.0191375938359773,
-0.0124214238050535));
#14110=CARTESIAN_POINT('Ctrl Pts',(-0.00307349999999984,-0.0191248501014089,
-0.0121758522939746));
#14111=CARTESIAN_POINT('Ctrl Pts',(-0.00307349982004621,-0.0190959336175149,
-0.0116186322258037));
#14112=CARTESIAN_POINT('Ctrl Pts',(-0.00291763168036504,-0.0190670171336208,
-0.0110595429415768));
#14113=CARTESIAN_POINT('Ctrl Pts',(-0.00262777150819455,-0.0190381006497267,
-0.0105817331057935));
#14114=CARTESIAN_POINT('Ctrl Pts',(-0.00250002772338218,-0.0190253569151583,
-0.0103711583435332));
#14115=CARTESIAN_POINT('Ctrl Pts',(-0.00234694651141168,-0.0190126131805899,
-0.0101762141856548));
#14116=CARTESIAN_POINT('Ctrl Pts',(-0.00217329126300049,-0.0189998694460215,
-0.0100025591656058));
#14117=CARTESIAN_POINT('Ctrl Pts',(-0.00177918055906308,-0.0189709475317834,
-0.00960844897993668));
#14118=CARTESIAN_POINT('Ctrl Pts',(-0.00127350455405528,-0.0189420256175452,
-0.00932330818517744));
#14119=CARTESIAN_POINT('Ctrl Pts',(-0.000730574967265789,-0.0189131037033071,
-0.00919044502851287));
#14120=CARTESIAN_POINT('Ctrl Pts',(-0.000491448255527693,-0.0189003653990827,
-0.00913192707234067));
#14121=CARTESIAN_POINT('Ctrl Pts',(-0.000245469588832847,-0.0188876270948584,
-0.00910235304303009));
#14122=CARTESIAN_POINT('Ctrl Pts',(3.04917062178946E-9,-0.018874888790634,
-0.00910235328655961));
#14123=CARTESIAN_POINT('Ctrl Pts',(0.000555286857799042,-0.0188460734646461,
-0.00910235383744787));
#14124=CARTESIAN_POINT('Ctrl Pts',(0.00111258570577606,-0.0188172581386582,
-0.00925717495982157));
#14125=CARTESIAN_POINT('Ctrl Pts',(0.00158924916809846,-0.0187884428126704,
-0.00954513297993134));
#14126=CARTESIAN_POINT('Ctrl Pts',(0.00180172953089864,-0.0187755979201957,
-0.00967349487342752));
#14127=CARTESIAN_POINT('Ctrl Pts',(0.00199834367379624,-0.0187627530277211,
-0.00982761111220334));
#14128=CARTESIAN_POINT('Ctrl Pts',(0.00217329557517749,-0.0187499081352465,
-0.0100025634777857));
#14129=CARTESIAN_POINT('Ctrl Pts',(0.0025731383406563,-0.018720551853384,
-0.0104024073041701));
#14130=CARTESIAN_POINT('Ctrl Pts',(0.00286056189175292,-0.0186911955715216,
-0.0109166284047005));
#14131=CARTESIAN_POINT('Ctrl Pts',(0.00299109361119617,-0.0186618392896591,
-0.0114689153408645));
#14132=CARTESIAN_POINT('Ctrl Pts',(0.0030458026512524,-0.0186495353530591,
-0.0117003923201153));
#14133=CARTESIAN_POINT('Ctrl Pts',(0.0030735003947725,-0.0186372314164591,
-0.0119382156415932));
#14134=CARTESIAN_POINT('Ctrl Pts',(0.00307349999999576,-0.0186249274798591,
-0.0121758583923158));
#14135=CARTESIAN_POINT('',(0.00307349990129765,-0.017624751935175,-0.0121753126773873));
#14136=CARTESIAN_POINT('Ctrl Pts',(0.00307349869753639,-0.0186247811395518,
-0.0121786828169311));
#14137=CARTESIAN_POINT('Ctrl Pts',(0.00307297670297644,-0.018595414100554,
-0.0127456848945252));
#14138=CARTESIAN_POINT('Ctrl Pts',(0.00291125166932543,-0.0185660470615561,
-0.0133126766736151));
#14139=CARTESIAN_POINT('Ctrl Pts',(0.00261269539128645,-0.0185366800225583,
-0.0137945642065035));
#14140=CARTESIAN_POINT('Ctrl Pts',(0.00248765278626428,-0.0185243803948895,
-0.0139963903842542));
#14141=CARTESIAN_POINT('Ctrl Pts',(0.00233923178850257,-0.0185120807672206,
-0.014183460423467));
#14142=CARTESIAN_POINT('Ctrl Pts',(0.00217163872964959,-0.0184997811395518,
-0.0143507986830878));
#14143=CARTESIAN_POINT('Ctrl Pts',(0.00177885827015184,-0.0184709550447214,
-0.0147429819808644));
#14144=CARTESIAN_POINT('Ctrl Pts',(0.00127521384053096,-0.0184421289498909,
-0.0150272512926739));
#14145=CARTESIAN_POINT('Ctrl Pts',(0.000734355529584412,-0.0184133028550605,
-0.0151603338454106));
#14146=CARTESIAN_POINT('Ctrl Pts',(0.000493430422115672,-0.0184004622832242,
-0.015219615412637));
#14147=CARTESIAN_POINT('Ctrl Pts',(0.000245508262046727,-0.018387621711388,
-0.0152495013622853));
#14148=CARTESIAN_POINT('Ctrl Pts',(-1.84680271542727E-6,-0.0183747811395518,
-0.0152493527317052));
#14149=CARTESIAN_POINT('Ctrl Pts',(-0.000559193420020552,-0.0183458484419979,
-0.0152490178335656));
#14150=CARTESIAN_POINT('Ctrl Pts',(-0.0011182949906921,-0.0183169157444441,
-0.0150927454132629));
#14151=CARTESIAN_POINT('Ctrl Pts',(-0.0015959901063058,-0.0182879830468902,
-0.0148024895062455));
#14152=CARTESIAN_POINT('Ctrl Pts',(-0.00180623510113311,-0.0182752490777774,
-0.014674740970255));
#14153=CARTESIAN_POINT('Ctrl Pts',(-0.00200086728772786,-0.0182625151086646,
-0.0145217239548106));
#14154=CARTESIAN_POINT('Ctrl Pts',(-0.00217425092061059,-0.0182497811395518,
-0.0143481873272213));
#14155=CARTESIAN_POINT('Ctrl Pts',(-0.00256811967853617,-0.0182208538843402,
-0.0139539710172573));
#14156=CARTESIAN_POINT('Ctrl Pts',(-0.00285301144956077,-0.0181919266291286,
-0.0134482695177798));
#14157=CARTESIAN_POINT('Ctrl Pts',(-0.00298566230667035,-0.0181629993739169,
-0.0129053893312659));
#14158=CARTESIAN_POINT('Ctrl Pts',(-0.00304408104831109,-0.0181502599624619,
-0.0126663077448451));
#14159=CARTESIAN_POINT('Ctrl Pts',(-0.00307356886975759,-0.0181375205510068,
-0.0124203898267037));
#14160=CARTESIAN_POINT('Ctrl Pts',(-0.00307349987853825,-0.0181247811395518,
-0.0121749892116891));
#14161=CARTESIAN_POINT('Ctrl Pts',(-0.00307334322086089,-0.0180958538843402,
-0.0116177604696338));
#14162=CARTESIAN_POINT('Ctrl Pts',(-0.00291731342951439,-0.0180669266291286,
-0.0110587080557867));
#14163=CARTESIAN_POINT('Ctrl Pts',(-0.00262731199399766,-0.0180379993739169,
-0.0105809758818037));
#14164=CARTESIAN_POINT('Ctrl Pts',(-0.00249959688302106,-0.0180252599624619,
-0.0103705851383627));
#14165=CARTESIAN_POINT('Ctrl Pts',(-0.00234658445395589,-0.0180125205510068,
-0.0101758103009194));
#14166=CARTESIAN_POINT('Ctrl Pts',(-0.00217302912958789,-0.0179997811395518,
-0.0100022970641515));
#14167=CARTESIAN_POINT('Ctrl Pts',(-0.00177886463254465,-0.0179708484419979,
-0.00960822815298435));
#14168=CARTESIAN_POINT('Ctrl Pts',(-0.00127314587228529,-0.017941915744444,
-0.00932314669040304));
#14169=CARTESIAN_POINT('Ctrl Pts',(-0.000730192371507065,-0.0179129830468902,
-0.00919035142747428));
#14170=CARTESIAN_POINT('Ctrl Pts',(-0.000491225607494931,-0.0179002490777774,
-0.00913190507025817));
#14171=CARTESIAN_POINT('Ctrl Pts',(-0.000245420214478279,-0.0178875151086646,
-0.00910236275876294));
#14172=CARTESIAN_POINT('Ctrl Pts',(-1.18653065741516E-7,-0.0178747811395518,
-0.00910235328884841));
#14173=CARTESIAN_POINT('Ctrl Pts',(0.000555174516620966,-0.0178459550447214,
-0.00910233185164749));
#14174=CARTESIAN_POINT('Ctrl Pts',(0.00111248697751199,-0.0178171289498909,
-0.00925713590221569));
#14175=CARTESIAN_POINT('Ctrl Pts',(0.00158916594125725,-0.0177883028550605,
-0.00954508270341179));
#14176=CARTESIAN_POINT('Ctrl Pts',(0.00180150238546827,-0.0177754622832242,
-0.00967334848507651));
#14177=CARTESIAN_POINT('Ctrl Pts',(0.00199799566702671,-0.017762621711388,
-0.00982733305485337));
#14178=CARTESIAN_POINT('Ctrl Pts',(0.00217286130198874,-0.0177497811395518,
-0.0100021292902053));
#14179=CARTESIAN_POINT('Ctrl Pts',(0.00257278787744105,-0.017720414100554,
-0.0104018971452298));
#14180=CARTESIAN_POINT('Ctrl Pts',(0.00286031494897729,-0.0176910470615562,
-0.0109160658455345));
#14181=CARTESIAN_POINT('Ctrl Pts',(0.0029909554462368,-0.0176616800225583,
-0.0114683310122611));
#14182=CARTESIAN_POINT('Ctrl Pts',(0.00304567085267882,-0.0176493803948895,
-0.0116996330487283));
#14183=CARTESIAN_POINT('Ctrl Pts',(0.00307341470433931,-0.0176370807672207,
-0.0119372776082813));
#14184=CARTESIAN_POINT('Ctrl Pts',(0.00307349980266144,-0.0176247811395518,
-0.0121747519055697));
#14185=CARTESIAN_POINT('',(0.00307349956938691,-0.0166247219214524,-0.0121746998012189));
#14186=CARTESIAN_POINT('Ctrl Pts',(0.00307349999993387,-0.0176247227307983,
-0.0121758734492049));
#14187=CARTESIAN_POINT('Ctrl Pts',(0.0030734962803204,-0.017595359946596,
-0.0127428740067176));
#14188=CARTESIAN_POINT('Ctrl Pts',(0.0029122905308065,-0.0175659971623937,
-0.0133100118969287));
#14189=CARTESIAN_POINT('Ctrl Pts',(0.00261417645067601,-0.0175366343781914,
-0.0137921712425095));
#14190=CARTESIAN_POINT('Ctrl Pts',(0.00248928246725899,-0.0175243329294251,
-0.0139941704278045));
#14191=CARTESIAN_POINT('Ctrl Pts',(0.00234098296327957,-0.0175120314806588,
-0.0141814262629012));
#14192=CARTESIAN_POINT('Ctrl Pts',(0.00217348357710258,-0.0174997300318925,
-0.0143489550766419));
#14193=CARTESIAN_POINT('Ctrl Pts',(0.00178103880370149,-0.017470908199265,
-0.0147414687977199));
#14194=CARTESIAN_POINT('Ctrl Pts',(0.00127763942897038,-0.0174420863666376,
-0.015026164674513));
#14195=CARTESIAN_POINT('Ctrl Pts',(0.000736897654871983,-0.0174132645340101,
-0.0151597071865076));
#14196=CARTESIAN_POINT('Ctrl Pts',(0.000495954532555534,-0.017400422133669,
-0.0152192109114707));
#14197=CARTESIAN_POINT('Ctrl Pts',(0.000247985299515979,-0.0173875797333278,
-0.0152493081466551));
#14198=CARTESIAN_POINT('Ctrl Pts',(5.6009102431774E-7,-0.0173747373329867,
-0.0152493532355248));
#14199=CARTESIAN_POINT('Ctrl Pts',(-0.000556782977434645,-0.0173458089030335,
-0.0152494548014448));
#14200=CARTESIAN_POINT('Ctrl Pts',(-0.00111600385162446,-0.0173168804730803,
-0.0150936222173342));
#14201=CARTESIAN_POINT('Ctrl Pts',(-0.00159392454543696,-0.0172879520431271,
-0.0148037434656663));
#14202=CARTESIAN_POINT('Ctrl Pts',(-0.00180433015069223,-0.0172752162401117,
-0.0146761237266909));
#14203=CARTESIAN_POINT('Ctrl Pts',(-0.00199913382837564,-0.0172624804370963,
-0.0145232086804128));
#14204=CARTESIAN_POINT('Ctrl Pts',(-0.0021726914140132,-0.0172497446340809,
-0.014349747090191));
#14205=CARTESIAN_POINT('Ctrl Pts',(-0.00256684047077401,-0.017220821641593,
-0.0139558160388974));
#14206=CARTESIAN_POINT('Ctrl Pts',(-0.00285209442065788,-0.017191898649105,
-0.0134503224554305));
#14207=CARTESIAN_POINT('Ctrl Pts',(-0.00298513579568746,-0.0171629756566171,
-0.0129075407412171));
#14208=CARTESIAN_POINT('Ctrl Pts',(-0.00304374356782033,-0.0171502344161364,
-0.0126684329672826));
#14209=CARTESIAN_POINT('Ctrl Pts',(-0.00307340871282563,-0.0171374931756557,
-0.0124224640790486));
#14210=CARTESIAN_POINT('Ctrl Pts',(-0.00307349978845192,-0.017124751935175,
-0.0121769936312336));
#14211=CARTESIAN_POINT('Ctrl Pts',(-0.00307370653281557,-0.0170958289426871,
-0.0116197684592478));
#14212=CARTESIAN_POINT('Ctrl Pts',(-0.00291804326889372,-0.0170669059501992,
-0.0110606172375488));
#14213=CARTESIAN_POINT('Ctrl Pts',(-0.00262835635395399,-0.0170379829577112,
-0.010582697573318));
#14214=CARTESIAN_POINT('Ctrl Pts',(-0.00250074263456118,-0.0170252417172306,
-0.0103721630176369));
#14215=CARTESIAN_POINT('Ctrl Pts',(-0.00234780681771066,-0.0170125004767499,
-0.0101772367700652));
#14216=CARTESIAN_POINT('Ctrl Pts',(-0.00217430395267995,-0.0169997592362692,
-0.0100035723260559));
#14217=CARTESIAN_POINT('Ctrl Pts',(-0.00178037327651628,-0.016970830806316,
-0.00960927479187941));
#14218=CARTESIAN_POINT('Ctrl Pts',(-0.00127482527644342,-0.0169419023763628,
-0.00932389735964255));
#14219=CARTESIAN_POINT('Ctrl Pts',(-0.000731953004829246,-0.0169129739464096,
-0.00919078259246701));
#14220=CARTESIAN_POINT('Ctrl Pts',(-0.000492952328850823,-0.0169002381433942,
-0.00913217853217292));
#14221=CARTESIAN_POINT('Ctrl Pts',(-0.000247092039078856,-0.0168875023403788,
-0.00910249113135262));
#14222=CARTESIAN_POINT('Ctrl Pts',(-1.72059828612464E-6,-0.0168747665373634,
-0.00910235376816842));
#14223=CARTESIAN_POINT('Ctrl Pts',(0.000553568659056523,-0.0168459447047359,
-0.00910204290762045));
#14224=CARTESIAN_POINT('Ctrl Pts',(0.00111095867085604,-0.0168171228721085,
-0.00925655441912994));
#14225=CARTESIAN_POINT('Ctrl Pts',(0.00158778597419169,-0.016788301039481,
-0.00954424960245972));
#14226=CARTESIAN_POINT('Ctrl Pts',(0.00180025015723536,-0.0167754586391399,
-0.00967244050441554));
#14227=CARTESIAN_POINT('Ctrl Pts',(0.0019968755877652,-0.0167626162387987,
-0.0098263732388435));
#14228=CARTESIAN_POINT('Ctrl Pts',(0.00217187042956542,-0.0167497738384576,
-0.0100011392623289));
#14229=CARTESIAN_POINT('Ctrl Pts',(0.00257197754660007,-0.0167204110542553,
-0.0104007232105927));
#14230=CARTESIAN_POINT('Ctrl Pts',(0.00285973859300779,-0.016691048270053,
-0.0109147587619568));
#14231=CARTESIAN_POINT('Ctrl Pts',(0.00299063140450493,-0.0166616854858507,
-0.0114669625669201));
#14232=CARTESIAN_POINT('Ctrl Pts',(0.00304546854812922,-0.0166493840370844,
-0.0116983066645546));
#14233=CARTESIAN_POINT('Ctrl Pts',(0.0030733213116782,-0.0166370825883181,
-0.011936009349354));
#14234=CARTESIAN_POINT('Ctrl Pts',(0.00307349913877991,-0.0166247811395518,
-0.0121735524347227));
#14235=CARTESIAN_POINT('',(0.00307390633487226,-0.0156241056269589,-0.0121772501359052));
#14236=CARTESIAN_POINT('Ctrl Pts',(0.00307349999999391,-0.0166246627033529,
-0.0121758471677152));
#14237=CARTESIAN_POINT('Ctrl Pts',(0.00307350112877669,-0.0165953700180398,
-0.0127428357199062));
#14238=CARTESIAN_POINT('Ctrl Pts',(0.00291230682244614,-0.0165660689951853,
-0.0133099641739799));
#14239=CARTESIAN_POINT('Ctrl Pts',(0.002614208497438,-0.0165367543867582,
-0.0137921194100424));
#14240=CARTESIAN_POINT('Ctrl Pts',(0.00248926772237858,-0.0165244678705648,
-0.0139942032321872));
#14241=CARTESIAN_POINT('Ctrl Pts',(0.00234090209310256,-0.0165121789678393,
-0.0141815319419045));
#14242=CARTESIAN_POINT('Ctrl Pts',(0.00217332274698239,-0.0164998872921877,
-0.0143491159231138));
#14243=CARTESIAN_POINT('Ctrl Pts',(0.00178084467378571,-0.0164710996564333,
-0.0147416048518896));
#14244=CARTESIAN_POINT('Ctrl Pts',(0.00127741700944676,-0.0164422968107177,
-0.0150262660493983));
#14245=CARTESIAN_POINT('Ctrl Pts',(0.000736656043588142,-0.01641349364647,
-0.0151597668448645));
#14246=CARTESIAN_POINT('Ctrl Pts',(0.000495625379421995,-0.0164006553570093,
-0.0152192714826426));
#14247=CARTESIAN_POINT('Ctrl Pts',(0.000247565780935063,-0.0163878170042657,
-0.0152493488464267));
#14248=CARTESIAN_POINT('Ctrl Pts',(5.5129846927282E-8,-0.0163749799069125,
-0.0152493532860637));
#14249=CARTESIAN_POINT('Ctrl Pts',(-0.000557318558336918,-0.0163460718164288,
-0.0152493632837621));
#14250=CARTESIAN_POINT('Ctrl Pts',(-0.00111654073205856,-0.0163171700921992,
-0.0150934222221862));
#14251=CARTESIAN_POINT('Ctrl Pts',(-0.0015944298199754,-0.0162882195180373,
-0.0148034369292179));
#14252=CARTESIAN_POINT('Ctrl Pts',(-0.00180486528662487,-0.0162754713140344,
-0.0146757437217557));
#14253=CARTESIAN_POINT('Ctrl Pts',(-0.00199968605253971,-0.0162627136379023,
-0.0145227449648848));
#14254=CARTESIAN_POINT('Ctrl Pts',(-0.00217324478123971,-0.0162499417750734,
-0.0143491938882159));
#14255=CARTESIAN_POINT('Ctrl Pts',(-0.00256704881673858,-0.0162209624712921,
-0.0139554072151439));
#14256=CARTESIAN_POINT('Ctrl Pts',(-0.00285208114276245,-0.016191910129541,
-0.0134501990338245));
#14257=CARTESIAN_POINT('Ctrl Pts',(-0.0029850804100728,-0.0161629900239187,
-0.0129077666662688));
#14258=CARTESIAN_POINT('Ctrl Pts',(-0.00304381105415618,-0.0161502193037148,
-0.0126682360059692));
#14259=CARTESIAN_POINT('Ctrl Pts',(-0.0030734935682315,-0.0161374743693433,
-0.0124218235040799));
#14260=CARTESIAN_POINT('Ctrl Pts',(-0.00307349999894891,-0.0161247728966703,
-0.0121759336673099));
#14261=CARTESIAN_POINT('Ctrl Pts',(-0.00307351459136934,-0.0160959510378268,
-0.011617966701677));
#14262=CARTESIAN_POINT('Ctrl Pts',(-0.00291725659147299,-0.0160673529699291,
-0.0110582110209378));
#14263=CARTESIAN_POINT('Ctrl Pts',(-0.00262671455400442,-0.0160387229375742,
-0.0105799921078269));
#14264=CARTESIAN_POINT('Ctrl Pts',(-0.00249926631704068,-0.0160261641795383,
-0.0103702181353934));
#14265=CARTESIAN_POINT('Ctrl Pts',(-0.00234666050317676,-0.0160135992709085,
-0.0101759774061611));
#14266=CARTESIAN_POINT('Ctrl Pts',(-0.00217360002710924,-0.0160010066243327,
-0.0100028679731814));
#14267=CARTESIAN_POINT('Ctrl Pts',(-0.00177991703981202,-0.0159723605068909,
-0.00960907361728126));
#14268=CARTESIAN_POINT('Ctrl Pts',(-0.00127479307298006,-0.0159435708498243,
-0.00932397045489184));
#14269=CARTESIAN_POINT('Ctrl Pts',(-0.000732373258603867,-0.0159147081592691,
-0.00919088567197968));
#14270=CARTESIAN_POINT('Ctrl Pts',(-0.000492770773530023,-0.015901958675936,
-0.00913209828282809));
#14271=CARTESIAN_POINT('Ctrl Pts',(-0.000246268960427492,-0.0158891949419885,
-0.00910237570626738));
#14272=CARTESIAN_POINT('Ctrl Pts',(-2.79962873519633E-7,-0.0158764230344964,
-0.0091023532993089));
#14273=CARTESIAN_POINT('Ctrl Pts',(0.00055505745979561,-0.0158475895571469,
-0.00910230271402786));
#14274=CARTESIAN_POINT('Ctrl Pts',(0.00111241738463871,-0.0158187144223219,
-0.00925710145582043));
#14275=CARTESIAN_POINT('Ctrl Pts',(0.00158913524431839,-0.0157897785602021,
-0.0095450641605989));
#14276=CARTESIAN_POINT('Ctrl Pts',(0.00180162169350743,-0.0157768810392236,
-0.00967341717149378));
#14277=CARTESIAN_POINT('Ctrl Pts',(0.00199824333142999,-0.0157639714533495,
-0.00982752549781976));
#14278=CARTESIAN_POINT('Ctrl Pts',(0.00217320411947251,-0.0157510481138661,
-0.0100024720256865));
#14279=CARTESIAN_POINT('Ctrl Pts',(0.00257308049831668,-0.0157215115631165,
-0.0104023158126139));
#14280=CARTESIAN_POINT('Ctrl Pts',(0.00286053074137381,-0.015691903168991,
-0.0109165483225608));
#14281=CARTESIAN_POINT('Ctrl Pts',(0.00299107879379126,-0.0156622296518079,
-0.0114688526505384));
#14282=CARTESIAN_POINT('Ctrl Pts',(0.00304579761884114,-0.0156497920859822,
-0.011700349354911));
#14283=CARTESIAN_POINT('Ctrl Pts',(0.00307350041344759,-0.0156373430790635,
-0.0119381941485527));
#14284=CARTESIAN_POINT('Ctrl Pts',(0.00307349999999535,-0.0156248831259193,
-0.0121758586333623));
#14285=CARTESIAN_POINT('',(0.00307349980039059,-0.0146248225157206,-0.012176624660313));
#14286=CARTESIAN_POINT('Ctrl Pts',(0.00307349936069457,-0.0156247811395518,
-0.012177835661408));
#14287=CARTESIAN_POINT('Ctrl Pts',(0.00307313365158047,-0.0155954195670811,
-0.0127448357564998));
#14288=CARTESIAN_POINT('Ctrl Pts',(0.00291156604386341,-0.0155660579946104,
-0.0133118703234303));
#14289=CARTESIAN_POINT('Ctrl Pts',(0.00261314451277681,-0.0155366964221397,
-0.0137938390730669));
#14290=CARTESIAN_POINT('Ctrl Pts',(0.00248811455764909,-0.0155243947759578,
-0.0139957699824105));
#14291=CARTESIAN_POINT('Ctrl Pts',(0.00233968582882625,-0.0155120931297759,
-0.0141829409193754));
#14292=CARTESIAN_POINT('Ctrl Pts',(0.00217206790103134,-0.015499791483594,
-0.0143503700796202));
#14293=CARTESIAN_POINT('Ctrl Pts',(0.00177936812662347,-0.0154709708571608,
-0.0147426276043517));
#14294=CARTESIAN_POINT('Ctrl Pts',(0.00127578416642009,-0.0154421502307276,
-0.0150269954458057));
#14295=CARTESIAN_POINT('Ctrl Pts',(0.000734956205693867,-0.0154133296042945,
-0.0151601859800948));
#14296=CARTESIAN_POINT('Ctrl Pts',(0.000493960994275608,-0.0154004870120751,
-0.0152195362417322));
#14297=CARTESIAN_POINT('Ctrl Pts',(0.000245958020913104,-0.0153876444198556,
-0.0152494721514421));
#14298=CARTESIAN_POINT('Ctrl Pts',(-1.48088146134381E-6,-0.0153748018276362,
-0.0152493529297971));
#14299=CARTESIAN_POINT('Ctrl Pts',(-0.000558823182087959,-0.0153458746063105,
-0.0152490843897039));
#14300=CARTESIAN_POINT('Ctrl Pts',(-0.00111793988359,-0.0153169473849847,
-0.0150928808685131));
#14301=CARTESIAN_POINT('Ctrl Pts',(-0.00159566766821423,-0.015288020163659,
-0.0148026853981739));
#14302=CARTESIAN_POINT('Ctrl Pts',(-0.00180600034135376,-0.0152752841663321,
-0.0146749189358203));
#14303=CARTESIAN_POINT('Ctrl Pts',(-0.00200071254666846,-0.0152625481690053,
-0.0145218646740806));
#14304=CARTESIAN_POINT('Ctrl Pts',(-0.00217416235453008,-0.0152498121716784,
-0.0143482759678391));
#14305=CARTESIAN_POINT('Ctrl Pts',(-0.00256804419217434,-0.0152208903867933,
-0.0139540787101331));
#14306=CARTESIAN_POINT('Ctrl Pts',(-0.00285295579622096,-0.0151919686019082,
-0.0134483928164419));
#14307=CARTESIAN_POINT('Ctrl Pts',(-0.00298562993797293,-0.0151630468170231,
-0.0129055217890164));
#14308=CARTESIAN_POINT('Ctrl Pts',(-0.00304407926247028,-0.0151503053832556,
-0.0126663610571421));
#14309=CARTESIAN_POINT('Ctrl Pts',(-0.00307357806885326,-0.0151375639494881,
-0.0124203580177665));
#14310=CARTESIAN_POINT('Ctrl Pts',(-0.00307349984395625,-0.0151248225157206,
-0.0121748738985247));
#14311=CARTESIAN_POINT('Ctrl Pts',(-0.00307332228123565,-0.0150959007308355,
-0.0116176494119419));
#14312=CARTESIAN_POINT('Ctrl Pts',(-0.00291727379124065,-0.0150669789459504,
-0.011058606234676));
#14313=CARTESIAN_POINT('Ctrl Pts',(-0.00262725790115753,-0.0150380571610653,
-0.0105808867756854));
#14314=CARTESIAN_POINT('Ctrl Pts',(-0.00249949198803375,-0.0150253157272978,
-0.0103704284353599));
#14315=CARTESIAN_POINT('Ctrl Pts',(-0.00234641189170714,-0.0150125742935303,
-0.0101755976081592));
#14316=CARTESIAN_POINT('Ctrl Pts',(-0.0021727774036934,-0.0149998328597628,
-0.0100020454284438));
#14317=CARTESIAN_POINT('Ctrl Pts',(-0.00177857033436272,-0.0149709056384371,
-0.0096080252258667));
#14318=CARTESIAN_POINT('Ctrl Pts',(-0.00127282265264435,-0.0149419784171113,
-0.00932300314062889));
#14319=CARTESIAN_POINT('Ctrl Pts',(-0.000729857634045862,-0.0149130511957856,
-0.00919026957746116));
#14320=CARTESIAN_POINT('Ctrl Pts',(-0.000490802491224546,-0.0149003151984587,
-0.00913183000987696));
#14321=CARTESIAN_POINT('Ctrl Pts',(-0.000244907263889183,-0.0148875792011319,
-0.00910231516908718));
#14322=CARTESIAN_POINT('Ctrl Pts',(4.7789457918649E-7,-0.014874843203805,
-0.0091023533237117));
#14323=CARTESIAN_POINT('Ctrl Pts',(0.000555766483525987,-0.0148460225773718,
-0.00910243966482436));
#14324=CARTESIAN_POINT('Ctrl Pts',(0.00111304523135227,-0.0148172019509386,
-0.00925734944151976));
#14325=CARTESIAN_POINT('Ctrl Pts',(0.00158966629488911,-0.0147883813245055,
-0.00954538501628879));
#14326=CARTESIAN_POINT('Ctrl Pts',(0.00180205064317471,-0.014775538732286,
-0.00967373487849681));
#14327=CARTESIAN_POINT('Ctrl Pts',(0.00199857606672519,-0.0147626961400666,
-0.00982781813059075));
#14328=CARTESIAN_POINT('Ctrl Pts',(0.00217345330382419,-0.0147498535478472,
-0.0100027212182991));
#14329=CARTESIAN_POINT('Ctrl Pts',(0.00257326905619171,-0.0147204919753765,
-0.0104025960720167));
#14330=CARTESIAN_POINT('Ctrl Pts',(0.0028606556848834,-0.0146911304029058,
-0.0109168406083762));
#14331=CARTESIAN_POINT('Ctrl Pts',(0.00299114651727006,-0.0146617688304351,
-0.0114691392268259));
#14332=CARTESIAN_POINT('Ctrl Pts',(0.00304581838648291,-0.0146494671842532,
-0.0117005363087668));
#14333=CARTESIAN_POINT('Ctrl Pts',(0.00307349817590678,-0.0146371655380713,
-0.0119382730645528));
#14334=CARTESIAN_POINT('Ctrl Pts',(0.0030734999999094,-0.0146248638918894,
-0.0121758296876704));
#14335=CARTESIAN_POINT('',(0.00307349954753674,-0.0136246902846469,-0.0121748470396884));
#14336=CARTESIAN_POINT('Ctrl Pts',(0.00307349960087178,-0.0146247811395518,
-0.0121774196329556));
#14337=CARTESIAN_POINT('Ctrl Pts',(0.00307321063952067,-0.0145954134790752,
-0.0127444223079151));
#14338=CARTESIAN_POINT('Ctrl Pts',(0.00291171841574269,-0.0145660458185986,
-0.0133114808685064));
#14339=CARTESIAN_POINT('Ctrl Pts',(0.00261335982369163,-0.014536678158122,
-0.0137934912812635));
#14340=CARTESIAN_POINT('Ctrl Pts',(0.00248840897262105,-0.014524379151932,
-0.0139953544516346));
#14341=CARTESIAN_POINT('Ctrl Pts',(0.00234007700429877,-0.0145120801457419,
-0.0141824731954777));
#14342=CARTESIAN_POINT('Ctrl Pts',(0.002172567261298,-0.0144997811395518,
-0.0143498711671506));
#14343=CARTESIAN_POINT('Ctrl Pts',(0.00177995363344448,-0.0144709544136982,
-0.014742222822502));
#14344=CARTESIAN_POINT('Ctrl Pts',(0.00127642974412018,-0.0144421276878447,
-0.0150267073464758));
#14345=CARTESIAN_POINT('Ctrl Pts',(0.000735627476184249,-0.0144133009619911,
-0.0151600205851998));
#14346=CARTESIAN_POINT('Ctrl Pts',(0.000494744444681753,-0.014400461021178,
-0.015219400693212));
#14347=CARTESIAN_POINT('Ctrl Pts',(0.000246852814080745,-0.0143876210803649,
-0.0152493922895258));
#14348=CARTESIAN_POINT('Ctrl Pts',(-4.85139050949205E-7,-0.0143747811395518,
-0.0152493532482695));
#14349=CARTESIAN_POINT('Ctrl Pts',(-0.000557832740682571,-0.0143458478111779,
-0.0152492652732931));
#14350=CARTESIAN_POINT('Ctrl Pts',(-0.00111700420073623,-0.0143169144828041,
-0.0150932400919133));
#14351=CARTESIAN_POINT('Ctrl Pts',(-0.00159482824846356,-0.0142879811544302,
-0.0148031951196477));
#14352=CARTESIAN_POINT('Ctrl Pts',(-0.00180511498649533,-0.0142752478161374,
-0.0146755485279988));
#14353=CARTESIAN_POINT('Ctrl Pts',(-0.00199980229410829,-0.0142625144778446,
-0.0145226301155781));
#14354=CARTESIAN_POINT('Ctrl Pts',(-0.0021732534721906,-0.0142497811395518,
-0.0143491851976134));
#14355=CARTESIAN_POINT('Ctrl Pts',(-0.00256730376778178,-0.0142208532546356,
-0.0139551491238987));
#14356=CARTESIAN_POINT('Ctrl Pts',(-0.00285242781397656,-0.0141919253697195,
-0.0134495776419844));
#14357=CARTESIAN_POINT('Ctrl Pts',(-0.00298532763319761,-0.0141629974848033,
-0.012906757639033));
#14358=CARTESIAN_POINT('Ctrl Pts',(-0.0030438518494217,-0.0141502587030528,
-0.0126677195770576));
#14359=CARTESIAN_POINT('Ctrl Pts',(-0.00307345235301464,-0.0141375199213023,
-0.0124218328862067));
#14360=CARTESIAN_POINT('Ctrl Pts',(-0.00307349994219986,-0.0141247811395518,
-0.0121764493549137));
#14361=CARTESIAN_POINT('Ctrl Pts',(-0.00307360801018469,-0.0140958532546356,
-0.0116192197318156));
#14362=CARTESIAN_POINT('Ctrl Pts',(-0.00291784336291199,-0.0140669253697195,
-0.01106009256286));
#14363=CARTESIAN_POINT('Ctrl Pts',(-0.00262806820907844,-0.0140379974848033,
-0.0105822222946308));
#14364=CARTESIAN_POINT('Ctrl Pts',(-0.00250046183716071,-0.0140252587030528,
-0.0103717857186533));
#14365=CARTESIAN_POINT('Ctrl Pts',(-0.00234755430279202,-0.0140125199213023,
-0.0101769508500219));
#14366=CARTESIAN_POINT('Ctrl Pts',(-0.00217409629185899,-0.0139997811395518,
-0.0100033644917136));
#14367=CARTESIAN_POINT('Ctrl Pts',(-0.00178012474201237,-0.0139708478111779,
-0.00960910142915965));
#14368=CARTESIAN_POINT('Ctrl Pts',(-0.00127454520834623,-0.0139419144828041,
-0.00932377147832942));
#14369=CARTESIAN_POINT('Ctrl Pts',(-0.000731656198816013,-0.0139129811544302,
-0.00919070982991583));
#14370=CARTESIAN_POINT('Ctrl Pts',(-0.000492734864759313,-0.0139002478161374,
-0.00913215040802171));
#14371=CARTESIAN_POINT('Ctrl Pts',(-0.000246961692959371,-0.0138875144778446,
-0.00910248760127359));
#14372=CARTESIAN_POINT('Ctrl Pts',(-1.67727568855383E-6,-0.0138747811395518,
-0.00910235374422101));
#14373=CARTESIAN_POINT('Ctrl Pts',(0.000553616747781886,-0.0138459544136982,
-0.00910205070816952));
#14374=CARTESIAN_POINT('Ctrl Pts',(0.00111100838919363,-0.0138171276878447,
-0.00925657261563487));
#14375=CARTESIAN_POINT('Ctrl Pts',(0.00158783372454616,-0.0137883009619911,
-0.0095442784133702));
#14376=CARTESIAN_POINT('Ctrl Pts',(0.00180022028260421,-0.013775461021178,
-0.00967242773678896));
#14377=CARTESIAN_POINT('Ctrl Pts',(0.00199677892354685,-0.0137626210803649,
-0.00982630026110334));
#14378=CARTESIAN_POINT('Ctrl Pts',(0.00217172384864896,-0.0137497811395518,
-0.0100009928829438));
#14379=CARTESIAN_POINT('Ctrl Pts',(0.00257185989579124,-0.0137204134790752,
-0.0104005518591608));
#14380=CARTESIAN_POINT('Ctrl Pts',(0.00285965598737614,-0.0136910458185987,
-0.0109145705767058));
#14381=CARTESIAN_POINT('Ctrl Pts',(0.00299058522067098,-0.0136616781581221,
-0.0114667677572287));
#14382=CARTESIAN_POINT('Ctrl Pts',(0.00304541762558932,-0.013649379151932,
-0.0116980247396096));
#14383=CARTESIAN_POINT('Ctrl Pts',(0.00307328564276539,-0.0136370801457419,
-0.0119356374308079));
#14384=CARTESIAN_POINT('Ctrl Pts',(0.00307349876212316,-0.0136247811395518,
-0.0121730948037442));
#14385=CARTESIAN_POINT('',(-0.00289832479094502,-0.0131787743898721,-0.0131986512412849));
#14386=CARTESIAN_POINT('Ctrl Pts',(0.00307349999999835,-0.0136246379448887,
-0.0121758564690173));
#14387=CARTESIAN_POINT('Ctrl Pts',(0.00307349925680341,-0.0135874826486382,
-0.0128936063191386));
#14388=CARTESIAN_POINT('Ctrl Pts',(0.00254975520022809,-0.0135131720561371,
-0.0143255433828562));
#14389=CARTESIAN_POINT('Ctrl Pts',(0.000563092149707625,-0.0134017061673856,
-0.0154635975636764));
#14390=CARTESIAN_POINT('Ctrl Pts',(-0.00168906107875945,-0.013290240278634,
-0.0150515256885247));
#14391=CARTESIAN_POINT('Ctrl Pts',(-0.00265947231698363,-0.0132159296861329,
-0.0138754926872979));
#14392=CARTESIAN_POINT('Ctrl Pts',(-0.00289832479094299,-0.0131787743898824,
-0.0131986512412907));
#14393=CARTESIAN_POINT('',(-0.00132721716346492,-0.0131811320840746,-0.00940066304710818));
#14394=CARTESIAN_POINT('Origin',(0.,-0.0131787743898824,-0.012175853286568));
#14395=CARTESIAN_POINT('',(0.00307349448959333,-0.0138578957495471,-0.0121758980191793));
#14396=CARTESIAN_POINT('Ctrl Pts',(-0.00132669617051746,-0.0131812255681309,
-0.00940188040761344));
#14397=CARTESIAN_POINT('Ctrl Pts',(-0.0018196919059704,-0.013209392323556,
-0.00963774239526866));
#14398=CARTESIAN_POINT('Ctrl Pts',(-0.00224604746585449,-0.0132329816360925,
-0.0100099352992059));
#14399=CARTESIAN_POINT('Ctrl Pts',(-0.00255047574633007,-0.0132616754020662,
-0.010462835535099));
#14400=CARTESIAN_POINT('Ctrl Pts',(-0.0028069991368114,-0.0132858539117688,
-0.0108444673068898));
#14401=CARTESIAN_POINT('Ctrl Pts',(-0.00297896355371799,-0.013313136885812,
-0.0112851249369724));
#14402=CARTESIAN_POINT('Ctrl Pts',(-0.00304385678131681,-0.0133371739441656,
-0.0117402552548227));
#14403=CARTESIAN_POINT('Ctrl Pts',(-0.00305597537574073,-0.0133416627848677,
-0.0118252493279509));
#14404=CARTESIAN_POINT('Ctrl Pts',(-0.00306438599299585,-0.0133460384264664,
-0.0119107898015695));
#14405=CARTESIAN_POINT('Ctrl Pts',(-0.0030692671948678,-0.0133502595110746,
-0.0119966084976508));
#14406=CARTESIAN_POINT('Ctrl Pts',(-0.00310028648940561,-0.0133770838609308,
-0.0125419732419139));
#14407=CARTESIAN_POINT('Ctrl Pts',(-0.00298081293685468,-0.0134022194800802,
-0.0130948328051767));
#14408=CARTESIAN_POINT('Ctrl Pts',(-0.00273221661189375,-0.0134317107918798,
-0.0135805976612059));
#14409=CARTESIAN_POINT('Ctrl Pts',(-0.00255384908424496,-0.013452870768294,
-0.0139291332898087));
#14410=CARTESIAN_POINT('Ctrl Pts',(-0.00230883215863813,-0.0134753555341454,
-0.0142457915368782));
#14411=CARTESIAN_POINT('Ctrl Pts',(-0.00201232942765066,-0.0134960192056483,
-0.0145016804695592));
#14412=CARTESIAN_POINT('Ctrl Pts',(-0.00189558715694983,-0.0135041551304819,
-0.01460243183515));
#14413=CARTESIAN_POINT('Ctrl Pts',(-0.00177086859135001,-0.0135120087420253,
-0.0146938583727293));
#14414=CARTESIAN_POINT('Ctrl Pts',(-0.00164017617792611,-0.0135193880226992,
-0.0147758852505195));
#14415=CARTESIAN_POINT('Ctrl Pts',(-0.00117755037596263,-0.0135455092454253,
-0.0150662444926982));
#14416=CARTESIAN_POINT('Ctrl Pts',(-0.000636279900124425,-0.0135718670537832,
-0.0152296424015862));
#14417=CARTESIAN_POINT('Ctrl Pts',(-9.08461531836337E-5,-0.0136020240639464,
-0.0152471101049117));
#14418=CARTESIAN_POINT('Ctrl Pts',(0.000232536519338722,-0.0136199038790413,
-0.0152574665462135));
#14419=CARTESIAN_POINT('Ctrl Pts',(0.000558965697174523,-0.0136378116522388,
-0.0152183595818082));
#14420=CARTESIAN_POINT('Ctrl Pts',(0.000869600935216467,-0.0136548250124208,
-0.0151265683100328));
#14421=CARTESIAN_POINT('Ctrl Pts',(0.00108289896946619,-0.0136665072552522,
-0.0150635397304216));
#14422=CARTESIAN_POINT('Ctrl Pts',(0.00128876025895534,-0.0136777677915046,
-0.014975755649426));
#14423=CARTESIAN_POINT('Ctrl Pts',(0.00148321885597551,-0.0136883080044757,
-0.0148679674384441));
#14424=CARTESIAN_POINT('Ctrl Pts',(0.00196087599623186,-0.0137141983896922,
-0.0146032025506996));
#14425=CARTESIAN_POINT('Ctrl Pts',(0.00236635307333829,-0.0137418711774504,
-0.0142092494390052));
#14426=CARTESIAN_POINT('Ctrl Pts',(0.00264532404574679,-0.0137724708213245,
-0.0137401927099414));
#14427=CARTESIAN_POINT('Ctrl Pts',(0.002775992199874,-0.0137868034916645,
-0.0135204896475096));
#14428=CARTESIAN_POINT('Ctrl Pts',(0.00288080040326081,-0.0138005638977075,
-0.0132846571839918));
#14429=CARTESIAN_POINT('Ctrl Pts',(0.00295272353125746,-0.0138138184898977,
-0.0130390338119726));
#14430=CARTESIAN_POINT('Ctrl Pts',(0.00303435323401673,-0.0138288618904118,
-0.0127602616922508));
#14431=CARTESIAN_POINT('Ctrl Pts',(0.00307355007668885,-0.0138432537375257,
-0.0124689291532911));
#14432=CARTESIAN_POINT('Ctrl Pts',(0.00307310808197872,-0.0138570911799035,
-0.0121785284790189));
#14433=CARTESIAN_POINT('',(0.00307349989340788,-0.0148577382240435,-0.0121752793767589));
#14434=CARTESIAN_POINT('Ctrl Pts',(0.00307349999999152,-0.01385790722318,
-0.0121758605072862));
#14435=CARTESIAN_POINT('Ctrl Pts',(0.00307350133207145,-0.0138872385042673,
-0.0116088612229254));
#14436=CARTESIAN_POINT('Ctrl Pts',(0.0029123013203729,-0.0139165723499641,
-0.0110417229255565));
#14437=CARTESIAN_POINT('Ctrl Pts',(0.00261419264222686,-0.0139459126747149,
-0.0105595615185512));
#14438=CARTESIAN_POINT('Ctrl Pts',(0.00248926933561196,-0.01395820782294,
-0.0103575103818322));
#14439=CARTESIAN_POINT('Ctrl Pts',(0.00234092856375039,-0.0139705041089217,
-0.0101702098174937));
#14440=CARTESIAN_POINT('Ctrl Pts',(0.0021733792536772,-0.0139828018207156,
-0.0100026471597294));
#14441=CARTESIAN_POINT('Ctrl Pts',(0.00178091745653428,-0.0140116075619584,
-0.00961015409740957));
#14442=CARTESIAN_POINT('Ctrl Pts',(0.00127750678143459,-0.0140404211261745,
-0.00932548282021525));
#14443=CARTESIAN_POINT('Ctrl Pts',(0.000736760751761841,-0.0140692314072482,
-0.00919196558011481));
#14444=CARTESIAN_POINT('Ctrl Pts',(0.00049575116194729,-0.0140820721007401,
-0.00913245717227823));
#14445=CARTESIAN_POINT('Ctrl Pts',(0.000247713071908436,-0.0140949121420458,
-0.00910237122778308));
#14446=CARTESIAN_POINT('Ctrl Pts',(2.22705864387592E-7,-0.0141077505478671,
-0.00910235329462672));
#14447=CARTESIAN_POINT('Ctrl Pts',(-0.000557104288925352,-0.0141366615323579,
-0.00910231291070271));
#14448=CARTESIAN_POINT('Ctrl Pts',(-0.00111629365783261,-0.0141655642231179,
-0.0092581981881314));
#14449=CARTESIAN_POINT('Ctrl Pts',(-0.00159417362234604,-0.0141944997930902,
-0.00954811419908839));
#14450=CARTESIAN_POINT('Ctrl Pts',(-0.0018046348026978,-0.0142072431903087,
-0.00967579493567463));
#14451=CARTESIAN_POINT('Ctrl Pts',(-0.00199948134856071,-0.0142199929646937,
-0.00982878575482296));
#14452=CARTESIAN_POINT('Ctrl Pts',(-0.00217306428972824,-0.014232752633238,
-0.010002332216334));
#14453=CARTESIAN_POINT('Ctrl Pts',(-0.00256717902049182,-0.0142617230683459,
-0.0103963641211593));
#14454=CARTESIAN_POINT('Ctrl Pts',(-0.00285235991347764,-0.0142907445081475,
-0.0109019563653772));
#14455=CARTESIAN_POINT('Ctrl Pts',(-0.00298529505148537,-0.0143196635229212,
-0.0114448158692004));
#14456=CARTESIAN_POINT('Ctrl Pts',(-0.00304385423221388,-0.0143324026213869,
-0.0116839505951352));
#14457=CARTESIAN_POINT('Ctrl Pts',(-0.00307346616249905,-0.0143451218444243,
-0.0119299420581625));
#14458=CARTESIAN_POINT('Ctrl Pts',(-0.0030734999708532,-0.0143578080768281,
-0.0121754300072245));
#14459=CARTESIAN_POINT('Ctrl Pts',(-0.00307357671814756,-0.01438660669886,
-0.0127327045733367));
#14460=CARTESIAN_POINT('Ctrl Pts',(-0.00291775615137512,-0.0144152353131311,
-0.0132918738548947));
#14461=CARTESIAN_POINT('Ctrl Pts',(-0.00262789661615805,-0.0144438906823375,
-0.0137697672192361));
#14462=CARTESIAN_POINT('Ctrl Pts',(-0.00250020522803293,-0.0144565141893353,
-0.0139802928692646));
#14463=CARTESIAN_POINT('Ctrl Pts',(-0.00234718809325915,-0.0144691428885395,
-0.0141752011655309));
#14464=CARTESIAN_POINT('Ctrl Pts',(-0.0021736016670944,-0.0144817936014535,
-0.0143488369594844));
#14465=CARTESIAN_POINT('Ctrl Pts',(-0.00177965194790562,-0.0145105040537058,
-0.0147428987175403));
#14466=CARTESIAN_POINT('Ctrl Pts',(-0.00127416024100349,-0.0145393278877474,
-0.0150280814152012));
#14467=CARTESIAN_POINT('Ctrl Pts',(-0.000731386520761171,-0.0145682115985004,
-0.0151610628281563));
#14468=CARTESIAN_POINT('Ctrl Pts',(-0.000492097458306903,-0.0145809453691465,
-0.0152196894647142));
#14469=CARTESIAN_POINT('Ctrl Pts',(-0.000245938049725031,-0.0145936907774618,
-0.0152493305261509));
#14470=CARTESIAN_POINT('Ctrl Pts',(-2.84602609272593E-7,-0.0146064432387867,
-0.0152493532733812));
#14471=CARTESIAN_POINT('Ctrl Pts',(0.000555018639657029,-0.0146352703657973,
-0.0152494046938309));
#14472=CARTESIAN_POINT('Ctrl Pts',(0.00111234868679064,-0.0146641335331714,
-0.0150946252343135));
#14473=CARTESIAN_POINT('Ctrl Pts',(0.00158904880133423,-0.0146930471839194,
-0.0148066946266959));
#14474=CARTESIAN_POINT('Ctrl Pts',(0.00180156679688988,-0.0147059371978164,
-0.0146783320907469));
#14475=CARTESIAN_POINT('Ctrl Pts',(0.00199821641796431,-0.0147188372451401,
-0.0145242071941443));
#14476=CARTESIAN_POINT('Ctrl Pts',(0.00217319919795374,-0.0147317486055931,
-0.0143492394685362));
#14477=CARTESIAN_POINT('Ctrl Pts',(0.0025730612372781,-0.0147612530112353,
-0.0139494118307433));
#14478=CARTESIAN_POINT('Ctrl Pts',(0.00286050813803622,-0.014790816493068,
-0.0134352012199921));
#14479=CARTESIAN_POINT('Ctrl Pts',(0.00299106370368742,-0.0148204339609196,
-0.0128829177606223));
#14480=CARTESIAN_POINT('Ctrl Pts',(0.00304579235279836,-0.0148328495480876,
-0.0126514015666794));
#14481=CARTESIAN_POINT('Ctrl Pts',(0.00307350023801115,-0.0148452746220606,
-0.0124135355879753));
#14482=CARTESIAN_POINT('Ctrl Pts',(0.00307349999999846,-0.014857708807874,
-0.0121758502088256));
#14483=CARTESIAN_POINT('',(0.00307349955219906,-0.0158577062176384,-0.012174689201038));
#14484=CARTESIAN_POINT('Ctrl Pts',(0.00307349978681731,-0.0148577676402129,
-0.0121747085446921));
#14485=CARTESIAN_POINT('Ctrl Pts',(0.00307328860483376,-0.0148871267056932,
-0.0116077092929736));
#14486=CARTESIAN_POINT('Ctrl Pts',(0.00291187603779568,-0.0149164857711735,
-0.0110406314886779));
#14487=CARTESIAN_POINT('Ctrl Pts',(0.00261358670794305,-0.0149458448366537,
-0.010558581890019));
#14488=CARTESIAN_POINT('Ctrl Pts',(0.00248859297119646,-0.0149581473192923,
-0.0103565861275044));
#14489=CARTESIAN_POINT('Ctrl Pts',(0.00234018929001624,-0.0149704498019308,
-0.0101693484610414));
#14490=CARTESIAN_POINT('Ctrl Pts',(0.00217258590305342,-0.0149827522845693,
-0.0100018540354419));
#14491=CARTESIAN_POINT('Ctrl Pts',(0.00177998102983827,-0.0150115704052771,
-0.00960950440028021));
#14492=CARTESIAN_POINT('Ctrl Pts',(0.00127646674261242,-0.0150403885259848,
-0.00932501696702219));
#14493=CARTESIAN_POINT('Ctrl Pts',(0.0007356723147371,-0.0150692066466926,
-0.00919169704143128));
#14494=CARTESIAN_POINT('Ctrl Pts',(0.000494655419529813,-0.0150820500741036,
-0.00913228009318085));
#14495=CARTESIAN_POINT('Ctrl Pts',(0.000246621602187934,-0.0150948935015146,
-0.00910228463910051));
#14496=CARTESIAN_POINT('Ctrl Pts',(-8.54034130405478E-7,-0.0151077369289256,
-0.00910235340521342));
#14497=CARTESIAN_POINT('Ctrl Pts',(-0.000558194471297123,-0.015136661640685,
-0.00910250827353096));
#14498=CARTESIAN_POINT('Ctrl Pts',(-0.00111734149881382,-0.0151655863524443,
-0.00925859673664403));
#14499=CARTESIAN_POINT('Ctrl Pts',(-0.00159512763372221,-0.0151945110642037,
-0.00954869320728318));
#14500=CARTESIAN_POINT('Ctrl Pts',(-0.00180551810764494,-0.0152072479005631,
-0.00967643557877912));
#14501=CARTESIAN_POINT('Ctrl Pts',(-0.0020002885992337,-0.0152199847369226,
-0.00982947658612617));
#14502=CARTESIAN_POINT('Ctrl Pts',(-0.00217379374682141,-0.015232721573282,
-0.0100030617649711));
#14503=CARTESIAN_POINT('Ctrl Pts',(-0.00256774114811238,-0.0152616408512068,
-0.01039719087906));
#14504=CARTESIAN_POINT('Ctrl Pts',(-0.00285273819986065,-0.0152905601291315,
-0.0109028266790015));
#14505=CARTESIAN_POINT('Ctrl Pts',(-0.00298550494832231,-0.0153194794070563,
-0.0114456735459853));
#14506=CARTESIAN_POINT('Ctrl Pts',(-0.00304400398090827,-0.0153322216772503,
-0.0116848600661706));
#14507=CARTESIAN_POINT('Ctrl Pts',(-0.00307354494863363,-0.0153449639474444,
-0.0119308959084206));
#14508=CARTESIAN_POINT('Ctrl Pts',(-0.00307349994837537,-0.0153577062176384,
-0.0121764166129453));
#14509=CARTESIAN_POINT('Ctrl Pts',(-0.00307339781783225,-0.0153866254955631,
-0.0127336392571295));
#14510=CARTESIAN_POINT('Ctrl Pts',(-0.00291742600410256,-0.0154155447734879,
-0.0132927020720123));
#14511=CARTESIAN_POINT('Ctrl Pts',(-0.00262747630529442,-0.0154444640514126,
-0.0137704599826172));
#14512=CARTESIAN_POINT('Ctrl Pts',(-0.00249972009317517,-0.0154572063216067,
-0.0139809673265453));
#14513=CARTESIAN_POINT('Ctrl Pts',(-0.00234663993625058,-0.0154699485918007,
-0.0141758459158392));
#14514=CARTESIAN_POINT('Ctrl Pts',(-0.00217299712068187,-0.0154826908619947,
-0.0143494415096372));
#14515=CARTESIAN_POINT('Ctrl Pts',(-0.00177883122144032,-0.0155116155737541,
-0.0147435002163547));
#14516=CARTESIAN_POINT('Ctrl Pts',(-0.00127311414354502,-0.0155405402855134,
-0.0150285730660098));
#14517=CARTESIAN_POINT('Ctrl Pts',(-0.000730164233966559,-0.0155694649972728,
-0.0151613620273653));
#14518=CARTESIAN_POINT('Ctrl Pts',(-0.000491079253372756,-0.0155822018336322,
-0.0152198349098332));
#14519=CARTESIAN_POINT('Ctrl Pts',(-0.000245149159454215,-0.0155949386699917,
-0.0152493750433145));
#14520=CARTESIAN_POINT('Ctrl Pts',(2.72618638915599E-7,-0.0156076755063511,
-0.0152493532744675));
#14521=CARTESIAN_POINT('Ctrl Pts',(0.000555559208324033,-0.0156364936270589,
-0.0152493040206933));
#14522=CARTESIAN_POINT('Ctrl Pts',(0.00111284669964006,-0.0156653117477667,
-0.0150944325339671));
#14523=CARTESIAN_POINT('Ctrl Pts',(0.00158948612246453,-0.0156941298684745,
-0.0148064304316904));
#14524=CARTESIAN_POINT('Ctrl Pts',(0.00180191093289366,-0.0157069732958855,
-0.0146780759795623));
#14525=CARTESIAN_POINT('Ctrl Pts',(0.00199847381907867,-0.0157198167232965,
-0.0145239793332489));
#14526=CARTESIAN_POINT('Ctrl Pts',(0.00217338267989119,-0.0157326601507075,
-0.0143490559868944));
#14527=CARTESIAN_POINT('Ctrl Pts',(0.00257321058667491,-0.0157620192161878,
-0.0139491949673004));
#14528=CARTESIAN_POINT('Ctrl Pts',(0.00286061375982055,-0.0157913782816681,
-0.0134349608491815));
#14529=CARTESIAN_POINT('Ctrl Pts',(0.0029911228767067,-0.0158207373471483,
-0.0128826673968034));
#14530=CARTESIAN_POINT('Ctrl Pts',(0.00304581079399547,-0.0158330398297868,
-0.0126512369851707));
#14531=CARTESIAN_POINT('Ctrl Pts',(0.00307349860159295,-0.0158453423124253,
-0.0124134640517282));
#14532=CARTESIAN_POINT('Ctrl Pts',(0.00307349999994677,-0.0158576447950638,
-0.0121758713756698));
#14533=CARTESIAN_POINT('',(0.00307349958720421,-0.0168578266932082,-0.0121769697098861));
#14534=CARTESIAN_POINT('Ctrl Pts',(0.00307349910445136,-0.0158577676402129,
-0.0121735070264063));
#14535=CARTESIAN_POINT('Ctrl Pts',(0.0030730662635019,-0.015887135733148,
-0.0116065041433245));
#14536=CARTESIAN_POINT('Ctrl Pts',(0.00291142998921608,-0.0159165038260831,
-0.0110394863287188));
#14537=CARTESIAN_POINT('Ctrl Pts',(0.00261294882229721,-0.0159458719190182,
-0.0105575514908304));
#14538=CARTESIAN_POINT('Ctrl Pts',(0.00248795287356632,-0.0159581704927498,
-0.010355730039547));
#14539=CARTESIAN_POINT('Ctrl Pts',(0.00233958187208303,-0.0159704690664813,
-0.0101686574839441));
#14540=CARTESIAN_POINT('Ctrl Pts',(0.00217203976625694,-0.0159827676402129,
-0.0100013083907699));
#14541=CARTESIAN_POINT('Ctrl Pts',(0.00177933049551567,-0.0160115948051663,
-0.0096090515308265));
#14542=CARTESIAN_POINT('Ctrl Pts',(0.00127573698229395,-0.0160404219701197,
-0.00932468905152511));
#14543=CARTESIAN_POINT('Ctrl Pts',(0.000734901807145515,-0.016069249135073,
-0.00919150719673301));
#14544=CARTESIAN_POINT('Ctrl Pts',(0.000494016025655897,-0.0160820886367863,
-0.00913218854172314));
#14545=CARTESIAN_POINT('Ctrl Pts',(0.000246129473808355,-0.0160949281384996,
-0.00910225723428693));
#14546=CARTESIAN_POINT('Ctrl Pts',(-1.1965279448354E-6,-0.0161077676402129,
-0.00910235351946507));
#14547=CARTESIAN_POINT('Ctrl Pts',(-0.000558544714015742,-0.0161367014075452,
-0.00910257049774071));
#14548=CARTESIAN_POINT('Ctrl Pts',(-0.00111768053985367,-0.0161656351748775,
-0.00925872543230002));
#14549=CARTESIAN_POINT('Ctrl Pts',(-0.00159543770967884,-0.0161945689422098,
-0.00954888150054006));
#14550=CARTESIAN_POINT('Ctrl Pts',(-0.00180568457728475,-0.0162073018415442,
-0.00967657064539715));
#14551=CARTESIAN_POINT('Ctrl Pts',(-0.00200032768393728,-0.0162200347408785,
-0.00982952551388758));
#14552=CARTESIAN_POINT('Ctrl Pts',(-0.00217373222877299,-0.0162327676402129,
-0.0100030002202893));
#14553=CARTESIAN_POINT('Ctrl Pts',(-0.00256769613031811,-0.0162616959633114,
-0.010397123524371));
#14554=CARTESIAN_POINT('Ctrl Pts',(-0.0028527088982565,-0.0162906242864098,
-0.010902758378207));
#14555=CARTESIAN_POINT('Ctrl Pts',(-0.00298548896101624,-0.0163195526095083,
-0.0114456081813707));
#14556=CARTESIAN_POINT('Ctrl Pts',(-0.00304395754395783,-0.0163322909530765,
-0.01168464752268));
#14557=CARTESIAN_POINT('Ctrl Pts',(-0.00307350373554943,-0.0163450292966447,
-0.0119305284371561));
#14558=CARTESIAN_POINT('Ctrl Pts',(-0.00307349999964376,-0.0163577676402129,
-0.0121759000821285));
#14559=CARTESIAN_POINT('Ctrl Pts',(-0.00307349151553545,-0.0163866959633114,
-0.0127331303206558));
#14560=CARTESIAN_POINT('Ctrl Pts',(-0.00291760959876268,-0.0164156242864098,
-0.0132922253787799));
#14561=CARTESIAN_POINT('Ctrl Pts',(-0.00262773400439643,-0.0164445526095082,
-0.0137700352875036));
#14562=CARTESIAN_POINT('Ctrl Pts',(-0.00250008972648538,-0.0164572909530765,
-0.0139804348587788));
#14563=CARTESIAN_POINT('Ctrl Pts',(-0.00234715003467735,-0.0164700292966447,
-0.0141752289474491));
#14564=CARTESIAN_POINT('Ctrl Pts',(-0.00217366606222184,-0.0164827676402129,
-0.0143487725441342));
#14565=CARTESIAN_POINT('Ctrl Pts',(-0.00177961601418933,-0.0165117014075452,
-0.0147429580221444));
#14566=CARTESIAN_POINT('Ctrl Pts',(-0.00127397940839639,-0.0165406351748775,
-0.0150281879702471));
#14567=CARTESIAN_POINT('Ctrl Pts',(-0.000731063511943571,-0.0165695689422098,
-0.0151611419478947));
#14568=CARTESIAN_POINT('Ctrl Pts',(-0.00049214220670302,-0.0165823018415442,
-0.0152196510799426));
#14569=CARTESIAN_POINT('Ctrl Pts',(-0.000246375470689803,-0.0165950347408785,
-0.0152492650717026));
#14570=CARTESIAN_POINT('Ctrl Pts',(-1.10293681041439E-6,-0.0166077676402129,
-0.0152493530886616));
#14571=CARTESIAN_POINT('Ctrl Pts',(0.000554191784918156,-0.0166365948051663,
-0.0152495523582333));
#14572=CARTESIAN_POINT('Ctrl Pts',(0.00111155506214211,-0.0166654219701197,
-0.0150949259473566));
#14573=CARTESIAN_POINT('Ctrl Pts',(0.00158832691156067,-0.016694249135073,
-0.0148071305186285));
#14574=CARTESIAN_POINT('Ctrl Pts',(0.00180067914901998,-0.0167070886367863,
-0.0146789476083005));
#14575=CARTESIAN_POINT('Ctrl Pts',(0.00199720019475119,-0.0167199281384996,
-0.0145250469724957));
#14576=CARTESIAN_POINT('Ctrl Pts',(0.00217210598231125,-0.0167327676402129,
-0.0143503320405605));
#14577=CARTESIAN_POINT('Ctrl Pts',(0.00257217208601626,-0.016762135733148,
-0.0139507024853955));
#14578=CARTESIAN_POINT('Ctrl Pts',(0.00285987790424067,-0.0167915038260831,
-0.0134366328536536));
#14579=CARTESIAN_POINT('Ctrl Pts',(0.00299070999424267,-0.0168208719190182,
-0.012884412373958));
#14580=CARTESIAN_POINT('Ctrl Pts',(0.0030454989827174,-0.0168331704927497,
-0.0126531571712238));
#14581=CARTESIAN_POINT('Ctrl Pts',(0.00307332514268951,-0.0168454690664813,
-0.0124155516398577));
#14582=CARTESIAN_POINT('Ctrl Pts',(0.00307349917447235,-0.0168577676402129,
-0.012178105955595));
#14583=CARTESIAN_POINT('',(0.00307349973395781,-0.017857767640213,-0.0121771320990067));
#14584=CARTESIAN_POINT('Ctrl Pts',(0.00307349999993608,-0.0168578857462035,
-0.0121758334641773));
#14585=CARTESIAN_POINT('Ctrl Pts',(0.00307349634310224,-0.0168872451650051,
-0.011608834024638));
#14586=CARTESIAN_POINT('Ctrl Pts',(0.00291229126051317,-0.0169166045838068,
-0.0110416970556195));
#14587=CARTESIAN_POINT('Ctrl Pts',(0.00261417824885523,-0.0169459640026085,
-0.0105595382389228));
#14588=CARTESIAN_POINT('Ctrl Pts',(0.00248926148152478,-0.0169582663293905,
-0.010357501701213));
#14589=CARTESIAN_POINT('Ctrl Pts',(0.00234093052159938,-0.0169705686561726,
-0.0101702139657608));
#14590=CARTESIAN_POINT('Ctrl Pts',(0.00217339345729084,-0.0169828709829547,
-0.0100026613645675));
#14591=CARTESIAN_POINT('Ctrl Pts',(0.00178093414907792,-0.0170116894577097,
-0.0096101656608555));
#14592=CARTESIAN_POINT('Ctrl Pts',(0.00127752528436554,-0.0170405079324647,
-0.0093254911163739));
#14593=CARTESIAN_POINT('Ctrl Pts',(0.000736780138390888,-0.0170693264072197,
-0.00919197036699293));
#14594=CARTESIAN_POINT('Ctrl Pts',(0.000495791105552733,-0.0170821696780484,
-0.00913246537375042));
#14595=CARTESIAN_POINT('Ctrl Pts',(0.000247774567391759,-0.0170950129488772,
-0.00910237784625514));
#14596=CARTESIAN_POINT('Ctrl Pts',(3.04836335295681E-7,-0.0171078562197059,
-0.00910235330167525));
#14597=CARTESIAN_POINT('Ctrl Pts',(-0.000557035926712533,-0.017136781285948,
-0.00910229802342031));
#14598=CARTESIAN_POINT('Ctrl Pts',(-0.00111624201296547,-0.0171657063521901,
-0.00925817581220162));
#14599=CARTESIAN_POINT('Ctrl Pts',(-0.00159413762858014,-0.0171946314184321,
-0.00954809236304452));
#14600=CARTESIAN_POINT('Ctrl Pts',(-0.00180457113853043,-0.0172073680977738,
-0.0096757523695254));
#14601=CARTESIAN_POINT('Ctrl Pts',(-0.00199939495831796,-0.0172201047771154,
-0.00982871566688341));
#14602=CARTESIAN_POINT('Ctrl Pts',(-0.00217296233084268,-0.0172328414564571,
-0.0100022302836575));
#14603=CARTESIAN_POINT('Ctrl Pts',(-0.00256706069867207,-0.0172617610884542,
-0.0103962088654065));
#14604=CARTESIAN_POINT('Ctrl Pts',(-0.00285225122890694,-0.0172906807204512,
-0.0109017358769659));
#14605=CARTESIAN_POINT('Ctrl Pts',(-0.00298522556645655,-0.0173196003524483,
-0.0114445321755718));
#14606=CARTESIAN_POINT('Ctrl Pts',(-0.00304381462849378,-0.0173323424660349,
-0.0116836905470188));
#14607=CARTESIAN_POINT('Ctrl Pts',(-0.00307344965072599,-0.0173450845796216,
-0.0119297089794094));
#14608=CARTESIAN_POINT('Ctrl Pts',(-0.00307349993553538,-0.0173578266932083,
-0.0121752237915101));
#14609=CARTESIAN_POINT('Ctrl Pts',(-0.00307361406245576,-0.0173867463252053,
-0.0127324467331738));
#14610=CARTESIAN_POINT('Ctrl Pts',(-0.00291785907157083,-0.0174156659572024,
-0.0132915702771264));
#14611=CARTESIAN_POINT('Ctrl Pts',(-0.00262809456714721,-0.0174445855891994,
-0.0137694408103958));
#14612=CARTESIAN_POINT('Ctrl Pts',(-0.00250042308677956,-0.0174573277027861,
-0.0139799926118594));
#14613=CARTESIAN_POINT('Ctrl Pts',(-0.00234742282997037,-0.0174700698163728,
-0.0141749262395666));
#14614=CARTESIAN_POINT('Ctrl Pts',(-0.00217385252425702,-0.0174828119299594,
-0.0143485860020069));
#14615=CARTESIAN_POINT('Ctrl Pts',(-0.00177984154984009,-0.0175117369962015,
-0.0147428000464823));
#14616=CARTESIAN_POINT('Ctrl Pts',(-0.00127423643353935,-0.0175406620624436,
-0.0150280719926622));
#14617=CARTESIAN_POINT('Ctrl Pts',(-0.000731338562493786,-0.0175695871286856,
-0.015161074577687));
#14618=CARTESIAN_POINT('Ctrl Pts',(-0.000492282373619284,-0.0175823238080273,
-0.0152196400884069));
#14619=CARTESIAN_POINT('Ctrl Pts',(-0.000246370023034821,-0.0175950604873689,
-0.0152492769502351));
#14620=CARTESIAN_POINT('Ctrl Pts',(-9.54153753620061E-7,-0.0176077971667106,
-0.0152493531384518));
#14621=CARTESIAN_POINT('Ctrl Pts',(0.000554332734110935,-0.0176366156414656,
-0.015249525524687));
#14622=CARTESIAN_POINT('Ctrl Pts',(0.00111168225525367,-0.0176654341162206,
-0.0150948763166834));
#14623=CARTESIAN_POINT('Ctrl Pts',(0.00158843673613355,-0.0176942525909756,
-0.0148070642217173));
#14624=CARTESIAN_POINT('Ctrl Pts',(0.00180090762395152,-0.0177070958618043,
-0.0146787975901602));
#14625=CARTESIAN_POINT('Ctrl Pts',(0.00199752762317113,-0.0177199391326331,
-0.0145247836831463));
#14626=CARTESIAN_POINT('Ctrl Pts',(0.00217250307581148,-0.0177327824034618,
-0.0143499353079155));
#14627=CARTESIAN_POINT('Ctrl Pts',(0.0025724928963627,-0.0177621418222635,
-0.0139502359833711));
#14628=CARTESIAN_POINT('Ctrl Pts',(0.00286010416722769,-0.0177915012410651,
-0.0134361180366009));
#14629=CARTESIAN_POINT('Ctrl Pts',(0.00299083671501046,-0.0178208606598668,
-0.012883877293316));
#14630=CARTESIAN_POINT('Ctrl Pts',(0.00304561690445299,-0.0178331629866489,
-0.0126524746851047));
#14631=CARTESIAN_POINT('Ctrl Pts',(0.00307340087954239,-0.0178454653134309,
-0.0124147189475048));
#14632=CARTESIAN_POINT('Ctrl Pts',(0.00307349973395781,-0.017857767640213,
-0.0121771320990067));
#14633=CARTESIAN_POINT('',(0.00307349903227376,-0.0188577420250978,-0.0121736488040434));
#14634=CARTESIAN_POINT('Ctrl Pts',(0.00307349999999813,-0.0178578333594276,
-0.0121758566778537));
#14635=CARTESIAN_POINT('Ctrl Pts',(0.0030735006215337,-0.0178869007967827,
-0.0116125647073703));
#14636=CARTESIAN_POINT('Ctrl Pts',(0.00291433696992175,-0.0179159846530298,
-0.0110488283918617));
#14637=CARTESIAN_POINT('Ctrl Pts',(0.00261987653841084,-0.0179450851484625,
-0.0105687910060336));
#14638=CARTESIAN_POINT('Ctrl Pts',(0.00249371415197432,-0.0179575533362304,
-0.0103631176601649));
#14639=CARTESIAN_POINT('Ctrl Pts',(0.00234336486540254,-0.017970024578483,
-0.0101726346057528));
#14640=CARTESIAN_POINT('Ctrl Pts',(0.00217330443424238,-0.0179824988925469,
-0.0100025723369102));
#14641=CARTESIAN_POINT('Ctrl Pts',(0.00177902997917332,-0.018011419808167,
-0.00960829362128951));
#14642=CARTESIAN_POINT('Ctrl Pts',(0.00127275718761501,-0.0180403572352389,
-0.009322737625378));
#14643=CARTESIAN_POINT('Ctrl Pts',(0.000728564199173013,-0.0180693105259971,
-0.00918995368046224));
#14644=CARTESIAN_POINT('Ctrl Pts',(0.000490185945838011,-0.018081993223176,
-0.00913178901180201));
#14645=CARTESIAN_POINT('Ctrl Pts',(0.000244911249906314,-0.0180946789642627,
-0.00910235416870036));
#14646=CARTESIAN_POINT('Ctrl Pts',(1.10706451622527E-8,-0.0181073676948121,
-0.00910235328657803));
#14647=CARTESIAN_POINT('Ctrl Pts',(-0.000401979955621974,-0.0181281955922476,
-0.00910235183861967));
#14648=CARTESIAN_POINT('Ctrl Pts',(-0.000804358317651879,-0.0181490315443514,
-0.00918229815991824));
#14649=CARTESIAN_POINT('Ctrl Pts',(-0.00117616985844715,-0.0181698779590349,
-0.00933630636599481));
#14650=CARTESIAN_POINT('Ctrl Pts',(-0.00154798139924243,-0.0181907243737183,
-0.00949031457207138));
#14651=CARTESIAN_POINT('Ctrl Pts',(-0.00188889766670545,-0.0182115812509814,
-0.00971816659367328));
#14652=CARTESIAN_POINT('Ctrl Pts',(-0.00217328877794405,-0.018232438798651,
-0.0100025566805555));
#14653=CARTESIAN_POINT('Ctrl Pts',(-0.00231548433356335,-0.0182428675724858,
-0.0101447517239966));
#14654=CARTESIAN_POINT('Ctrl Pts',(-0.00244369725231803,-0.0182532965139223,
-0.0103009513223182));
#14655=CARTESIAN_POINT('Ctrl Pts',(-0.00255551954698984,-0.0182637381842315,
-0.0104683047235729));
#14656=CARTESIAN_POINT('Ctrl Pts',(-0.00266734184166164,-0.0182741798545408,
-0.0106356581248275));
#14657=CARTESIAN_POINT('Ctrl Pts',(-0.00276272283879781,-0.018284634253723,
-0.0108142141603233));
#14658=CARTESIAN_POINT('Ctrl Pts',(-0.00283954268404827,-0.0182950502136605,
-0.0109996732002329));
#14659=CARTESIAN_POINT('Ctrl Pts',(-0.00291636252929872,-0.0183054661735979,
-0.0111851322401425));
#14660=CARTESIAN_POINT('Ctrl Pts',(-0.00297487762643972,-0.0183158436942908,
-0.0113773322729812));
#14661=CARTESIAN_POINT('Ctrl Pts',(-0.00301444328935122,-0.0183263748869377,
-0.0115762418246218));
#14662=CARTESIAN_POINT('Ctrl Pts',(-0.00303422612080698,-0.0183316404832612,
-0.0116756966004421));
#14663=CARTESIAN_POINT('Ctrl Pts',(-0.00304907659667239,-0.0183369444975732,
-0.0117768871638611));
#14664=CARTESIAN_POINT('Ctrl Pts',(-0.00305870018960846,-0.0183420419650195,
-0.0118745969171828));
#14665=CARTESIAN_POINT('Ctrl Pts',(-0.0030635119860765,-0.0183445906987426,
-0.0119234517938437));
#14666=CARTESIAN_POINT('Ctrl Pts',(-0.00306716319515293,-0.0183470877957494,
-0.0119714145937676));
#14667=CARTESIAN_POINT('Ctrl Pts',(-0.00306979781767152,-0.0183498766894212,
-0.0120250434439775));
#14668=CARTESIAN_POINT('Ctrl Pts',(-0.0030724324401901,-0.018352665583093,
-0.0120786722941874));
#14669=CARTESIAN_POINT('Ctrl Pts',(-0.0030735,-0.0183557462734298,-0.0121380003223703));
#14670=CARTESIAN_POINT('Ctrl Pts',(-0.0030735,-0.0183577122040634,-0.0121758532865577));
#14671=CARTESIAN_POINT('Ctrl Pts',(-0.00307350000000001,-0.0183596781346969,
-0.0122137062507451));
#14672=CARTESIAN_POINT('Ctrl Pts',(-0.00307310376848221,-0.0183605293056272,
-0.0122300919653714));
#14673=CARTESIAN_POINT('Ctrl Pts',(-0.0030725419671156,-0.0183616976447121,
-0.0122525873097381));
#14674=CARTESIAN_POINT('Ctrl Pts',(-0.003071980165749,-0.0183628659837971,
-0.0122750826541048));
#14675=CARTESIAN_POINT('Ctrl Pts',(-0.00307096835910987,-0.0183643514910369,
-0.0123036761037775));
#14676=CARTESIAN_POINT('Ctrl Pts',(-0.00306955009680357,-0.0183658045381892,
-0.0123316238011403));
#14677=CARTESIAN_POINT('Ctrl Pts',(-0.00306671357219098,-0.0183687106324938,
-0.0123875191958658));
#14678=CARTESIAN_POINT('Ctrl Pts',(-0.00306256243770937,-0.0183714868864489,
-0.0124408581493612));
#14679=CARTESIAN_POINT('Ctrl Pts',(-0.00305674327724998,-0.0183743826836283,
-0.0124963572443917));
#14680=CARTESIAN_POINT('Ctrl Pts',(-0.00304510495633122,-0.0183801742779871,
-0.0126073554344527));
#14681=CARTESIAN_POINT('Ctrl Pts',(-0.00302633139541316,-0.018386444045243,
-0.0127269199041359));
#14682=CARTESIAN_POINT('Ctrl Pts',(-0.00299862041661768,-0.0183929964084466,
-0.0128501513267774));
#14683=CARTESIAN_POINT('Ctrl Pts',(-0.0029709094378222,-0.0183995487716502,
-0.0129733827494189));
#14684=CARTESIAN_POINT('Ctrl Pts',(-0.0029344247030508,-0.0184063837308014,
-0.0131003379592189));
#14685=CARTESIAN_POINT('Ctrl Pts',(-0.00288699201251265,-0.0184135533785181,
-0.0132302153542029));
#14686=CARTESIAN_POINT('Ctrl Pts',(-0.0028395593219745,-0.0184207230262348,
-0.0133600927491869));
#14687=CARTESIAN_POINT('Ctrl Pts',(-0.00278113531337715,-0.018428227362517,
-0.0134928631967346));
#14688=CARTESIAN_POINT('Ctrl Pts',(-0.00270984678779956,-0.018436053593843,
-0.0136260714207201));
#14689=CARTESIAN_POINT('Ctrl Pts',(-0.00256726973664439,-0.0184517060564951,
-0.0138924878686913));
#14690=CARTESIAN_POINT('Ctrl Pts',(-0.00237306306717248,-0.0184686460993229,
-0.0141605357837572));
#14691=CARTESIAN_POINT('Ctrl Pts',(-0.00211788429611001,-0.0184868837602526,
-0.0144031764239341));
#14692=CARTESIAN_POINT('Ctrl Pts',(-0.00186270552504755,-0.0185051214211823,
-0.0146458170641111));
#14693=CARTESIAN_POINT('Ctrl Pts',(-0.00154608949796055,-0.018524656700214,
-0.0148624700046778));
#14694=CARTESIAN_POINT('Ctrl Pts',(-0.00117424541782602,-0.0185454869076755,
-0.0150161965666414));
#14695=CARTESIAN_POINT('Ctrl Pts',(-0.000802401337691485,-0.018566317115137,
-0.0151699231286051));
#14696=CARTESIAN_POINT('Ctrl Pts',(-0.000374985873875508,-0.0185884422510285,
-0.0152597732637985));
#14697=CARTESIAN_POINT('Ctrl Pts',(7.73909019784573E-5,-0.0186118630361116,
-0.0152483787784444));
#14698=CARTESIAN_POINT('Ctrl Pts',(0.00052976767783242,-0.0186352838211947,
-0.0152369842930902));
#14699=CARTESIAN_POINT('Ctrl Pts',(0.00100698173546338,-0.0186600002554696,
-0.0151229073790469));
#14700=CARTESIAN_POINT('Ctrl Pts',(0.00145022863864532,-0.018686012145561,
-0.0148856944526881));
#14701=CARTESIAN_POINT('Ctrl Pts',(0.00189347554182726,-0.0187120240356524,
-0.0146484815263293));
#14702=CARTESIAN_POINT('Ctrl Pts',(0.00230162808382228,-0.0187393313815604,
-0.014286383187642));
#14703=CARTESIAN_POINT('Ctrl Pts',(0.00259715510412251,-0.0187679342360236,
-0.0138193822991193));
#14704=CARTESIAN_POINT('Ctrl Pts',(0.00287285221500992,-0.0187946178344663,
-0.0133837172434613));
#14705=CARTESIAN_POINT('Ctrl Pts',(0.00304908377064998,-0.0188224289167476,
-0.012855992906357));
#14706=CARTESIAN_POINT('Ctrl Pts',(0.00307111645156604,-0.0188513674685947,
-0.0122968739084389));
#14707=CARTESIAN_POINT('Ctrl Pts',(0.00307270096662869,-0.0188534486302775,
-0.0122566639822211));
#14708=CARTESIAN_POINT('Ctrl Pts',(0.0030735000947714,-0.0188555356232268,
-0.0122163109465063));
#14709=CARTESIAN_POINT('Ctrl Pts',(0.00307349999999157,-0.0188576284474371,
-0.012175846087576));
#14710=CARTESIAN_POINT('',(0.00307349999999759,-0.0198577587605502,-0.0121758571382905));
#14711=CARTESIAN_POINT('Ctrl Pts',(0.00307349881402483,-0.0188577676402129,
-0.0121731532517477));
#14712=CARTESIAN_POINT('Ctrl Pts',(0.00307300071011293,-0.018887132482759,
-0.0116061524943504));
#14713=CARTESIAN_POINT('Ctrl Pts',(0.00291130029165572,-0.0189164973253051,
-0.0110391550281488));
#14714=CARTESIAN_POINT('Ctrl Pts',(0.00261276553606138,-0.0189458621678513,
-0.0105572555899176));
#14715=CARTESIAN_POINT('Ctrl Pts',(0.00248770402422934,-0.0189581636219859,
-0.01035537935552));
#14716=CARTESIAN_POINT('Ctrl Pts',(0.00233925310066207,-0.0189704650761205,
-0.010168264828373));
#14717=CARTESIAN_POINT('Ctrl Pts',(0.0021716218292663,-0.0189827665302551,
-0.0100008910154706));
#14718=CARTESIAN_POINT('Ctrl Pts',(0.0017788404149206,-0.0190115904037082,
-0.00960871285915861));
#14719=CARTESIAN_POINT('Ctrl Pts',(0.00127519655609348,-0.0190404142771613,
-0.00932444800617673));
#14720=CARTESIAN_POINT('Ctrl Pts',(0.000734339809416652,-0.0190692381506144,
-0.0091913688596753));
#14721=CARTESIAN_POINT('Ctrl Pts',(0.00049336209149727,-0.019082080573842,
-0.00913207569337273));
#14722=CARTESIAN_POINT('Ctrl Pts',(0.000245384423439502,-0.0190949229970696,
-0.00910219102134657));
#14723=CARTESIAN_POINT('Ctrl Pts',(-2.02406328883577E-6,-0.0191077654202972,
-0.00910235395303485));
#14724=CARTESIAN_POINT('Ctrl Pts',(-0.00055936788590402,-0.0191366958961591,
-0.00910272099367752));
#14725=CARTESIAN_POINT('Ctrl Pts',(-0.00111845823087898,-0.019165626372021,
-0.009259024171689));
#14726=CARTESIAN_POINT('Ctrl Pts',(-0.00159613540464352,-0.0191945568478828,
-0.00954930535818452));
#14727=CARTESIAN_POINT('Ctrl Pts',(-0.00180641922172863,-0.0192072926687017,
-0.00967709341103036));
#14728=CARTESIAN_POINT('Ctrl Pts',(-0.00200108197151192,-0.0192200284895205,
-0.00983016017137237));
#14729=CARTESIAN_POINT('Ctrl Pts',(-0.00217448460178119,-0.0192327643103394,
-0.0100037531584294));
#14730=CARTESIAN_POINT('Ctrl Pts',(-0.00256830904193374,-0.0192616893473823,
-0.0103980099285603));
#14731=CARTESIAN_POINT('Ctrl Pts',(-0.00285314591010015,-0.0192906143844251,
-0.0109037395292233));
#14732=CARTESIAN_POINT('Ctrl Pts',(-0.00298573909953144,-0.019319539421468,
-0.0114466315921954));
#14733=CARTESIAN_POINT('Ctrl Pts',(-0.00304414539475079,-0.0193322806811059,
-0.011685771432169));
#14734=CARTESIAN_POINT('Ctrl Pts',(-0.00307360736477033,-0.0193450219407437,
-0.0119317475467586));
#14735=CARTESIAN_POINT('Ctrl Pts',(-0.00307349970435152,-0.0193577632003816,
-0.0121772013782274));
#14736=CARTESIAN_POINT('Ctrl Pts',(-0.00307325529511013,-0.0193866882374244,
-0.0127344273801568));
#14737=CARTESIAN_POINT('Ctrl Pts',(-0.00291713891682898,-0.0194156132744673,
-0.0132934530596749));
#14738=CARTESIAN_POINT('Ctrl Pts',(-0.0026270644627302,-0.0194445383115101,
-0.013771138389184));
#14739=CARTESIAN_POINT('Ctrl Pts',(-0.00249928886373934,-0.019457279571148,
-0.0139815551571714));
#14740=CARTESIAN_POINT('Ctrl Pts',(-0.0023462072838056,-0.0194700208307859,
-0.0141763452408011));
#14741=CARTESIAN_POINT('Ctrl Pts',(-0.00217257832192293,-0.0194827620904237,
-0.0143498601138497));
#14742=CARTESIAN_POINT('Ctrl Pts',(-0.0017783340608814,-0.0195116925662856,
-0.0147438453232469));
#14743=CARTESIAN_POINT('Ctrl Pts',(-0.00127255879685045,-0.0195406230421475,
-0.0150288213855679));
#14744=CARTESIAN_POINT('Ctrl Pts',(-0.000729580226654389,-0.0195695535180093,
-0.0151615047971793));
#14745=CARTESIAN_POINT('Ctrl Pts',(-0.000490549323342851,-0.0195822893388282,
-0.0152199149029787));
#14746=CARTESIAN_POINT('Ctrl Pts',(-0.000244682725290316,-0.019595025159647,
-0.0152494068678258));
#14747=CARTESIAN_POINT('Ctrl Pts',(6.72119984720121E-7,-0.0196077609804659,
-0.0152493532130677));
#14748=CARTESIAN_POINT('Ctrl Pts',(0.000555962360944095,-0.019636584853919,
-0.0152492317809294));
#14749=CARTESIAN_POINT('Ctrl Pts',(0.00111323264387907,-0.0196654087273722,
-0.0150942859026573));
#14750=CARTESIAN_POINT('Ctrl Pts',(0.00158983623043085,-0.0196942326008253,
-0.0148062188524841));
#14751=CARTESIAN_POINT('Ctrl Pts',(0.00180218607231614,-0.0197070750240529,
-0.0146778711138546));
#14752=CARTESIAN_POINT('Ctrl Pts',(0.00199867926914927,-0.0197199174472805,
-0.014523797397214));
#14753=CARTESIAN_POINT('Ctrl Pts',(0.00217352894764179,-0.0197327598705081,
-0.0143489096971842));
#14754=CARTESIAN_POINT('Ctrl Pts',(0.00257333147611902,-0.0197621247130542,
-0.0139490202305618));
#14755=CARTESIAN_POINT('Ctrl Pts',(0.00286070034265989,-0.0197914895556003,
-0.0134347647981465));
#14756=CARTESIAN_POINT('Ctrl Pts',(0.00299117167179052,-0.0198208543981464,
-0.0128824608720523));
#14757=CARTESIAN_POINT('Ctrl Pts',(0.00304582842905604,-0.019833155852281,
-0.012651090947131));
#14758=CARTESIAN_POINT('Ctrl Pts',(0.00307349970232731,-0.0198454573064156,
-0.012413383918551));
#14759=CARTESIAN_POINT('Ctrl Pts',(0.00307349999999759,-0.0198577587605502,
-0.0121758571382905));
#14760=CARTESIAN_POINT('',(0.00307349938939493,-0.0208578413935592,-0.0121772072451699));
#14761=CARTESIAN_POINT('Ctrl Pts',(0.00307349999548701,-0.0198577676402129,
-0.0121756867291843));
#14762=CARTESIAN_POINT('Ctrl Pts',(0.00307346926887639,-0.0198871331262766,
-0.0116086854885077));
#14763=CARTESIAN_POINT('Ctrl Pts',(0.00291223613639999,-0.0199164986123403,
-0.0110415547028757));
#14764=CARTESIAN_POINT('Ctrl Pts',(0.00261409846967682,-0.019945864098404,
-0.010559409213652));
#14765=CARTESIAN_POINT('Ctrl Pts',(0.00248920881946095,-0.019958165279007,
-0.0103574388213693));
#14766=CARTESIAN_POINT('Ctrl Pts',(0.00234091965474288,-0.0199704664596099,
-0.010170209557073));
#14767=CARTESIAN_POINT('Ctrl Pts',(0.00217343535246285,-0.0199827676402129,
-0.0100027032644324));
#14768=CARTESIAN_POINT('Ctrl Pts',(0.00178098080283119,-0.0200115921582588,
-0.00961019718628788));
#14769=CARTESIAN_POINT('Ctrl Pts',(0.00127757369359316,-0.0200404166763048,
-0.00932551220153036));
#14770=CARTESIAN_POINT('Ctrl Pts',(0.000736827631172451,-0.0200692411943507,
-0.00919198209430787));
#14771=CARTESIAN_POINT('Ctrl Pts',(0.000495909767823558,-0.0200820833429714,
-0.00913249060586174));
#14772=CARTESIAN_POINT('Ctrl Pts',(0.00024796804554989,-0.0200949254915922,
-0.0091023992270146));
#14773=CARTESIAN_POINT('Ctrl Pts',(5.7007540347468E-7,-0.0201077676402129,
-0.00910235333942713));
#14774=CARTESIAN_POINT('Ctrl Pts',(-0.000556774407145435,-0.0201366987614893,
-0.00910224996269499));
#14775=CARTESIAN_POINT('Ctrl Pts',(-0.00111599691584013,-0.0201656298827657,
-0.00925808148757206));
#14776=CARTESIAN_POINT('Ctrl Pts',(-0.00159391916450755,-0.0201945610040421,
-0.00954795984370019));
#14777=CARTESIAN_POINT('Ctrl Pts',(-0.00180430162541425,-0.0202072965494324,
-0.00967556495540167));
#14778=CARTESIAN_POINT('Ctrl Pts',(-0.0019990857039826,-0.0202200320948226,
-0.00982845974830203));
#14779=CARTESIAN_POINT('Ctrl Pts',(-0.00217262904748856,-0.0202327676402129,
-0.010001897152684));
#14780=CARTESIAN_POINT('Ctrl Pts',(-0.00256679037826628,-0.0202616933219348,
-0.0103958178686086));
#14781=CARTESIAN_POINT('Ctrl Pts',(-0.00285205908546481,-0.0202906190036567,
-0.0109013045649633));
#14782=CARTESIAN_POINT('Ctrl Pts',(-0.00298511565851904,-0.0203195446853786,
-0.011444083681242));
#14783=CARTESIAN_POINT('Ctrl Pts',(-0.00304372350086436,-0.0203322856703234,
-0.0116831632858417));
#14784=CARTESIAN_POINT('Ctrl Pts',(-0.00307339537122476,-0.0203450266552681,
-0.0119291032718217));
#14785=CARTESIAN_POINT('Ctrl Pts',(-0.00307349972222446,-0.0203577676402129,
-0.0121745465784101));
#14786=CARTESIAN_POINT('Ctrl Pts',(-0.00307373662885434,-0.0203866933219348,
-0.0127317731192086));
#14787=CARTESIAN_POINT('Ctrl Pts',(-0.00291810289228469,-0.0204156190036567,
-0.0132909338655017));
#14788=CARTESIAN_POINT('Ctrl Pts',(-0.00262844071992795,-0.0204445446853786,
-0.0137688698061914));
#14789=CARTESIAN_POINT('Ctrl Pts',(-0.00250085232244247,-0.0204572856703233,
-0.0139793877356718));
#14790=CARTESIAN_POINT('Ctrl Pts',(-0.00234794665639152,-0.0204700266552681,
-0.0141743021870652));
#14791=CARTESIAN_POINT('Ctrl Pts',(-0.00217447679040723,-0.0204827676402129,
-0.0143479612346077));
#14792=CARTESIAN_POINT('Ctrl Pts',(-0.00178057649523043,-0.0205116987614893,
-0.014742291106825));
#14793=CARTESIAN_POINT('Ctrl Pts',(-0.00127504987507543,-0.0205406298827657,
-0.0150277090280041));
#14794=CARTESIAN_POINT('Ctrl Pts',(-0.000732186943210237,-0.0205695610040421,
-0.0151608666081686));
#14795=CARTESIAN_POINT('Ctrl Pts',(-0.000493217445851103,-0.0205822965494324,
-0.0152194828778265));
#14796=CARTESIAN_POINT('Ctrl Pts',(-0.000247387599726067,-0.0205950320948226,
-0.0152491894961984));
#14797=CARTESIAN_POINT('Ctrl Pts',(-2.04334081728397E-6,-0.0206077676402129,
-0.0152493526073256));
#14798=CARTESIAN_POINT('Ctrl Pts',(0.000553247367328469,-0.0206365921582588,
-0.0152497217787654));
#14799=CARTESIAN_POINT('Ctrl Pts',(0.00111065478973551,-0.0206654166763048,
-0.0150952680060627));
#14800=CARTESIAN_POINT('Ctrl Pts',(0.00158751295250971,-0.0206942411943507,
-0.0148076216797899));
#14801=CARTESIAN_POINT('Ctrl Pts',(0.00179996692615825,-0.0207070833429714,
-0.0146794670002799));
#14802=CARTESIAN_POINT('Ctrl Pts',(0.00199658834590345,-0.0207199254915922,
-0.0145255745727847));
#14803=CARTESIAN_POINT('Ctrl Pts',(0.00217158672383872,-0.0207327676402129,
-0.0143508506085903));
#14804=CARTESIAN_POINT('Ctrl Pts',(0.00257174658650591,-0.0207621331262766,
-0.0139513182338244));
#14805=CARTESIAN_POINT('Ctrl Pts',(0.002859574810257,-0.0207914986123403,
-0.013437319424777));
#14806=CARTESIAN_POINT('Ctrl Pts',(0.00299053940595569,-0.020820864098404,
-0.0128851320127484));
#14807=CARTESIAN_POINT('Ctrl Pts',(0.00304540037916721,-0.020833165279007,
-0.0126538211103063));
#14808=CARTESIAN_POINT('Ctrl Pts',(0.0030732839097424,-0.0208454664596099,
-0.0124161495675305));
#14809=CARTESIAN_POINT('Ctrl Pts',(0.00307349874276012,-0.0208577676402129,
-0.0121786332599273));
#14810=CARTESIAN_POINT('',(0.00307349991751608,-0.0218577417662807,-0.0121753484333405));
#14811=CARTESIAN_POINT('Ctrl Pts',(0.00307349999999104,-0.0208579110364346,
-0.0121758607060226));
#14812=CARTESIAN_POINT('Ctrl Pts',(0.00307350136873632,-0.0208872481983145,
-0.0116088604069139));
#14813=CARTESIAN_POINT('Ctrl Pts',(0.002912300834902,-0.0209165870425929,
-0.0110417211748914));
#14814=CARTESIAN_POINT('Ctrl Pts',(0.00261419119460617,-0.020945931248704,
-0.0105595591771697));
#14815=CARTESIAN_POINT('Ctrl Pts',(0.002489269261174,-0.0209582278485684,
-0.0103575106660141));
#14816=CARTESIAN_POINT('Ctrl Pts',(0.00234093045349195,-0.0209705253899725,
-0.010170212365268));
#14817=CARTESIAN_POINT('Ctrl Pts',(0.0021733835198766,-0.0209828241436666,
-0.0100026514262771));
#14818=CARTESIAN_POINT('Ctrl Pts',(0.00178092303245176,-0.0210116326378917,
-0.00961015813278175));
#14819=CARTESIAN_POINT('Ctrl Pts',(0.00127751376905249,-0.0210404477837066,
-0.00932548613589601));
#14820=CARTESIAN_POINT('Ctrl Pts',(0.000736769023118917,-0.0210692591418753,
-0.00919196762243281));
#14821=CARTESIAN_POINT('Ctrl Pts',(0.000495761426462938,-0.0210821002397146,
-0.00913245899792775));
#14822=CARTESIAN_POINT('Ctrl Pts',(0.000247725386902452,-0.0210949405851584,
-0.00910237237716682));
#14823=CARTESIAN_POINT('Ctrl Pts',(2.36968295708491E-7,-0.0211077792539681,
-0.00910235329569328));
#14824=CARTESIAN_POINT('Ctrl Pts',(-0.00055708584513428,-0.021136690841274,
-0.00910231032584208));
#14825=CARTESIAN_POINT('Ctrl Pts',(-0.00111627223786569,-0.0211655939261682,
-0.00925819074347665));
#14826=CARTESIAN_POINT('Ctrl Pts',(-0.00159415131407735,-0.0211945272086743,
-0.00954810066543382));
#14827=CARTESIAN_POINT('Ctrl Pts',(-0.00180461465842751,-0.0212072697531848,
-0.00967578027053203));
#14828=CARTESIAN_POINT('Ctrl Pts',(-0.0019994633841539,-0.0212200181548879,
-0.00982877033427998));
#14829=CARTESIAN_POINT('Ctrl Pts',(-0.00217304838425305,-0.0212327757196597,
-0.0100023163143179));
#14830=CARTESIAN_POINT('Ctrl Pts',(-0.00256719098401647,-0.0212617430828706,
-0.0103963703150181));
#14831=CARTESIAN_POINT('Ctrl Pts',(-0.00285238515458049,-0.0212907576875417,
-0.0109019971240844));
#14832=CARTESIAN_POINT('Ctrl Pts',(-0.00298531443795843,-0.021319675288494,
-0.011444895041159));
#14833=CARTESIAN_POINT('Ctrl Pts',(-0.00304385815732449,-0.0213324109617171,
-0.0116839940755777));
#14834=CARTESIAN_POINT('Ctrl Pts',(-0.00307346370977526,-0.0213451278197905,
-0.0119299475821563));
#14835=CARTESIAN_POINT('Ctrl Pts',(-0.00307349996646892,-0.0213578135407414,
-0.0121753992870766));
#14836=CARTESIAN_POINT('Ctrl Pts',(-0.00307358227467943,-0.0213866120572328,
-0.0127326119988626));
#14837=CARTESIAN_POINT('Ctrl Pts',(-0.00291780077213178,-0.0214152501057386,
-0.0132917289026298));
#14838=CARTESIAN_POINT('Ctrl Pts',(-0.00262800217461437,-0.0214439139712749,
-0.0137695931713016));
#14839=CARTESIAN_POINT('Ctrl Pts',(-0.00250028916401618,-0.0214565460150266,
-0.0139801859241036));
#14840=CARTESIAN_POINT('Ctrl Pts',(-0.00234723536954019,-0.0214691830727747,
-0.0141751538149292));
#14841=CARTESIAN_POINT('Ctrl Pts',(-0.00217360204790616,-0.0214818410884174,
-0.0143488365785643));
#14842=CARTESIAN_POINT('Ctrl Pts',(-0.00177962843165187,-0.0215105620974404,
-0.0147429223786078));
#14843=CARTESIAN_POINT('Ctrl Pts',(-0.00127410374523453,-0.0215393910050567,
-0.0150281122649468));
#14844=CARTESIAN_POINT('Ctrl Pts',(-0.000731298271848334,-0.0215682772307582,
-0.0151610844480583));
#14845=CARTESIAN_POINT('Ctrl Pts',(-0.000492037458318172,-0.0215810098618757,
-0.0152196966660038));
#14846=CARTESIAN_POINT('Ctrl Pts',(-0.000245908898367081,-0.0215937536294333,
-0.0152493304427505));
#14847=CARTESIAN_POINT('Ctrl Pts',(-2.85679979158681E-7,-0.0216065042016624,
-0.0152493532732812));
#14848=CARTESIAN_POINT('Ctrl Pts',(0.000555014508283015,-0.021635330447022,
-0.0152494048881004));
#14849=CARTESIAN_POINT('Ctrl Pts',(0.00111234191860738,-0.0216641914719324,
-0.0150946272716086));
#14850=CARTESIAN_POINT('Ctrl Pts',(0.00158904050890284,-0.0216931009275372,
-0.0148066996353717));
#14851=CARTESIAN_POINT('Ctrl Pts',(0.00180156125657449,-0.021705989279307,
-0.0146783363513719));
#14852=CARTESIAN_POINT('Ctrl Pts',(0.00199821333105363,-0.0217188872568502,
-0.0145242100967846));
#14853=CARTESIAN_POINT('Ctrl Pts',(0.00217319805514847,-0.0217317960697658,
-0.0143492406112425));
#14854=CARTESIAN_POINT('Ctrl Pts',(0.00257305896431553,-0.0217612942427944,
-0.0139494145239813));
#14855=CARTESIAN_POINT('Ctrl Pts',(0.00286050574081673,-0.0217908489956305,
-0.0134352059308452));
#14856=CARTESIAN_POINT('Ctrl Pts',(0.00299106214730737,-0.0218204555171494,
-0.0128829243444759));
#14857=CARTESIAN_POINT('Ctrl Pts',(0.00304579179865083,-0.0218328666629811,
-0.0126514061870918));
#14858=CARTESIAN_POINT('Ctrl Pts',(0.00307350020926293,-0.021845286906188,
-0.0124135380719837));
#14859=CARTESIAN_POINT('Ctrl Pts',(0.00307349999999881,-0.0218577158923484,
-0.0121758505805963));
#14860=CARTESIAN_POINT('',(0.00307349949439479,-0.0228577072780383,-0.01217458316111));
#14861=CARTESIAN_POINT('Ctrl Pts',(0.00307349983503335,-0.0218577676402129,
-0.0121748462860847));
#14862=CARTESIAN_POINT('Ctrl Pts',(0.00307331406363246,-0.0218871263583065,
-0.0116078471782629));
#14863=CARTESIAN_POINT('Ctrl Pts',(0.00291192699341664,-0.0219164850764001,
-0.0110407622690103));
#14864=CARTESIAN_POINT('Ctrl Pts',(0.00261365940606214,-0.0219458437944937,
-0.0105586993795032));
#14865=CARTESIAN_POINT('Ctrl Pts',(0.00248867160359435,-0.0219581464442396,
-0.0103566929136141));
#14866=CARTESIAN_POINT('Ctrl Pts',(0.00234027201046346,-0.0219704490939856,
-0.0101694442405646));
#14867=CARTESIAN_POINT('Ctrl Pts',(0.00217267097699875,-0.0219827517437315,
-0.0100019390574066));
#14868=CARTESIAN_POINT('Ctrl Pts',(0.00178008169618916,-0.0220115695160087,
-0.00960957429671008));
#14869=CARTESIAN_POINT('Ctrl Pts',(0.00127657885878497,-0.022040387288286,
-0.00932506722177673));
#14870=CARTESIAN_POINT('Ctrl Pts',(0.000735789944503822,-0.0220692050605632,
-0.00919172604269481));
#14871=CARTESIAN_POINT('Ctrl Pts',(0.000494769436991987,-0.0220820486561255,
-0.00913229812580182));
#14872=CARTESIAN_POINT('Ctrl Pts',(0.000246730499174395,-0.0220948922516879,
-0.00910229288898429));
#14873=CARTESIAN_POINT('Ctrl Pts',(-7.5122358097326E-7,-0.0221077358472502,
-0.00910235337836497));
#14874=CARTESIAN_POINT('Ctrl Pts',(-0.000558091349644402,-0.0221366602101895,
-0.00910248960320891));
#14875=CARTESIAN_POINT('Ctrl Pts',(-0.00111724334613616,-0.0221655845731287,
-0.00925855919309804));
#14876=CARTESIAN_POINT('Ctrl Pts',(-0.00159503904782892,-0.022194508936068,
-0.00954863942280413));
#14877=CARTESIAN_POINT('Ctrl Pts',(-0.00180543905582782,-0.0222072459409683,
-0.00967637787343116));
#14878=CARTESIAN_POINT('Ctrl Pts',(-0.00200021915344352,-0.0222199829458685,
-0.0098294167504658));
#14879=CARTESIAN_POINT('Ctrl Pts',(-0.00217373341178053,-0.0222327199507688,
-0.0100030014037762));
#14880=CARTESIAN_POINT('Ctrl Pts',(-0.00256769153989136,-0.0222616388802927,
-0.0103971193612416));
#14881=CARTESIAN_POINT('Ctrl Pts',(-0.00285270257510404,-0.0222905578098167,
-0.0109027469575032));
#14882=CARTESIAN_POINT('Ctrl Pts',(-0.00298548448088764,-0.0223194767393406,
-0.0114455898653332));
#14883=CARTESIAN_POINT('Ctrl Pts',(-0.00304399166879977,-0.0223322191776562,
-0.0116847806784771));
#14884=CARTESIAN_POINT('Ctrl Pts',(-0.0030735395388613,-0.0223449616159718,
-0.0119308219663486));
#14885=CARTESIAN_POINT('Ctrl Pts',(-0.00307349996006712,-0.0223577040542874,
-0.0121763487332415));
#14886=CARTESIAN_POINT('Ctrl Pts',(-0.00307341013610005,-0.0223866229838114,
-0.0127335710710829));
#14887=CARTESIAN_POINT('Ctrl Pts',(-0.00291745083476184,-0.0224155419133353,
-0.0132926370849982));
#14888=CARTESIAN_POINT('Ctrl Pts',(-0.00262751193933117,-0.0224444608428593,
-0.013770401265978));
#14889=CARTESIAN_POINT('Ctrl Pts',(-0.00249975726268389,-0.0224572032811749,
-0.0139809166863533));
#14890=CARTESIAN_POINT('Ctrl Pts',(-0.00234667702880692,-0.0224699457194905,
-0.0141758031377059));
#14891=CARTESIAN_POINT('Ctrl Pts',(-0.00217303277351682,-0.0224826881578061,
-0.0143494058659133));
#14892=CARTESIAN_POINT('Ctrl Pts',(-0.00177887356019078,-0.0225116125207454,
-0.0147434708159295));
#14893=CARTESIAN_POINT('Ctrl Pts',(-0.00127316145523074,-0.0225405368836846,
-0.0150285519019311));
#14894=CARTESIAN_POINT('Ctrl Pts',(-0.000730214003843846,-0.0225694612466239,
-0.015161349854734));
#14895=CARTESIAN_POINT('Ctrl Pts',(-0.000491124058685119,-0.0225821982515242,
-0.0152198281755582));
#14896=CARTESIAN_POINT('Ctrl Pts',(-0.000245188176706377,-0.0225949352564245,
-0.0152493724155374));
#14897=CARTESIAN_POINT('Ctrl Pts',(2.39669782465268E-7,-0.0226076722613247,
-0.0152493532772134));
#14898=CARTESIAN_POINT('Ctrl Pts',(0.000555525927892844,-0.0226364900336019,
-0.0152493099763066));
#14899=CARTESIAN_POINT('Ctrl Pts',(0.00111281481403792,-0.0226653078058792,
-0.0150944446411238));
#14900=CARTESIAN_POINT('Ctrl Pts',(0.00158945717892497,-0.0226941255781564,
-0.0148064479201655));
#14901=CARTESIAN_POINT('Ctrl Pts',(0.00180188865015705,-0.0227069691737187,
-0.014678092634001));
#14902=CARTESIAN_POINT('Ctrl Pts',(0.00199845769115906,-0.0227198127692811,
-0.014523993699976));
#14903=CARTESIAN_POINT('Ctrl Pts',(0.00217337173187688,-0.0227326563648434,
-0.0143490669357602));
#14904=CARTESIAN_POINT('Ctrl Pts',(0.00257320151374196,-0.022762015082937,
-0.0139492080697039));
#14905=CARTESIAN_POINT('Ctrl Pts',(0.00286060724971039,-0.0227913738010306,
-0.0134349755781676));
#14906=CARTESIAN_POINT('Ctrl Pts',(0.00299111920455669,-0.0228207325191242,
-0.0128826829365673));
#14907=CARTESIAN_POINT('Ctrl Pts',(0.00304580970102223,-0.0228330351688702,
-0.0126512469826813));
#14908=CARTESIAN_POINT('Ctrl Pts',(0.00307349875478779,-0.0228453378186161,
-0.0124134680443367));
#14909=CARTESIAN_POINT('Ctrl Pts',(0.00307349999995779,-0.022857640468362,
-0.0121758693936782));
#14910=CARTESIAN_POINT('',(0.00307349962338454,-0.0238578241218712,-0.0121769184793798));
#14911=CARTESIAN_POINT('Ctrl Pts',(0.0030734990376214,-0.022857767640213,
-0.0121734210570659));
#14912=CARTESIAN_POINT('Ctrl Pts',(0.00307305033695564,-0.0228871357094251,
-0.0116064182027534));
#14913=CARTESIAN_POINT('Ctrl Pts',(0.00291139821148099,-0.0229165037786371,
-0.0110394049233265));
#14914=CARTESIAN_POINT('Ctrl Pts',(0.00261290357933612,-0.0229458718478492,
-0.0105574784427433));
#14915=CARTESIAN_POINT('Ctrl Pts',(0.00248790164963457,-0.0229581704453038,
-0.0103556599389589));
#14916=CARTESIAN_POINT('Ctrl Pts',(0.00233952495234875,-0.0229704690427584,
-0.0101685910649555));
#14917=CARTESIAN_POINT('Ctrl Pts',(0.0021719776110592,-0.022982767640213,
-0.010001246308951));
#14918=CARTESIAN_POINT('Ctrl Pts',(0.00177925715436449,-0.023011594781079,
-0.00960900069945493));
#14919=CARTESIAN_POINT('Ctrl Pts',(0.0012756555475673,-0.0230404219219451,
-0.00932465262100666));
#14920=CARTESIAN_POINT('Ctrl Pts',(0.000734816597786818,-0.0230692490628111,
-0.0091914862150307));
#14921=CARTESIAN_POINT('Ctrl Pts',(0.000493928481897427,-0.0230820885886117,
-0.00913217428002985));
#14922=CARTESIAN_POINT('Ctrl Pts',(0.000246040397300628,-0.0230949281144124,
-0.0091022500497725));
#14923=CARTESIAN_POINT('Ctrl Pts',(-1.28625627569396E-6,-0.023107767640213,
-0.00910235355570651));
#14924=CARTESIAN_POINT('Ctrl Pts',(-0.000558634401779208,-0.0231367013834657,
-0.0091025868052958));
#14925=CARTESIAN_POINT('Ctrl Pts',(-0.00111776564145458,-0.0231656351267184,
-0.00925875804508432));
#14926=CARTESIAN_POINT('Ctrl Pts',(-0.00159551432548366,-0.0231945688699711,
-0.00954892803311513));
#14927=CARTESIAN_POINT('Ctrl Pts',(-0.00180575803130939,-0.0232073017933851,
-0.00967662365142329));
#14928=CARTESIAN_POINT('Ctrl Pts',(-0.00200039715527956,-0.023220034716799,
-0.00982958467417083));
#14929=CARTESIAN_POINT('Ctrl Pts',(-0.0021737969912177,-0.023232767640213,
-0.0100030650108688));
#14930=CARTESIAN_POINT('Ctrl Pts',(-0.0025677491220947,-0.0232616959392744,
-0.0103972000337635));
#14931=CARTESIAN_POINT('Ctrl Pts',(-0.00285274681297765,-0.0232906242383358,
-0.0109028433512128));
#14932=CARTESIAN_POINT('Ctrl Pts',(-0.00298551070465185,-0.0233195525373972,
-0.011445697082442));
#14933=CARTESIAN_POINT('Ctrl Pts',(-0.00304397232568449,-0.0233322909050025,
-0.0116847388031318));
#14934=CARTESIAN_POINT('Ctrl Pts',(-0.00307351119625606,-0.0233450292726077,
-0.0119306212724117));
#14935=CARTESIAN_POINT('Ctrl Pts',(-0.00307349999679855,-0.0233577676402129,
-0.0121759935694385));
#14936=CARTESIAN_POINT('Ctrl Pts',(-0.00307347456329985,-0.0233866959392743,
-0.0127332237742619));
#14937=CARTESIAN_POINT('Ctrl Pts',(-0.00291757565825456,-0.0234156242383358,
-0.0132923140642119));
#14938=CARTESIAN_POINT('Ctrl Pts',(-0.00262768555746732,-0.0234445525373972,
-0.0137701151411722));
#14939=CARTESIAN_POINT('Ctrl Pts',(-0.00250003454483423,-0.0234572909050024,
-0.013980511395289));
#14940=CARTESIAN_POINT('Ctrl Pts',(-0.00234708845669796,-0.0234700292726077,
-0.0141753013142027));
#14941=CARTESIAN_POINT('Ctrl Pts',(-0.0021735986382546,-0.0234827676402129,
-0.0143488399891814));
#14942=CARTESIAN_POINT('Ctrl Pts',(-0.00177953638323401,-0.0235117013834656,
-0.0147430132162271));
#14943=CARTESIAN_POINT('Ctrl Pts',(-0.00127389095929958,-0.0235406351267183,
-0.0150282274685925));
#14944=CARTESIAN_POINT('Ctrl Pts',(-0.00073097096784502,-0.023569568869971,
-0.0151611646093798));
#14945=CARTESIAN_POINT('Ctrl Pts',(-0.000492047209839665,-0.023582301793385,
-0.0152196664913428));
#14946=CARTESIAN_POINT('Ctrl Pts',(-0.000246278880082321,-0.0235950347167989,
-0.0152492728653299));
#14947=CARTESIAN_POINT('Ctrl Pts',(-1.00569053437863E-6,-0.0236077676402129,
-0.0152493531220204));
#14948=CARTESIAN_POINT('Ctrl Pts',(0.00055428900149266,-0.0236365947810789,
-0.0152495348219213));
#14949=CARTESIAN_POINT('Ctrl Pts',(0.0011116473574554,-0.023665421921945,
-0.0150948907950721));
#14950=CARTESIAN_POINT('Ctrl Pts',(0.00158841008506312,-0.023694249062811,
-0.0148070803105281));
#14951=CARTESIAN_POINT('Ctrl Pts',(0.00180075883551153,-0.0237070885886116,
-0.0146788903468001));
#14952=CARTESIAN_POINT('Ctrl Pts',(0.00199727549648617,-0.0237199281144123,
-0.0145249830204326));
#14953=CARTESIAN_POINT('Ctrl Pts',(0.0021721761119366,-0.0237327676402129,
-0.0143502619852006));
#14954=CARTESIAN_POINT('Ctrl Pts',(0.00257222931168367,-0.023762135709425,
-0.0139506195423898));
#14955=CARTESIAN_POINT('Ctrl Pts',(0.00285991854711518,-0.023791503778637,
-0.0134365406511251));
#14956=CARTESIAN_POINT('Ctrl Pts',(0.00299073283294949,-0.0238208718478491,
-0.0128843159686508));
#14957=CARTESIAN_POINT('Ctrl Pts',(0.00304551451543502,-0.0238331704453037,
-0.0126530583730217));
#14958=CARTESIAN_POINT('Ctrl Pts',(0.00307333301785099,-0.0238454690427583,
-0.0124154512831565));
#14959=CARTESIAN_POINT('Ctrl Pts',(0.00307349924684273,-0.0238577676402129,
-0.0121780049503674));
#14960=CARTESIAN_POINT('',(0.00307349967665051,-0.0248577676402129,-0.012177263119607));
#14961=CARTESIAN_POINT('Ctrl Pts',(0.00307349999992634,-0.0238578806035296,
-0.0121758320083923));
#14962=CARTESIAN_POINT('Ctrl Pts',(0.00307349607452821,-0.0238872403822584,
-0.0116088324239896));
#14963=CARTESIAN_POINT('Ctrl Pts',(0.00291229064502768,-0.0239166001609873,
-0.0110416954096486));
#14964=CARTESIAN_POINT('Ctrl Pts',(0.00261417727345869,-0.0239459599397161,
-0.0105595366613475));
#14965=CARTESIAN_POINT('Ctrl Pts',(0.0024892633655894,-0.0239582621208491,
-0.0103575050210133));
#14966=CARTESIAN_POINT('Ctrl Pts',(0.00234093639568344,-0.0239705643019821,
-0.0101702214871738));
#14967=CARTESIAN_POINT('Ctrl Pts',(0.0021734041367439,-0.023982866483115,
-0.0100026720450634));
#14968=CARTESIAN_POINT('Ctrl Pts',(0.00178094653157099,-0.0240116853182242,
-0.00961017418694974));
#14969=CARTESIAN_POINT('Ctrl Pts',(0.00127753876572544,-0.0240405041533333,
-0.00932549710950571));
#14970=CARTESIAN_POINT('Ctrl Pts',(0.000736793995285274,-0.0240693229884425,
-0.00919197378857036));
#14971=CARTESIAN_POINT('Ctrl Pts',(0.000495810884073522,-0.0240821661131951,
-0.00913246907015739));
#14972=CARTESIAN_POINT('Ctrl Pts',(0.000247800461736436,-0.0240950092379478,
-0.00910238039836973));
#14973=CARTESIAN_POINT('Ctrl Pts',(3.36499649636908E-7,-0.0241078523627004,
-0.00910235330497879));
#14974=CARTESIAN_POINT('Ctrl Pts',(-0.00055700456237791,-0.0241367777897768,
-0.00910229228494521));
#14975=CARTESIAN_POINT('Ctrl Pts',(-0.00111621249341672,-0.0241657032168533,
-0.00925816447319608));
#14976=CARTESIAN_POINT('Ctrl Pts',(-0.00159411122558648,-0.0241946286439297,
-0.00954807634578493));
#14977=CARTESIAN_POINT('Ctrl Pts',(-0.00180454106139394,-0.0242073651767151,
-0.00967573123089108));
#14978=CARTESIAN_POINT('Ctrl Pts',(-0.00199936220140598,-0.0242201017095004,
-0.00982868836518448));
#14979=CARTESIAN_POINT('Ctrl Pts',(-0.00217292822667836,-0.0242328382422858,
-0.010002196190394));
#14980=CARTESIAN_POINT('Ctrl Pts',(-0.00256703298197344,-0.024261758234714,
-0.0103961687947023));
#14981=CARTESIAN_POINT('Ctrl Pts',(-0.00285223149793234,-0.0242906782271423,
-0.0109016916062154));
#14982=CARTESIAN_POINT('Ctrl Pts',(-0.00298521427273911,-0.0243195982195706,
-0.0114444860765776));
#14983=CARTESIAN_POINT('Ctrl Pts',(-0.00304380564996769,-0.0243323401870041,
-0.0116836379187375));
#14984=CARTESIAN_POINT('Ctrl Pts',(-0.00307344446317736,-0.0243450821544377,
-0.0119296499451585));
#14985=CARTESIAN_POINT('Ctrl Pts',(-0.00307349992158432,-0.0243578241218712,
-0.0121751590090976));
#14986=CARTESIAN_POINT('Ctrl Pts',(-0.00307362579356741,-0.0243867441142995,
-0.0127323822406914));
#14987=CARTESIAN_POINT('Ctrl Pts',(-0.00291788243124792,-0.0244156641067277,
-0.0132915093003472));
#14988=CARTESIAN_POINT('Ctrl Pts',(-0.00262812776063055,-0.0244445840991559,
-0.0137693860674581));
#14989=CARTESIAN_POINT('Ctrl Pts',(-0.00250046366853621,-0.0244573260665895,
-0.0139799355763797));
#14990=CARTESIAN_POINT('Ctrl Pts',(-0.00234747167256663,-0.0244700680340231,
-0.0141748681784755));
#14991=CARTESIAN_POINT('Ctrl Pts',(-0.0021739100261297,-0.0244828100014566,
-0.0143485284689756));
#14992=CARTESIAN_POINT('Ctrl Pts',(-0.00177990927440443,-0.0245117354285331,
-0.0147427531517122));
#14993=CARTESIAN_POINT('Ctrl Pts',(-0.00127431142674241,-0.0245406608556095,
-0.0150280385348234));
#14994=CARTESIAN_POINT('Ctrl Pts',(-0.000731416810373939,-0.024569586282686,
-0.0151610554069349));
#14995=CARTESIAN_POINT('Ctrl Pts',(-0.000492367787447086,-0.0245823228154714,
-0.0152196258041213));
#14996=CARTESIAN_POINT('Ctrl Pts',(-0.0002464621685526,-0.0245950593482567,
-0.0152492691029153));
#14997=CARTESIAN_POINT('Ctrl Pts',(-1.05205526183687E-6,-0.0246077958810421,
-0.0152493531064995));
#14998=CARTESIAN_POINT('Ctrl Pts',(0.000554235141673008,-0.0246366147161513,
-0.0152495431806337));
#14999=CARTESIAN_POINT('Ctrl Pts',(0.00111158984035125,-0.0246654335512604,
-0.0150949115582599));
#15000=CARTESIAN_POINT('Ctrl Pts',(0.0015883536267387,-0.0246942523863696,
-0.0148071143922688));
#15001=CARTESIAN_POINT('Ctrl Pts',(0.00180082358823867,-0.0247070955111222,
-0.0146788574765302));
#15002=CARTESIAN_POINT('Ctrl Pts',(0.00199744422213352,-0.0247199386358749,
-0.0145248539977468));
#15003=CARTESIAN_POINT('Ctrl Pts',(0.00217242210871539,-0.0247327817606275,
-0.0143500162131955));
#15004=CARTESIAN_POINT('Ctrl Pts',(0.00257242694643423,-0.0247621415393563,
-0.0139503316530336));
#15005=CARTESIAN_POINT('Ctrl Pts',(0.00286005738988455,-0.0247915013180852,
-0.0134362242481947));
#15006=CARTESIAN_POINT('Ctrl Pts',(0.00299081045101602,-0.024820861096814,
-0.0128839882285666));
#15007=CARTESIAN_POINT('Ctrl Pts',(0.00304559791575083,-0.024833163277947,
-0.0126525931760236));
#15008=CARTESIAN_POINT('Ctrl Pts',(0.00307339069671438,-0.0248454654590799,
-0.0124148442989605));
#15009=CARTESIAN_POINT('Ctrl Pts',(0.00307349967665051,-0.0248577676402129,
-0.012177263119607));
#15010=CARTESIAN_POINT('',(0.00307349906472614,-0.0258577432759482,-0.0121736790431998));
#15011=CARTESIAN_POINT('Ctrl Pts',(0.00307349999999773,-0.0248578401021784,
-0.0121758570261513));
#15012=CARTESIAN_POINT('Ctrl Pts',(0.00307350068537023,-0.0248869104153856,
-0.0116125624938714));
#15013=CARTESIAN_POINT('Ctrl Pts',(0.00291433569470665,-0.0249159966875591,
-0.0110488238096736));
#15014=CARTESIAN_POINT('Ctrl Pts',(0.00261987280316784,-0.0249450991055997,
-0.010568784916755));
#15015=CARTESIAN_POINT('Ctrl Pts',(0.00249371145037095,-0.0249575679107875,
-0.0103631143284876));
#15016=CARTESIAN_POINT('Ctrl Pts',(0.00234336379447851,-0.0249700396798027,
-0.0101726336832762));
#15017=CARTESIAN_POINT('Ctrl Pts',(0.00217330538285328,-0.0249825144273446,
-0.0100025732855318));
#15018=CARTESIAN_POINT('Ctrl Pts',(0.00177902926068591,-0.0250114368137107,
-0.00960829255859728));
#15019=CARTESIAN_POINT('Ctrl Pts',(0.00127275405917176,-0.0250403752106253,
-0.00932273579918919));
#15020=CARTESIAN_POINT('Ctrl Pts',(0.000728558695200731,-0.0250693290685143,
-0.00918995233748972));
#15021=CARTESIAN_POINT('Ctrl Pts',(0.000490182471258236,-0.0250820118507816,
-0.0091317886295688));
#15022=CARTESIAN_POINT('Ctrl Pts',(0.000244909984473728,-0.0250946975996085,
-0.00910235423995953));
#15023=CARTESIAN_POINT('Ctrl Pts',(1.19650119577734E-8,-0.0251073862688045,
-0.00910235328658139));
#15024=CARTESIAN_POINT('Ctrl Pts',(-0.000401979116139882,-0.0251282142520593,
-0.00910235172164627));
#15025=CARTESIAN_POINT('Ctrl Pts',(-0.000804358817299954,-0.0251490501039609,
-0.00918229846194574));
#15026=CARTESIAN_POINT('Ctrl Pts',(-0.00117616923873007,-0.0251698958673943,
-0.00933630610930164));
#15027=CARTESIAN_POINT('Ctrl Pts',(-0.00154797966016019,-0.0251907416308277,
-0.00949031375665754));
#15028=CARTESIAN_POINT('Ctrl Pts',(-0.00188889080179529,-0.025211597305793,
-0.00971815981154555));
#15029=CARTESIAN_POINT('Ctrl Pts',(-0.00217328846173606,-0.0252324545845573,
-0.0100025563643487));
#15030=CARTESIAN_POINT('Ctrl Pts',(-0.00231548729170644,-0.0252428832239394,
-0.0101447546407502));
#15031=CARTESIAN_POINT('Ctrl Pts',(-0.00244370560832201,-0.0252533122642713,
-0.0103009638674558));
#15032=CARTESIAN_POINT('Ctrl Pts',(-0.00255551936065739,-0.0252637523626038,
-0.0104683044447075));
#15033=CARTESIAN_POINT('Ctrl Pts',(-0.00266733311299277,-0.0252741924609363,
-0.0106356450219593));
#15034=CARTESIAN_POINT('Ctrl Pts',(-0.00276269865287568,-0.0252846436172694,
-0.0108141558086635));
#15035=CARTESIAN_POINT('Ctrl Pts',(-0.00283954259848281,-0.0252950624202936,
-0.0109996729936602));
#15036=CARTESIAN_POINT('Ctrl Pts',(-0.00291638654408995,-0.0253054812233178,
-0.0111851901786568));
#15037=CARTESIAN_POINT('Ctrl Pts',(-0.00297492629622829,-0.0253158676730331,
-0.011377576989722));
#15038=CARTESIAN_POINT('Ctrl Pts',(-0.00301444326754076,-0.0253263847576267,
-0.0115762417149734));
#15039=CARTESIAN_POINT('Ctrl Pts',(-0.00303420175319699,-0.0253316432999235,
-0.0116755740775992));
#15040=CARTESIAN_POINT('Ctrl Pts',(-0.0030490409528902,-0.0253369345009398,
-0.0117765252855877));
#15041=CARTESIAN_POINT('Ctrl Pts',(-0.00305870018412946,-0.0253420505311595,
-0.0118745968615537));
#15042=CARTESIAN_POINT('Ctrl Pts',(-0.00306352979974909,-0.0253446085462694,
-0.0119236326495368));
#15043=CARTESIAN_POINT('Ctrl Pts',(-0.00306718850569586,-0.02534712276868,
-0.0119719298103766));
#15044=CARTESIAN_POINT('Ctrl Pts',(-0.00306979781630011,-0.0253498845691424,
-0.012025043416062));
#15045=CARTESIAN_POINT('Ctrl Pts',(-0.00307240712690437,-0.0253526463696048,
-0.0120781570217473));
#15046=CARTESIAN_POINT('Ctrl Pts',(-0.0030735,-0.025355655748119,-0.012136115688322));
#15047=CARTESIAN_POINT('Ctrl Pts',(-0.0030735,-0.0253577193746031,-0.0121758532865577));
#15048=CARTESIAN_POINT('Ctrl Pts',(-0.00307350000000001,-0.0253597830010872,
-0.0122155908847934));
#15049=CARTESIAN_POINT('Ctrl Pts',(-0.00307300554522283,-0.0253609008755414,
-0.0122371133043084));
#15050=CARTESIAN_POINT('Ctrl Pts',(-0.00307224100675227,-0.025362287812272,
-0.0122638160424823));
#15051=CARTESIAN_POINT('Ctrl Pts',(-0.00307147646828171,-0.0253636747490026,
-0.0122905187806561));
#15052=CARTESIAN_POINT('Ctrl Pts',(-0.00307016498421063,-0.0253653307480096,
-0.0123223895170306));
#15053=CARTESIAN_POINT('Ctrl Pts',(-0.0030683501683386,-0.0253669591928204,
-0.0123537001151958));
#15054=CARTESIAN_POINT('Ctrl Pts',(-0.00306472053659454,-0.0253702160824419,
-0.0124163213115264));
#15055=CARTESIAN_POINT('Ctrl Pts',(-0.00305937780406044,-0.0253733627552782,
-0.012476730769819));
#15056=CARTESIAN_POINT('Ctrl Pts',(-0.00305198487235182,-0.0253766107825558,
-0.0125388830221662));
#15057=CARTESIAN_POINT('Ctrl Pts',(-0.00303719900893458,-0.0253831068371111,
-0.0126631875268605));
#15058=CARTESIAN_POINT('Ctrl Pts',(-0.00301376367080274,-0.0253900083094319,
-0.0127943819767643));
#15059=CARTESIAN_POINT('Ctrl Pts',(-0.0029800853608862,-0.0253971492765809,
-0.0129278462997116));
#15060=CARTESIAN_POINT('Ctrl Pts',(-0.00294640705096966,-0.0254042902437299,
-0.013061310622659));
#15061=CARTESIAN_POINT('Ctrl Pts',(-0.00290263545605546,-0.0254116707057071,
-0.0131971045166008));
#15062=CARTESIAN_POINT('Ctrl Pts',(-0.00284694205880417,-0.0254193348566784,
-0.0133340083555415));
#15063=CARTESIAN_POINT('Ctrl Pts',(-0.00279124866155287,-0.0254269990076497,
-0.0134709121944821));
#15064=CARTESIAN_POINT('Ctrl Pts',(-0.00272359546920565,-0.0254349468476151,
-0.0136088948852597));
#15065=CARTESIAN_POINT('Ctrl Pts',(-0.00264256792344005,-0.0254431675228483,
-0.0137453235857373));
#15066=CARTESIAN_POINT('Ctrl Pts',(-0.00248051283190884,-0.0254596088733148,
-0.0140181809866926));
#15067=CARTESIAN_POINT('Ctrl Pts',(-0.00226469144760116,-0.0254771415648527,
-0.014284636089567));
#15068=CARTESIAN_POINT('Ctrl Pts',(-0.00199062313410204,-0.0254957741134054,
-0.0145176094198858));
#15069=CARTESIAN_POINT('Ctrl Pts',(-0.00171655482060292,-0.025514406661958,
-0.0147505827502045));
#15070=CARTESIAN_POINT('Ctrl Pts',(-0.00138383681775807,-0.0255341390675254,
-0.0149495290333914));
#15071=CARTESIAN_POINT('Ctrl Pts',(-0.00100354630252485,-0.0255549690482522,
-0.0150809001138379));
#15072=CARTESIAN_POINT('Ctrl Pts',(-0.000623255787291618,-0.025575799028979,
-0.0152122711942845));
#15073=CARTESIAN_POINT('Ctrl Pts',(-0.000195143521376919,-0.0255977265848653,
-0.015275248483919));
#15074=CARTESIAN_POINT('Ctrl Pts',(0.000248294841224699,-0.0256207523273886,
-0.0152393075332902));
#15075=CARTESIAN_POINT('Ctrl Pts',(0.000691733203826318,-0.0256437780699119,
-0.0152033665826615));
#15076=CARTESIAN_POINT('Ctrl Pts',(0.00115034288718135,-0.0256679019990723,
-0.01506735112295));
#15077=CARTESIAN_POINT('Ctrl Pts',(0.00156948119630631,-0.0256931239508147,
-0.0148184147379611));
#15078=CARTESIAN_POINT('Ctrl Pts',(0.00198861950543127,-0.0257183459025571,
-0.0145694783529722));
#15079=CARTESIAN_POINT('Ctrl Pts',(0.00236737253616329,-0.0257446658768816,
-0.0142063008048711));
#15080=CARTESIAN_POINT('Ctrl Pts',(0.00263898767146668,-0.0257720839185305,
-0.013751336171215));
#15081=CARTESIAN_POINT('Ctrl Pts',(0.00291059991413796,-0.0257995016681841,
-0.0132963763828165));
#15082=CARTESIAN_POINT('Ctrl Pts',(0.00307350131380818,-0.025828017461774,
-0.0127485450022714));
#15083=CARTESIAN_POINT('Ctrl Pts',(0.00307349999999191,-0.0258576312843864,
-0.012175846235706));
#15084=CARTESIAN_POINT('',(0.00307349999999503,-0.0268577565897941,-0.0121758588150803));
#15085=CARTESIAN_POINT('Ctrl Pts',(0.0030734988612549,-0.0258577676402129,
-0.0121732075607849));
#15086=CARTESIAN_POINT('Ctrl Pts',(0.00307301077635369,-0.0258871323359906,
-0.0116062068522265));
#15087=CARTESIAN_POINT('Ctrl Pts',(0.00291132040796627,-0.0259164970317683,
-0.0110392065771651));
#15088=CARTESIAN_POINT('Ctrl Pts',(0.00261279421991182,-0.025945861727546,
-0.0105573018927509));
#15089=CARTESIAN_POINT('Ctrl Pts',(0.00248773509955849,-0.0259581632380008,
-0.0103554215273472));
#15090=CARTESIAN_POINT('Ctrl Pts',(0.00233928586059097,-0.0259704647484557,
-0.0101683027370409));
#15091=CARTESIAN_POINT('Ctrl Pts',(0.00217165560515604,-0.0259827662589106,
-0.010000924740009));
#15092=CARTESIAN_POINT('Ctrl Pts',(0.00177888037096302,-0.0260115899854944,
-0.00960874057365779));
#15093=CARTESIAN_POINT('Ctrl Pts',(0.00127524104593229,-0.0260404137120782,
-0.00932446792274665));
#15094=CARTESIAN_POINT('Ctrl Pts',(0.000734386477435069,-0.0260692374386621,
-0.00919138034284417));
#15095=CARTESIAN_POINT('Ctrl Pts',(0.000493407443421635,-0.0260820799183108,
-0.00913208285639934));
#15096=CARTESIAN_POINT('Ctrl Pts',(0.000245427868459588,-0.0260949223979595,
-0.00910219430558744));
#15097=CARTESIAN_POINT('Ctrl Pts',(-1.98291230682416E-6,-0.0261077648776082,
-0.00910235392621023));
#15098=CARTESIAN_POINT('Ctrl Pts',(-0.000559326620774171,-0.0261366952063965,
-0.00910271350451791));
#15099=CARTESIAN_POINT('Ctrl Pts',(-0.00111841896355447,-0.0261656255351847,
-0.00925900913306373));
#15100=CARTESIAN_POINT('Ctrl Pts',(-0.00159609997232856,-0.026194555863973,
-0.00954928382653372));
#15101=CARTESIAN_POINT('Ctrl Pts',(-0.00180638748166665,-0.0262072917414173,
-0.00967707023878891));
#15102=CARTESIAN_POINT('Ctrl Pts',(-0.00200105397037653,-0.0262200276188616,
-0.00983013604509866));
#15103=CARTESIAN_POINT('Ctrl Pts',(-0.00217446016899265,-0.0262327634963059,
-0.0100037286990944));
#15104=CARTESIAN_POINT('Ctrl Pts',(-0.00256828896208452,-0.026261688386436,
-0.0103979809574239));
#15105=CARTESIAN_POINT('Ctrl Pts',(-0.00285313149746629,-0.0262906132765661,
-0.0109037072449803));
#15106=CARTESIAN_POINT('Ctrl Pts',(-0.00298573082506832,-0.0263195381666962,
-0.011446597713911));
#15107=CARTESIAN_POINT('Ctrl Pts',(-0.00304414037961968,-0.0263322794827987,
-0.0116857391261178));
#15108=CARTESIAN_POINT('Ctrl Pts',(-0.00307360514234931,-0.0263450207989011,
-0.0119317172695922));
#15109=CARTESIAN_POINT('Ctrl Pts',(-0.00307349971650223,-0.0263577621150035,
-0.0121771733853063));
#15110=CARTESIAN_POINT('Ctrl Pts',(-0.00307326038243195,-0.0263866870051336,
-0.0127343992732539));
#15111=CARTESIAN_POINT('Ctrl Pts',(-0.00291714915791347,-0.0264156118952638,
-0.0132934262821599));
#15112=CARTESIAN_POINT('Ctrl Pts',(-0.00262707914936251,-0.0264445367853939,
-0.0137711142034569));
#15113=CARTESIAN_POINT('Ctrl Pts',(-0.00249930429337674,-0.0264572781014963,
-0.0139815341143424));
#15114=CARTESIAN_POINT('Ctrl Pts',(-0.00234622283697911,-0.0264700194175988,
-0.0141763272798705));
#15115=CARTESIAN_POINT('Ctrl Pts',(-0.00217259346875283,-0.0264827607337012,
-0.0143498449768671));
#15116=CARTESIAN_POINT('Ctrl Pts',(-0.00177835203641551,-0.0265116910624894,
-0.0147438328494178));
#15117=CARTESIAN_POINT('Ctrl Pts',(-0.00127257886971661,-0.0265406213912777,
-0.0150288124134629));
#15118=CARTESIAN_POINT('Ctrl Pts',(-0.000729601329433494,-0.0265695517200659,
-0.0151614996403798));
#15119=CARTESIAN_POINT('Ctrl Pts',(-0.000490568601576626,-0.0265822875975102,
-0.0152199119824173));
#15120=CARTESIAN_POINT('Ctrl Pts',(-0.000244699846216731,-0.0265950234749545,
-0.0152494056872691));
#15121=CARTESIAN_POINT('Ctrl Pts',(6.57285128261936E-7,-0.0266077593523988,
-0.0152493532162761));
#15122=CARTESIAN_POINT('Ctrl Pts',(0.000555947401589652,-0.0266365830789827,
-0.0152492344643828));
#15123=CARTESIAN_POINT('Ctrl Pts',(0.00111321833243329,-0.0266654068055665,
-0.0150942913426623));
#15124=CARTESIAN_POINT('Ctrl Pts',(0.00158982325464466,-0.0266942305321503,
-0.0148062266952191));
#15125=CARTESIAN_POINT('Ctrl Pts',(0.0018021757065795,-0.0267070730117991,
-0.0146778788092668));
#15126=CARTESIAN_POINT('Ctrl Pts',(0.00199867134309933,-0.0267199154914478,
-0.0145238043854205));
#15127=CARTESIAN_POINT('Ctrl Pts',(0.00217352311052001,-0.0267327579710965,
-0.0143489155355596));
#15128=CARTESIAN_POINT('Ctrl Pts',(0.00257332666068658,-0.0267621226668742,
-0.0139490271953364));
#15129=CARTESIAN_POINT('Ctrl Pts',(0.00286069689813898,-0.0267914873626519,
-0.0134347726021502));
#15130=CARTESIAN_POINT('Ctrl Pts',(0.00299116973179934,-0.0268208520584295,
-0.012882469084264));
#15131=CARTESIAN_POINT('Ctrl Pts',(0.00304582764276496,-0.0268331535688844,
-0.0126510971146384));
#15132=CARTESIAN_POINT('Ctrl Pts',(0.00307349957273473,-0.0268454550793392,
-0.0124133878459035));
#15133=CARTESIAN_POINT('Ctrl Pts',(0.00307349999999503,-0.0268577565897941,
-0.0121758588150803));
#15134=CARTESIAN_POINT('',(-0.0013261977441873,-0.0271787743898721,-0.00940320080322876));
#15135=CARTESIAN_POINT('Ctrl Pts',(0.00307490613955397,-0.0268602076302924,
-0.012175775310944));
#15136=CARTESIAN_POINT('Ctrl Pts',(0.00307491292342961,-0.0268611376005165,
-0.012158051380771));
#15137=CARTESIAN_POINT('Ctrl Pts',(0.00307476249686456,-0.0268620613829282,
-0.0121403314445906));
#15138=CARTESIAN_POINT('Ctrl Pts',(0.00307445305337281,-0.0268629793711641,
-0.0121226174982785));
#15139=CARTESIAN_POINT('Ctrl Pts',(0.00306573943659914,-0.0268888289944517,
-0.0116238106277867));
#15140=CARTESIAN_POINT('Ctrl Pts',(0.00293065178342736,-0.0269100842487583,
-0.0111276312005785));
#15141=CARTESIAN_POINT('Ctrl Pts',(0.00268958940748811,-0.0269355342842967,
-0.0106913744809503));
#15142=CARTESIAN_POINT('Ctrl Pts',(0.00243996627138719,-0.0269618881176572,
-0.0102396251356849));
#15143=CARTESIAN_POINT('Ctrl Pts',(0.00207616383323794,-0.0269930635228418,
-0.0098502833634627));
#15144=CARTESIAN_POINT('Ctrl Pts',(0.00163926437820477,-0.0270202698942173,
-0.00957464222116215));
#15145=CARTESIAN_POINT('Ctrl Pts',(0.00163155978799815,-0.0270207496703764,
-0.00956978137269679));
#15146=CARTESIAN_POINT('Ctrl Pts',(0.00162383366347141,-0.0270212278936503,
-0.00956495627789788));
#15147=CARTESIAN_POINT('Ctrl Pts',(0.00161608611459192,-0.0270217046142949,
-0.0095601673085752));
#15148=CARTESIAN_POINT('Ctrl Pts',(0.00118449817741507,-0.0270482609978461,
-0.00929339114190244));
#15149=CARTESIAN_POINT('Ctrl Pts',(0.000684240449115547,-0.0270701544205097,
-0.00913816439777956));
#15150=CARTESIAN_POINT('Ctrl Pts',(0.000178117810484161,-0.0270960725546501,
-0.00910966736202029));
#15151=CARTESIAN_POINT('Ctrl Pts',(-0.000337090369108963,-0.0271224559520518,
-0.00908065876845681));
#15152=CARTESIAN_POINT('Ctrl Pts',(-0.000860189467237764,-0.027152024494513,
-0.00918030222031895));
#15153=CARTESIAN_POINT('Ctrl Pts',(-0.00132619774419796,-0.0271787743898752,
-0.00940320080323842));
#15154=CARTESIAN_POINT('',(-0.00290082504980717,-0.0271763869731017,-0.0131997112254818));
#15155=CARTESIAN_POINT('Origin',(0.,-0.0271787743898824,-0.0121758532865681));
#15156=CARTESIAN_POINT('',(0.0030735,-0.0266247798641645,-0.0121758532205251));
#15157=CARTESIAN_POINT('Ctrl Pts',(-0.00289961087048566,-0.0271763232091976,
-0.0131992324493061));
#15158=CARTESIAN_POINT('Ctrl Pts',(-0.00308763169612782,-0.0271471980364023,
-0.0126662862034661));
#15159=CARTESIAN_POINT('Ctrl Pts',(-0.00312155308971536,-0.0271224964632597,
-0.0120796370457119));
#15160=CARTESIAN_POINT('Ctrl Pts',(-0.00300304924290092,-0.0270927645607504,
-0.011527470947428));
#15161=CARTESIAN_POINT('Ctrl Pts',(-0.00293451349166028,-0.0270755693529233,
-0.0112081301043012));
#15162=CARTESIAN_POINT('Ctrl Pts',(-0.00281529683471947,-0.0270568702133368,
-0.0109001188883222));
#15163=CARTESIAN_POINT('Ctrl Pts',(-0.00265107719335906,-0.0270388739894333,
-0.0106192115375074));
#15164=CARTESIAN_POINT('Ctrl Pts',(-0.00259301567986319,-0.0270325112426364,
-0.0105198939053088));
#15165=CARTESIAN_POINT('Ctrl Pts',(-0.0025295230107784,-0.0270264147659866,
-0.0104236706696188));
#15166=CARTESIAN_POINT('Ctrl Pts',(-0.00246051730748276,-0.0270204974975181,
-0.0103314076212616));
#15167=CARTESIAN_POINT('Ctrl Pts',(-0.00219969424658502,-0.0269981318088809,
-0.0099826780303586));
#15168=CARTESIAN_POINT('Ctrl Pts',(-0.00185877014511459,-0.0269783263552642,
-0.00969034090217038));
#15169=CARTESIAN_POINT('Ctrl Pts',(-0.00147503608472361,-0.02695637990696,
-0.00948099890407491));
#15170=CARTESIAN_POINT('Ctrl Pts',(-0.00117664367801609,-0.0269393143029282,
-0.00931821412918935));
#15171=CARTESIAN_POINT('Ctrl Pts',(-0.000851985381520887,-0.0269210215646513,
-0.00920449927642397));
#15172=CARTESIAN_POINT('Ctrl Pts',(-0.000518818664669812,-0.0269020068478604,
-0.00914659649850862));
#15173=CARTESIAN_POINT('Ctrl Pts',(-0.000275393555156683,-0.026888113924939,
-0.00910429038165403));
#15174=CARTESIAN_POINT('Ctrl Pts',(-2.59212939084465E-5,-0.0268748219903249,
-0.00908976765259022));
#15175=CARTESIAN_POINT('Ctrl Pts',(0.000221735837015603,-0.0268620018707547,
-0.00910749573534982));
#15176=CARTESIAN_POINT('Ctrl Pts',(0.000525307879835055,-0.0268462872823129,
-0.00912922638481073));
#15177=CARTESIAN_POINT('Ctrl Pts',(0.000826058247928513,-0.0268312816080388,
-0.00919954037695764));
#15178=CARTESIAN_POINT('Ctrl Pts',(0.00110976365222905,-0.0268167469419083,
-0.00931015671458052));
#15179=CARTESIAN_POINT('Ctrl Pts',(0.0014265401172301,-0.0268005179942499,
-0.00943366741219987));
#15180=CARTESIAN_POINT('Ctrl Pts',(0.00172191944737471,-0.0267832082732035,
-0.00960988343338538));
#15181=CARTESIAN_POINT('Ctrl Pts',(0.00198065347741659,-0.0267648525352007,
-0.00982725230390036));
#15182=CARTESIAN_POINT('Ctrl Pts',(0.00227095652361926,-0.0267442571513749,
-0.0100711430872269));
#15183=CARTESIAN_POINT('Ctrl Pts',(0.0025193142480031,-0.0267226761994269,
-0.0103697063505273));
#15184=CARTESIAN_POINT('Ctrl Pts',(0.00270111735108537,-0.0267025569396926,
-0.0107044215657649));
#15185=CARTESIAN_POINT('Ctrl Pts',(0.0027889247782419,-0.0266928397214294,
-0.01086608262315));
#15186=CARTESIAN_POINT('Ctrl Pts',(0.00286131189634785,-0.0266834634729189,
-0.0110361616317958));
#15187=CARTESIAN_POINT('Ctrl Pts',(0.0029187151677258,-0.0266747039152927,
-0.0112112645346353));
#15188=CARTESIAN_POINT('Ctrl Pts',(0.00302065102293573,-0.0266591488262456,
-0.0115222096031344));
#15189=CARTESIAN_POINT('Ctrl Pts',(0.00307230929529488,-0.0266437720605787,
-0.0118493837213127));
#15190=CARTESIAN_POINT('Ctrl Pts',(0.00307224986630574,-0.0266269429077654,
-0.0121759396378161));
#15191=CARTESIAN_POINT('',(0.00307349935664723,-0.0256248537561334,-0.0121772619237424));
#15192=CARTESIAN_POINT('Ctrl Pts',(0.0030735,-0.0266247798641645,-0.0121758532205251));
#15193=CARTESIAN_POINT('Ctrl Pts',(0.00307350001218174,-0.0265954233398465,
-0.0127428512174199));
#15194=CARTESIAN_POINT('Ctrl Pts',(0.00291229937933948,-0.0265660668155286,
-0.0133099880167539));
#15195=CARTESIAN_POINT('Ctrl Pts',(0.00261419079830434,-0.0265367102912106,
-0.0137921480369242));
#15196=CARTESIAN_POINT('Ctrl Pts',(0.00248924640825892,-0.0265244062742915,
-0.0139942327585893));
#15197=CARTESIAN_POINT('Ctrl Pts',(0.00234087672716486,-0.0265121022573725,
-0.0141815619079462));
#15198=CARTESIAN_POINT('Ctrl Pts',(0.00217329292152179,-0.0264997982404535,
-0.01434914574899));
#15199=CARTESIAN_POINT('Ctrl Pts',(0.00178081767495824,-0.0264709826752771,
-0.0147416210784607));
#15200=CARTESIAN_POINT('Ctrl Pts',(0.00127739859003859,-0.0264421671101007,
-0.0150262717538645));
#15201=CARTESIAN_POINT('Ctrl Pts',(0.000736650025021551,-0.0264133515449242,
-0.0151597683306965));
#15202=CARTESIAN_POINT('Ctrl Pts',(0.000495602930727057,-0.0264005065579828,
-0.0152192765088507));
#15203=CARTESIAN_POINT('Ctrl Pts',(0.000247526363821311,-0.0263876615710414,
-0.0152493532903629));
#15204=CARTESIAN_POINT('Ctrl Pts',(-4.72438689886815E-11,-0.0263748165841,
-0.0152493532865581));
#15205=CARTESIAN_POINT('Ctrl Pts',(-0.000557337869483213,-0.0263458944298224,
-0.0152493532779911));
#15206=CARTESIAN_POINT('Ctrl Pts',(-0.00111652614259104,-0.0263169722755447,
-0.0150934215947984));
#15207=CARTESIAN_POINT('Ctrl Pts',(-0.00159439172129221,-0.0262880501212671,
-0.0148034600472959));
#15208=CARTESIAN_POINT('Ctrl Pts',(-0.00180486158453935,-0.0262753117234269,
-0.0146757501431516));
#15209=CARTESIAN_POINT('Ctrl Pts',(-0.00199971203677584,-0.0262625733255867,
-0.0145227266810762));
#15210=CARTESIAN_POINT('Ctrl Pts',(-0.00217329298833469,-0.0262498349277465,
-0.0143491456821771));
#15211=CARTESIAN_POINT('Ctrl Pts',(-0.00256732938986629,-0.0262209182038713,
-0.0139551091731811));
#15212=CARTESIAN_POINT('Ctrl Pts',(-0.0028524424777176,-0.0261920014799961,
-0.0134495414786068));
#15213=CARTESIAN_POINT('Ctrl Pts',(-0.00298533501378733,-0.0261630847561209,
-0.0129067274928723));
#15214=CARTESIAN_POINT('Ctrl Pts',(-0.00304390180239396,-0.0261503409278783,
-0.0126675050888499));
#15215=CARTESIAN_POINT('Ctrl Pts',(-0.00307350006319907,-0.0261375970996357,
-0.0124214237788402));
#15216=CARTESIAN_POINT('Ctrl Pts',(-0.0030734999999999,-0.0261248532713931,
-0.0121758524955754));
#15217=CARTESIAN_POINT('Ctrl Pts',(-0.00307349985659614,-0.0260959365475179,
-0.0116186324158105));
#15218=CARTESIAN_POINT('Ctrl Pts',(-0.00291763174738019,-0.0260670198236426,
-0.0110595431121297));
#15219=CARTESIAN_POINT('Ctrl Pts',(-0.00262777159708766,-0.0260381030997674,
-0.0105817332523262));
#15220=CARTESIAN_POINT('Ctrl Pts',(-0.00250002794308169,-0.0260253592715248,
-0.0103711586792096));
#15221=CARTESIAN_POINT('Ctrl Pts',(-0.0023469469085358,-0.0260126154432822,
-0.0101762146797365));
#15222=CARTESIAN_POINT('Ctrl Pts',(-0.00217329186971606,-0.0259998716150396,
-0.0100025597723208));
#15223=CARTESIAN_POINT('Ctrl Pts',(-0.00177918126745261,-0.025970949460762,
-0.00960844946827901));
#15224=CARTESIAN_POINT('Ctrl Pts',(-0.00127350533089006,-0.0259420273064843,
-0.00932330853013815));
#15225=CARTESIAN_POINT('Ctrl Pts',(-0.000730575770667611,-0.0259131051522067,
-0.00919044522511768));
#15226=CARTESIAN_POINT('Ctrl Pts',(-0.000491449297897936,-0.0259003667543665,
-0.00913192725921977));
#15227=CARTESIAN_POINT('Ctrl Pts',(-0.000245470875214288,-0.0258876283565263,
-0.00910235316398429));
#15228=CARTESIAN_POINT('Ctrl Pts',(1.53472154182256E-9,-0.0258748899586861,
-0.00910235328655848));
#15229=CARTESIAN_POINT('Ctrl Pts',(0.000555285355831455,-0.0258460743935097,
-0.00910235356383391));
#15230=CARTESIAN_POINT('Ctrl Pts',(0.00111258429007166,-0.0258172588283333,
-0.00925717441826294));
#15231=CARTESIAN_POINT('Ctrl Pts',(0.00158924789974853,-0.0257884432631569,
-0.00954513221370661));
#15232=CARTESIAN_POINT('Ctrl Pts',(0.00180172812716241,-0.0257755982762155,
-0.0096734938855845));
#15233=CARTESIAN_POINT('Ctrl Pts',(0.00199834217675505,-0.0257627532892741,
-0.00982760986230361));
#15234=CARTESIAN_POINT('Ctrl Pts',(0.00217329404013981,-0.0257499083023327,
-0.010002561942745));
#15235=CARTESIAN_POINT('Ctrl Pts',(0.00257313709327206,-0.0257205517770763,
-0.0104024054919486));
#15236=CARTESIAN_POINT('Ctrl Pts',(0.00286056100861589,-0.02569119525182,
-0.0109166263961833));
#15237=CARTESIAN_POINT('Ctrl Pts',(0.00299109311605828,-0.0256618387265637,
-0.011468913245912));
#15238=CARTESIAN_POINT('Ctrl Pts',(0.00304580226648514,-0.0256495346997022,
-0.0117003899678665));
#15239=CARTESIAN_POINT('Ctrl Pts',(0.00307350017616934,-0.0256372306728407,
-0.0119382130388463));
#15240=CARTESIAN_POINT('Ctrl Pts',(0.00307349999999916,-0.0256249266459792,
-0.0121758555650184));
#15241=CARTESIAN_POINT('',(0.00307349987269237,-0.024624748008777,-0.0121752386980468));
#15242=CARTESIAN_POINT('Ctrl Pts',(0.00307349871570724,-0.0256247811395518,
-0.0121786630100232));
#15243=CARTESIAN_POINT('Ctrl Pts',(0.00307298037501563,-0.0255954138959754,
-0.0127456652327553));
#15244=CARTESIAN_POINT('Ctrl Pts',(0.00291125891857178,-0.0255660466523991,
-0.0133126581730836));
#15245=CARTESIAN_POINT('Ctrl Pts',(0.00261270561721589,-0.0255366794088227,
-0.0137945477011307));
#15246=CARTESIAN_POINT('Ctrl Pts',(0.00248766720975212,-0.0255243799857324,
-0.0139963699515859));
#15247=CARTESIAN_POINT('Ctrl Pts',(0.00233925141307591,-0.0255120805626421,
-0.0141834369067124));
#15248=CARTESIAN_POINT('Ctrl Pts',(0.00217166421594283,-0.0254997811395518,
-0.0143507732352444));
#15249=CARTESIAN_POINT('Ctrl Pts',(0.00177888813102166,-0.025470954837001,
-0.0147429613564746));
#15250=CARTESIAN_POINT('Ctrl Pts',(0.00127524673881237,-0.0254421285344501,
-0.0150272366276994));
#15251=CARTESIAN_POINT('Ctrl Pts',(0.000734389712799084,-0.0254133022318993,
-0.0151603254341472));
#15252=CARTESIAN_POINT('Ctrl Pts',(0.000493470811168384,-0.0254004618677835,
-0.0152196084008585));
#15253=CARTESIAN_POINT('Ctrl Pts',(0.000245554842806924,-0.0253876215036676,
-0.015249497186873));
#15254=CARTESIAN_POINT('Ctrl Pts',(-1.79457787336804E-6,-0.0253747811395518,
-0.0152493527626424));
#15255=CARTESIAN_POINT('Ctrl Pts',(-0.000559141493980125,-0.0253458482343444,
-0.0152490273347543));
#15256=CARTESIAN_POINT('Ctrl Pts',(-0.00111824595371007,-0.025316915329137,
-0.0150927642575334));
#15257=CARTESIAN_POINT('Ctrl Pts',(-0.00159594612820109,-0.0252879824239296,
-0.0148025162276071));
#15258=CARTESIAN_POINT('Ctrl Pts',(-0.00180618841211308,-0.0252752486624703,
-0.0146747741584783));
#15259=CARTESIAN_POINT('Ctrl Pts',(-0.00200081903578972,-0.0252625149010111,
-0.0145217645205726));
#15260=CARTESIAN_POINT('Ctrl Pts',(-0.00217420255139949,-0.0252497811395518,
-0.0143482357380357));
#15261=CARTESIAN_POINT('Ctrl Pts',(-0.00256808028828137,-0.0252208536770538,
-0.013954027996261));
#15262=CARTESIAN_POINT('Ctrl Pts',(-0.00285298337185679,-0.0251919262145559,
-0.013448332571431));
#15263=CARTESIAN_POINT('Ctrl Pts',(-0.00298564623897108,-0.0251629987520579,
-0.0129054550859788));
#15264=CARTESIAN_POINT('Ctrl Pts',(-0.00304406890047807,-0.0251502595478892,
-0.0126663802923892));
#15265=CARTESIAN_POINT('Ctrl Pts',(-0.00307356213274085,-0.0251375203437205,
-0.0124204688459204));
#15266=CARTESIAN_POINT('Ctrl Pts',(-0.00307349990116896,-0.0251247811395518,
-0.0121750738544722));
#15267=CARTESIAN_POINT('Ctrl Pts',(-0.00307335858924413,-0.0250958536770538,
-0.0116178448220857));
#15268=CARTESIAN_POINT('Ctrl Pts',(-0.0029173440407025,-0.0250669262145559,
-0.0110587878836229));
#15269=CARTESIAN_POINT('Ctrl Pts',(-0.00262735552814881,-0.0250379987520579,
-0.0105810475997405));
#15270=CARTESIAN_POINT('Ctrl Pts',(-0.00249964910148719,-0.0250252595478892,
-0.0103706582157277));
#15271=CARTESIAN_POINT('Ctrl Pts',(-0.00234664610208603,-0.0250125203437205,
-0.0101758833232711));
#15272=CARTESIAN_POINT('Ctrl Pts',(-0.00217310045002427,-0.0249997811395518,
-0.0100023683696322));
#15273=CARTESIAN_POINT('Ctrl Pts',(-0.00177894867776568,-0.0249708482343444,
-0.00960828631872732));
#15274=CARTESIAN_POINT('Ctrl Pts',(-0.00127323899679475,-0.024941915329137,
-0.00932318820737745));
#15275=CARTESIAN_POINT('Ctrl Pts',(-0.000730289593933061,-0.0249129824239296,
-0.00919037520775847));
#15276=CARTESIAN_POINT('Ctrl Pts',(-0.000491330245367016,-0.0249002486624703,
-0.00913192241694081));
#15277=CARTESIAN_POINT('Ctrl Pts',(-0.000245531643034035,-0.0248875149010111,
-0.00910237210790608));
#15278=CARTESIAN_POINT('Ctrl Pts',(-2.35713786740483E-7,-0.0248747811395518,
-0.00910235329559681));
#15279=CARTESIAN_POINT('Ctrl Pts',(0.000555057762818296,-0.024845954837001,
-0.00910231070886231));
#15280=CARTESIAN_POINT('Ctrl Pts',(0.00111237636565889,-0.0248171285344501,
-0.00925709369733194));
#15281=CARTESIAN_POINT('Ctrl Pts',(0.00158906643107183,-0.0247883022318993,
-0.00954502259500065));
#15282=CARTESIAN_POINT('Ctrl Pts',(0.00180140285540206,-0.0247754618677835,
-0.00967327740253341));
#15283=CARTESIAN_POINT('Ctrl Pts',(0.00199789782178222,-0.0247626215036676,
-0.00982725041082163));
#15284=CARTESIAN_POINT('Ctrl Pts',(0.00217276704534377,-0.0247497811395518,
-0.0100020350750537));
#15285=CARTESIAN_POINT('Ctrl Pts',(0.00257271108400271,-0.0247204138959755,
-0.010401785717762));
#15286=CARTESIAN_POINT('Ctrl Pts',(0.00286026047587044,-0.0246910466523991,
-0.0109159421159849));
#15287=CARTESIAN_POINT('Ctrl Pts',(0.00299092486810477,-0.0246616794088228,
-0.0114682017597792));
#15288=CARTESIAN_POINT('Ctrl Pts',(0.00304564899087614,-0.0246493799857324,
-0.0116994960246657));
#15289=CARTESIAN_POINT('Ctrl Pts',(0.0030734030999119,-0.0246370805626421,
-0.0119371336788303));
#15290=CARTESIAN_POINT('Ctrl Pts',(0.00307349974546122,-0.0246247811395518,
-0.0121746024269245));
#15291=CARTESIAN_POINT('Ctrl Pts',(0.00307349999992352,-0.0246247148780022,
-0.0121758749691691));
#15292=CARTESIAN_POINT('Ctrl Pts',(0.00307349599990712,-0.024595352466092,
-0.0127428754284441));
#15293=CARTESIAN_POINT('Ctrl Pts',(0.00291229002300707,-0.0245659900541818,
-0.0133100131564192));
#15294=CARTESIAN_POINT('Ctrl Pts',(0.00261417579362664,-0.0245366276422716,
-0.0137921723051978));
#15295=CARTESIAN_POINT('Ctrl Pts',(0.00248927970630659,-0.024524326148413,
-0.0139941747096894));
#15296=CARTESIAN_POINT('Ctrl Pts',(0.0023409773439075,-0.0245120246545545,
-0.0141814332731449));
#15297=CARTESIAN_POINT('Ctrl Pts',(0.00217347456253716,-0.0244997231606959,
-0.0143489640927537));
#15298=CARTESIAN_POINT('Ctrl Pts',(0.00178102831398537,-0.0244709016982887,
-0.0147414760327609));
#15299=CARTESIAN_POINT('Ctrl Pts',(0.00127762796176171,-0.0244420802358815,
-0.0150261697812338));
#15300=CARTESIAN_POINT('Ctrl Pts',(0.000736885823996938,-0.0244132587734743,
-0.0151597101082559));
#15301=CARTESIAN_POINT('Ctrl Pts',(0.000495938637509918,-0.0244004163301127,
-0.0152192138233012));
#15302=CARTESIAN_POINT('Ctrl Pts',(0.000247965232569662,-0.0243875738867512,
-0.0152493100806458));
#15303=CARTESIAN_POINT('Ctrl Pts',(5.36111760505852E-7,-0.0243747314433896,
-0.015249353239801));
#15304=CARTESIAN_POINT('Ctrl Pts',(-0.000556806754329106,-0.0243458033844476,
-0.0152494504573282));
#15305=CARTESIAN_POINT('Ctrl Pts',(-0.00111602625065947,-0.0243168753255056,
-0.015093613618999));
#15306=CARTESIAN_POINT('Ctrl Pts',(-0.00159394459477676,-0.0242879472665637,
-0.0148037313048044));
#15307=CARTESIAN_POINT('Ctrl Pts',(-0.00180435258788129,-0.0242752114197369,
-0.0146761079216115));
#15308=CARTESIAN_POINT('Ctrl Pts',(-0.0019991579586532,-0.0242624755729101,
-0.0145231885374881));
#15309=CARTESIAN_POINT('Ctrl Pts',(-0.00217271631721875,-0.0242497397260833,
-0.0143497222004743));
#15310=CARTESIAN_POINT('Ctrl Pts',(-0.0025668607214936,-0.0242208171043095,
-0.0139557867736294));
#15311=CARTESIAN_POINT('Ctrl Pts',(-0.0028521088439021,-0.0241918944825356,
-0.0134502901086501));
#15312=CARTESIAN_POINT('Ctrl Pts',(-0.00298514405465798,-0.0241629718607618,
-0.012907507045477));
#15313=CARTESIAN_POINT('Ctrl Pts',(-0.00304375006260632,-0.0241502305767668,
-0.0126683947959168));
#15314=CARTESIAN_POINT('Ctrl Pts',(-0.00307341243721463,-0.0241374892927719,
-0.0124224215391223));
#15315=CARTESIAN_POINT('Ctrl Pts',(-0.00307349980533095,-0.024124748008777,
-0.0121769471926725));
#15316=CARTESIAN_POINT('Ctrl Pts',(-0.00307369813031801,-0.0240958253870032,
-0.0116197222159447));
#15317=CARTESIAN_POINT('Ctrl Pts',(-0.00291802652412777,-0.0240669027652293,
-0.011060573504202));
#15318=CARTESIAN_POINT('Ctrl Pts',(-0.00262833255001533,-0.0240379801434555,
-0.010582658302719));
#15319=CARTESIAN_POINT('Ctrl Pts',(-0.00250071364932767,-0.0240252388594605,
-0.0103721222954651));
#15320=CARTESIAN_POINT('Ctrl Pts',(-0.002347772072134,-0.0240124975754656,
-0.010177195475843));
#15321=CARTESIAN_POINT('Ctrl Pts',(-0.00217426319369506,-0.0239997562914707,
-0.0100035315298786));
#15322=CARTESIAN_POINT('Ctrl Pts',(-0.00178032526213027,-0.0239708282325287,
-0.00960924152998886));
#15323=CARTESIAN_POINT('Ctrl Pts',(-0.00127477209842849,-0.0239419001735867,
-0.00932387362135798));
#15324=CARTESIAN_POINT('Ctrl Pts',(-0.000731897509323036,-0.0239129721146448,
-0.00919076898526161));
#15325=CARTESIAN_POINT('Ctrl Pts',(-0.000492891925613767,-0.023900236267818,
-0.00913216843205273));
#15326=CARTESIAN_POINT('Ctrl Pts',(-0.000247027045862867,-0.0238875004209912,
-0.00910248559522246));
#15327=CARTESIAN_POINT('Ctrl Pts',(-1.65170043229059E-6,-0.0238747645741644,
-0.00910235373037045));
#15328=CARTESIAN_POINT('Ctrl Pts',(0.000553637350242043,-0.0238459431117572,
-0.00910205531771469));
#15329=CARTESIAN_POINT('Ctrl Pts',(0.00111102372754518,-0.02381712164935,
-0.00925657921020503));
#15330=CARTESIAN_POINT('Ctrl Pts',(0.00158784448799195,-0.0237883001869428,
-0.00954428490782393));
#15331=CARTESIAN_POINT('Ctrl Pts',(0.00180030919651852,-0.0237754577435812,
-0.00967248257088029));
#15332=CARTESIAN_POINT('Ctrl Pts',(0.00199693407333457,-0.0237626153002197,
-0.00982642253680694));
#15333=CARTESIAN_POINT('Ctrl Pts',(0.00217192712459075,-0.0237497728568581,
-0.0100011958846975));
#15334=CARTESIAN_POINT('Ctrl Pts',(0.00257202373453882,-0.0237204104449479,
-0.0104007901742898));
#15335=CARTESIAN_POINT('Ctrl Pts',(0.00285977136180032,-0.0236910480330377,
-0.0109148331126464));
#15336=CARTESIAN_POINT('Ctrl Pts',(0.00299064981277481,-0.0236616856211274,
-0.0114670402312678));
#15337=CARTESIAN_POINT('Ctrl Pts',(0.00304548183630884,-0.0236493841272689,
-0.0116983894984578));
#15338=CARTESIAN_POINT('Ctrl Pts',(0.00307332843671528,-0.0236370826334104,
-0.0119360968598615));
#15339=CARTESIAN_POINT('Ctrl Pts',(0.00307349920581301,-0.0236247811395518,
-0.0121736437918623));
#15340=CARTESIAN_POINT('Origin',(0.,-0.0271787743898721,-0.0121758532865581));
#15341=CARTESIAN_POINT('',(0.00251751029526666,-0.0221787894580564,-0.01217507662023));
#15342=CARTESIAN_POINT('',(0.00251749942082674,-0.0211788370573946,-0.0121771378810096));
#15343=CARTESIAN_POINT('Ctrl Pts',(0.0025174999999979,-0.0221787227179838,
-0.0121758500317772));
#15344=CARTESIAN_POINT('Ctrl Pts',(0.0025175006270217,-0.0221481735656116,
-0.0126608388780163));
#15345=CARTESIAN_POINT('Ctrl Pts',(0.00237306104723493,-0.0221176054100055,
-0.0131460858681194));
#15346=CARTESIAN_POINT('Ctrl Pts',(0.00210809405127732,-0.0220870179095754,
-0.0135519876262827));
#15347=CARTESIAN_POINT('Ctrl Pts',(0.00201298331277554,-0.0220760384298695,
-0.013697687341972));
#15348=CARTESIAN_POINT('Ctrl Pts',(0.00190281903971488,-0.0220650564576341,
-0.0138333157348486));
#15349=CARTESIAN_POINT('Ctrl Pts',(0.00178014970375261,-0.0220540719770704,
-0.0139559862260403));
#15350=CARTESIAN_POINT('Ctrl Pts',(0.00144068346397155,-0.0220236743207722,
-0.0142954556627196));
#15351=CARTESIAN_POINT('Ctrl Pts',(0.000999662972082794,-0.0219932574554404,
-0.0145361579274445));
#15352=CARTESIAN_POINT('Ctrl Pts',(0.000528152341818232,-0.0219628223855097,
-0.0146373287290177));
#15353=CARTESIAN_POINT('Ctrl Pts',(0.000354602569433263,-0.0219516200941509,
-0.0146745668493443));
#15354=CARTESIAN_POINT('Ctrl Pts',(0.000177184431567649,-0.0219404153364902,
-0.014693352730372));
#15355=CARTESIAN_POINT('Ctrl Pts',(7.90266785490307E-9,-0.021929208162614,
-0.0146933532865457));
#15356=CARTESIAN_POINT('Ctrl Pts',(-0.000329262373811186,-0.0219083804081497,
-0.0146933543201559));
#15357=CARTESIAN_POINT('Ctrl Pts',(-0.0006588475998666,-0.0218875443086468,
-0.0146278711993561));
#15358=CARTESIAN_POINT('Ctrl Pts',(-0.000963400065171092,-0.0218666966492722,
-0.0145017222778017));
#15359=CARTESIAN_POINT('Ctrl Pts',(-0.00126795253047558,-0.0218458489898976,
-0.0143755733562472));
#15360=CARTESIAN_POINT('Ctrl Pts',(-0.00154720597461104,-0.0218249897706513,
-0.0141889292240289));
#15361=CARTESIAN_POINT('Ctrl Pts',(-0.00178013852765,-0.021804132065188,
-0.013955997402178));
#15362=CARTESIAN_POINT('Ctrl Pts',(-0.00189660480416948,-0.0217937032124563,
-0.0138395314912525));
#15363=CARTESIAN_POINT('Ctrl Pts',(-0.00200161407899827,-0.0217832747381703,
-0.0137116060554127));
#15364=CARTESIAN_POINT('Ctrl Pts',(-0.00209322310255972,-0.0217728298716174,
-0.0135745038122114));
#15365=CARTESIAN_POINT('Ctrl Pts',(-0.00218483212612116,-0.0217623850050645,
-0.0134374015690101));
#15366=CARTESIAN_POINT('Ctrl Pts',(-0.00226298661049305,-0.0217519237462447,
-0.0132910645112378));
#15367=CARTESIAN_POINT('Ctrl Pts',(-0.00232586596705365,-0.0217415144103612,
-0.0131392606527857));
#15368=CARTESIAN_POINT('Ctrl Pts',(-0.00238874532361424,-0.0217311050744777,
-0.0129874567943336));
#15369=CARTESIAN_POINT('Ctrl Pts',(-0.00243663034191228,-0.0217207476615306,
-0.0128303642853091));
#15370=CARTESIAN_POINT('Ctrl Pts',(-0.00246912675070183,-0.0217101856814195,
-0.0126669941410679));
#15371=CARTESIAN_POINT('Ctrl Pts',(-0.0024853749550966,-0.021704904691364,
-0.0125853090689473));
#15372=CARTESIAN_POINT('Ctrl Pts',(-0.00249755937086223,-0.0216995725595175,
-0.0125019905764725));
#15373=CARTESIAN_POINT('Ctrl Pts',(-0.00250537750098589,-0.0216945163415666,
-0.0124226119288662));
#15374=CARTESIAN_POINT('Ctrl Pts',(-0.00250928656604771,-0.0216919882325911,
-0.012382922605063));
#15375=CARTESIAN_POINT('Ctrl Pts',(-0.00251226369782038,-0.0216895291020895,
-0.0123442417324174));
#15376=CARTESIAN_POINT('Ctrl Pts',(-0.00251446754887909,-0.0216866804277945,
-0.0122993814033331));
#15377=CARTESIAN_POINT('Ctrl Pts',(-0.0025166713999378,-0.0216838317534995,
-0.0122545210742488));
#15378=CARTESIAN_POINT('Ctrl Pts',(-0.0025175,-0.0216805935354111,-0.0122034465123688));
#15379=CARTESIAN_POINT('Ctrl Pts',(-0.0025175,-0.0216788436847921,-0.012175853286558));
#15380=CARTESIAN_POINT('Ctrl Pts',(-0.0025175,-0.0216770938341731,-0.0121482600607472));
#15381=CARTESIAN_POINT('Ctrl Pts',(-0.00251732341511713,-0.0216768323510236,
-0.0121441379809924));
#15382=CARTESIAN_POINT('Ctrl Pts',(-0.00251714088833399,-0.0216761473547436,
-0.012133332723566));
#15383=CARTESIAN_POINT('Ctrl Pts',(-0.00251695836155086,-0.0216754623584636,
-0.0121225274661396));
#15384=CARTESIAN_POINT('Ctrl Pts',(-0.00251656012884372,-0.0216743538490531,
-0.0121050456834368));
#15385=CARTESIAN_POINT('Ctrl Pts',(-0.00251597543186803,-0.021673288642944,
-0.0120882526231104));
#15386=CARTESIAN_POINT('Ctrl Pts',(-0.00251480603791666,-0.0216711582307259,
-0.0120546665024575));
#15387=CARTESIAN_POINT('Ctrl Pts',(-0.00251312737169555,-0.0216692010317134,
-0.0120238206193739));
#15388=CARTESIAN_POINT('Ctrl Pts',(-0.00251066671451669,-0.0216670840740922,
-0.0119904917516649));
#15389=CARTESIAN_POINT('Ctrl Pts',(-0.00250574540015897,-0.0216628501588498,
-0.0119238340162468));
#15390=CARTESIAN_POINT('Ctrl Pts',(-0.0024973438866829,-0.0216579772091725,
-0.0118472847469798));
#15391=CARTESIAN_POINT('Ctrl Pts',(-0.00248382492313489,-0.0216527263553775,
-0.01176546322672));
#15392=CARTESIAN_POINT('Ctrl Pts',(-0.00247030595958689,-0.0216474755015825,
-0.0116836417064601));
#15393=CARTESIAN_POINT('Ctrl Pts',(-0.00245181307897284,-0.0216418467436696,
-0.0115965131745003));
#15394=CARTESIAN_POINT('Ctrl Pts',(-0.00242619291886598,-0.0216357705286481,
-0.0115039945436332));
#15395=CARTESIAN_POINT('Ctrl Pts',(-0.00240057275875913,-0.0216296943136265,
-0.0114114759127662));
#15396=CARTESIAN_POINT('Ctrl Pts',(-0.00236778366178648,-0.0216231706414963,
-0.0113135845938267));
#15397=CARTESIAN_POINT('Ctrl Pts',(-0.0023256664652384,-0.0216162165939039,
-0.0112119644223909));
#15398=CARTESIAN_POINT('Ctrl Pts',(-0.00224143207214223,-0.0216023084987191,
-0.0110087240795193));
#15399=CARTESIAN_POINT('Ctrl Pts',(-0.00211996024600938,-0.0215866789016856,
-0.0107905612374037));
#15400=CARTESIAN_POINT('Ctrl Pts',(-0.00194563811812038,-0.0215693144003712,
-0.0105782617983118));
#15401=CARTESIAN_POINT('Ctrl Pts',(-0.00177131599023139,-0.0215519498990567,
-0.0103659623592199));
#15402=CARTESIAN_POINT('Ctrl Pts',(-0.00154366358191858,-0.0215328504934613,
-0.0101600234254014));
#15403=CARTESIAN_POINT('Ctrl Pts',(-0.00125814306546542,-0.0215120197747794,
-0.00999528403133567));
#15404=CARTESIAN_POINT('Ctrl Pts',(-0.000972622549012248,-0.0214911890560976,
-0.00983054463726996));
#15405=CARTESIAN_POINT('Ctrl Pts',(-0.000628743563775202,-0.0214686270243295,
-0.00970799681970146));
#15406=CARTESIAN_POINT('Ctrl Pts',(-0.000246101333787693,-0.0214443327171287,
-0.00967041113326301));
#15407=CARTESIAN_POINT('Ctrl Pts',(0.000136540896199817,-0.0214200384099279,
-0.00963282544682456));
#15408=CARTESIAN_POINT('Ctrl Pts',(0.000557976207619178,-0.0213940118272944,
-0.00968195163694664));
#15409=CARTESIAN_POINT('Ctrl Pts',(0.000963897772287331,-0.0213662532274188,
-0.00985019051337289));
#15410=CARTESIAN_POINT('Ctrl Pts',(0.00136981933695548,-0.0213384946275433,
-0.0100184293897991));
#15411=CARTESIAN_POINT('Ctrl Pts',(0.00175889506188566,-0.0213090040104255,
-0.0103082271150057));
#15412=CARTESIAN_POINT('Ctrl Pts',(0.00204652746439145,-0.02127778130565,
-0.010709725192737));
#15413=CARTESIAN_POINT('Ctrl Pts',(0.00229998122120466,-0.0212502687175191,
-0.0110635142487257));
#15414=CARTESIAN_POINT('Ctrl Pts',(0.00247306168481993,-0.0212214112240566,
-0.0115047157964407));
#15415=CARTESIAN_POINT('Ctrl Pts',(0.00250998397883032,-0.0211912088413219,
-0.0119814653342176));
#15416=CARTESIAN_POINT('Ctrl Pts',(0.00251496274895857,-0.021187136214607,
-0.012045752411198));
#15417=CARTESIAN_POINT('Ctrl Pts',(0.00251750023443854,-0.0211830391336996,
-0.012110615346057));
#15418=CARTESIAN_POINT('Ctrl Pts',(0.00251749999998375,-0.0211789175986389,
-0.0121758623327987));
#15419=CARTESIAN_POINT('',(0.00251749999999825,-0.02017876552198,-0.0121758562566413));
#15420=CARTESIAN_POINT('Ctrl Pts',(0.00251749897019639,-0.0211787743898821,
-0.0121781303592641));
#15421=CARTESIAN_POINT('Ctrl Pts',(0.00251705740623119,-0.0211479067710791,
-0.0126663171548534));
#15422=CARTESIAN_POINT('Ctrl Pts',(0.0023703289589053,-0.0211170391522761,
-0.0131543526657776));
#15423=CARTESIAN_POINT('Ctrl Pts',(0.00210170356769341,-0.0210861715334731,
-0.0135617278709072));
#15424=CARTESIAN_POINT('Ctrl Pts',(0.00200772487514791,-0.0210753724856095,
-0.0137042482372092));
#15425=CARTESIAN_POINT('Ctrl Pts',(0.00189928032167646,-0.0210645734377458,
-0.0138370435243574));
#15426=CARTESIAN_POINT('Ctrl Pts',(0.00177874396527104,-0.0210537743898821,
-0.0139573908685394));
#15427=CARTESIAN_POINT('Ctrl Pts',(0.00144055410491447,-0.0210234754112344,
-0.0142950504157245));
#15428=CARTESIAN_POINT('Ctrl Pts',(0.00100184213234116,-0.0209931764325866,
-0.0145346681905484));
#15429=CARTESIAN_POINT('Ctrl Pts',(0.000533254187855318,-0.0209628774539389,
-0.0146362285061404));
#15430=CARTESIAN_POINT('Ctrl Pts',(0.000357447550137102,-0.02095150976592,
-0.0146743322982246));
#15431=CARTESIAN_POINT('Ctrl Pts',(0.000177703303467145,-0.020940142077901,
-0.0146934719846099));
#15432=CARTESIAN_POINT('Ctrl Pts',(-1.67369790539226E-6,-0.0209287743898821,
-0.0146933527301996));
#15433=CARTESIAN_POINT('Ctrl Pts',(-0.000481546144216977,-0.0208983633549288,
-0.0146930336987455));
#15434=CARTESIAN_POINT('Ctrl Pts',(-0.000962865230832859,-0.0208679523199756,
-0.0145511889640779));
#15435=CARTESIAN_POINT('Ctrl Pts',(-0.00136692716455534,-0.0208375412850222,
-0.0142899290602239));
#15436=CARTESIAN_POINT('Ctrl Pts',(-0.00151647723157411,-0.0208262856533089,
-0.0141932324083747));
#15437=CARTESIAN_POINT('Ctrl Pts',(-0.00165558709770307,-0.0208150300215955,
-0.0140806851966216));
#15438=CARTESIAN_POINT('Ctrl Pts',(-0.00178111121517929,-0.0208037743898821,
-0.0139550241859274));
#15439=CARTESIAN_POINT('Ctrl Pts',(-0.00212019485783324,-0.0207733690727329,
-0.0136155707477957));
#15440=CARTESIAN_POINT('Ctrl Pts',(-0.00236026563099572,-0.0207429637555837,
-0.0131750429536424));
#15441=CARTESIAN_POINT('Ctrl Pts',(-0.00246132456596799,-0.0207125584384344,
-0.0127047083054078));
#15442=CARTESIAN_POINT('Ctrl Pts',(-0.00249875420312637,-0.0207012970889169,
-0.0125305084166867));
#15443=CARTESIAN_POINT('Ctrl Pts',(-0.00251757532001169,-0.0206900357393996,
-0.0123524778336015));
#15444=CARTESIAN_POINT('Ctrl Pts',(-0.0025174997724744,-0.0206787743898821,
-0.0121747829635494));
#15445=CARTESIAN_POINT('Ctrl Pts',(-0.00251729579631439,-0.0206483690727328,
-0.0116950119670646));
#15446=CARTESIAN_POINT('Ctrl Pts',(-0.00237562415070273,-0.0206179637555834,
-0.0112137432307141));
#15447=CARTESIAN_POINT('Ctrl Pts',(-0.00211455196730226,-0.0205875584384341,
-0.0108096628797779));
#15448=CARTESIAN_POINT('Ctrl Pts',(-0.00201785752757362,-0.0205762970889167,
-0.0106600018832282));
#15449=CARTESIAN_POINT('Ctrl Pts',(-0.00190529247357263,-0.0205650357393995,
-0.0105207865527399));
#15450=CARTESIAN_POINT('Ctrl Pts',(-0.00177959773126699,-0.0205537743898821,
-0.0103951685404929));
#15451=CARTESIAN_POINT('Ctrl Pts',(-0.00144016175196195,-0.0205233633549287,
-0.0100559397690798));
#15452=CARTESIAN_POINT('Ctrl Pts',(-0.000999596726135764,-0.0204929523199754,
-0.00981574134499383));
#15453=CARTESIAN_POINT('Ctrl Pts',(-0.00052918611128424,-0.020462541285022,
-0.00971459988440222));
#15454=CARTESIAN_POINT('Ctrl Pts',(-0.000355079289766713,-0.0204512856533087,
-0.0096771657413976));
#15455=CARTESIAN_POINT('Ctrl Pts',(-0.000177141891441104,-0.0204400300215954,
-0.00965832038682323));
#15456=CARTESIAN_POINT('Ctrl Pts',(4.66948050388447E-7,-0.0204287743898821,
-0.00965835332986306));
#15457=CARTESIAN_POINT('Ctrl Pts',(0.000478571293721941,-0.0203984754112344,
-0.009658442009067));
#15458=CARTESIAN_POINT('Ctrl Pts',(0.000958339118330285,-0.0203681764325867,
-0.00979905048057223));
#15459=CARTESIAN_POINT('Ctrl Pts',(0.00136155392147097,-0.0203378774539389,
-0.0100583129282822));
#15460=CARTESIAN_POINT('Ctrl Pts',(0.00151283361112674,-0.02032650976592,
-0.0101555840163561));
#15461=CARTESIAN_POINT('Ctrl Pts',(0.00165348256099827,-0.020315142077901,
-0.0102690365665635));
#15462=CARTESIAN_POINT('Ctrl Pts',(0.00178025817466354,-0.0203037743898821,
-0.0103958288256184));
#15463=CARTESIAN_POINT('Ctrl Pts',(0.00212450243168519,-0.0202729067710791,
-0.0107401182812365));
#15464=CARTESIAN_POINT('Ctrl Pts',(0.00236662192217892,-0.0202420391522763,
-0.0111881073528289));
#15465=CARTESIAN_POINT('Ctrl Pts',(0.00246545726791875,-0.0202111715334733,
-0.0116666119782703));
#15466=CARTESIAN_POINT('Ctrl Pts',(0.00250003485020926,-0.0202003724856096,
-0.0118340169985972));
#15467=CARTESIAN_POINT('Ctrl Pts',(0.00251749074081832,-0.0201895734377458,
-0.0120049244588735));
#15468=CARTESIAN_POINT('Ctrl Pts',(0.00251749999630341,-0.0201787743898821,
-0.0121757168596234));
#15469=CARTESIAN_POINT('',(0.00251749967158866,-0.019178682372853,-0.0121750998261193));
#15470=CARTESIAN_POINT('Ctrl Pts',(0.00251749999999825,-0.02017876552198,
-0.0121758562566413));
#15471=CARTESIAN_POINT('Ctrl Pts',(0.00251749942404778,-0.0201478985796235,
-0.0126640430232735));
#15472=CARTESIAN_POINT('Ctrl Pts',(0.00237121201732249,-0.0201170316372671,
-0.0131522106873684));
#15473=CARTESIAN_POINT('Ctrl Pts',(0.00210295494144678,-0.0200861646949107,
-0.0135598282734146));
#15474=CARTESIAN_POINT('Ctrl Pts',(0.00200910037981308,-0.0200753653400964,
-0.013702440615429));
#15475=CARTESIAN_POINT('Ctrl Pts',(0.00190076972724618,-0.0200645659852821,
-0.0138353399771734));
#15476=CARTESIAN_POINT('Ctrl Pts',(0.00178033495272378,-0.0200537666304678,
-0.0139558009560445));
#15477=CARTESIAN_POINT('Ctrl Pts',(0.00144244726229051,-0.0200234683294094,
-0.0142937621645035));
#15478=CARTESIAN_POINT('Ctrl Pts',(0.00100395002775284,-0.019993170028351,
-0.0145337717268215));
#15479=CARTESIAN_POINT('Ctrl Pts',(0.000535453448710425,-0.0199628717272925,
-0.0146357508157784));
#15480=CARTESIAN_POINT('Ctrl Pts',(0.000359672394884014,-0.0199515037311802,
-0.0146740136175298));
#15481=CARTESIAN_POINT('Ctrl Pts',(0.000179936394819805,-0.0199401357350679,
-0.0146933139879726));
#15482=CARTESIAN_POINT('Ctrl Pts',(5.50671286675763E-7,-0.0199287677389556,
-0.0146933532263319));
#15483=CARTESIAN_POINT('Ctrl Pts',(-0.000479321396759237,-0.0198983573824538,
-0.0146934581922805));
#15484=CARTESIAN_POINT('Ctrl Pts',(-0.000960765252524083,-0.0198679470259521,
-0.0145520390541735));
#15485=CARTESIAN_POINT('Ctrl Pts',(-0.00136505768018742,-0.0198375366694503,
-0.0142911366670443));
#15486=CARTESIAN_POINT('Ctrl Pts',(-0.00151470050263993,-0.0198262807287813,
-0.0141945675331126));
#15487=CARTESIAN_POINT('Ctrl Pts',(-0.0016539161141768,-0.0198150247881123,
-0.0140821370557623));
#15488=CARTESIAN_POINT('Ctrl Pts',(-0.00177955610029437,-0.0198037688474433,
-0.0139565796372097));
#15489=CARTESIAN_POINT('Ctrl Pts',(-0.00211893586369603,-0.0197733642079718,
-0.0136174229059933));
#15490=CARTESIAN_POINT('Ctrl Pts',(-0.00235939135465183,-0.0197429595685003,
-0.0131771054644321));
#15491=CARTESIAN_POINT('Ctrl Pts',(-0.00246086132166213,-0.0197125549290287,
-0.0127068596947561));
#15492=CARTESIAN_POINT('Ctrl Pts',(-0.0024984450606929,-0.0197012932713295,
-0.0125326840760133));
#15493=CARTESIAN_POINT('Ctrl Pts',(-0.00251742180734246,-0.0196900316136303,
-0.0123546611207697));
#15494=CARTESIAN_POINT('Ctrl Pts',(-0.00251749975779415,-0.019678769955931,
-0.012176957599188));
#15495=CARTESIAN_POINT('Ctrl Pts',(-0.0025177102113032,-0.0196483653164596,
-0.0116971870671051));
#15496=CARTESIAN_POINT('Ctrl Pts',(-0.00237645460119475,-0.0196179606769882,
-0.011215796495468));
#15497=CARTESIAN_POINT('Ctrl Pts',(-0.00211573195307296,-0.0195875560375168,
-0.0108114909619734));
#15498=CARTESIAN_POINT('Ctrl Pts',(-0.00201916217725421,-0.0195762943798175,
-0.010661739127934));
#15499=CARTESIAN_POINT('Ctrl Pts',(-0.00190671120570611,-0.0195650327221181,
-0.0105224202649405));
#15500=CARTESIAN_POINT('Ctrl Pts',(-0.00178111766245729,-0.0195537710644188,
-0.0103966888415214));
#15501=CARTESIAN_POINT('Ctrl Pts',(-0.00144197181674905,-0.0195233607079171,
-0.0100571706718406));
#15502=CARTESIAN_POINT('Ctrl Pts',(-0.00100161251329237,-0.0194929503514154,
-0.0098165961994737));
#15503=CARTESIAN_POINT('Ctrl Pts',(-0.000531288854696852,-0.0194625399949137,
-0.0097150529283667));
#15504=CARTESIAN_POINT('Ctrl Pts',(-0.000357205555275701,-0.0194512840542446,
-0.00967746819847854));
#15505=CARTESIAN_POINT('Ctrl Pts',(-0.000179275420660757,-0.0194400281135756,
-0.00965847080633757));
#15506=CARTESIAN_POINT('Ctrl Pts',(-1.65795391985757E-6,-0.0194287721729066,
-0.00965835383249881));
#15507=CARTESIAN_POINT('Ctrl Pts',(0.000476445799358355,-0.0193984738718482,
-0.00965803896689255));
#15508=CARTESIAN_POINT('Ctrl Pts',(0.000956331742318686,-0.0193681755707899,
-0.00979824216117706));
#15509=CARTESIAN_POINT('Ctrl Pts',(0.00135976503294221,-0.0193378772697315,
-0.0100571637611232));
#15510=CARTESIAN_POINT('Ctrl Pts',(0.00151113418300043,-0.0193265092736191,
-0.0101543117740077));
#15511=CARTESIAN_POINT('Ctrl Pts',(0.00165188522462424,-0.0193151412775067,
-0.0102676518033066));
#15512=CARTESIAN_POINT('Ctrl Pts',(0.00177877270373225,-0.0193037732813944,
-0.0103943443984363));
#15513=CARTESIAN_POINT('Ctrl Pts',(0.00212330382994413,-0.019272906339038,
-0.0107383463660817));
#15514=CARTESIAN_POINT('Ctrl Pts',(0.00236579690432436,-0.0192420393966816,
-0.0111861330421385));
#15515=CARTESIAN_POINT('Ctrl Pts',(0.0024650314678091,-0.0192111724543252,
-0.0116645548289906));
#15516=CARTESIAN_POINT('Ctrl Pts',(0.00249975046422119,-0.0192003730995108,
-0.0118319392938171));
#15517=CARTESIAN_POINT('Ctrl Pts',(0.00251734898190401,-0.0191895737446965,
-0.0120028408387453));
#15518=CARTESIAN_POINT('Ctrl Pts',(0.00251749902856922,-0.0191787743898821,
-0.0121736416914285));
#15519=CARTESIAN_POINT('',(0.00251749999999651,-0.0181788400336509,-0.0121758574807786));
#15520=CARTESIAN_POINT('Ctrl Pts',(0.0025174999999847,-0.0191786353788967,
-0.0121758445091258));
#15521=CARTESIAN_POINT('Ctrl Pts',(0.00251750170207121,-0.0191478104553933,
-0.0126640285958876));
#15522=CARTESIAN_POINT('Ctrl Pts',(0.0023712181033913,-0.019116981663674,
-0.0131521946266093));
#15523=CARTESIAN_POINT('Ctrl Pts',(0.00200907496145789,-0.0190753508046254,
-0.0137024816231192));
#15524=CARTESIAN_POINT('Ctrl Pts',(0.00190069671332285,-0.0190645563654964,
-0.0138354304943692));
#15525=CARTESIAN_POINT('Ctrl Pts',(0.00144229472143091,-0.0190234846160053,
-0.0142938656603467));
#15526=CARTESIAN_POINT('Ctrl Pts',(0.00100378140055006,-0.0189931985744862,
-0.0145338433849123));
#15527=CARTESIAN_POINT('Ctrl Pts',(0.000359425373225544,-0.0189515497284823,
-0.0146740542590721));
#15528=CARTESIAN_POINT('Ctrl Pts',(0.00017961579626026,-0.0189401837567628,
-0.0146933418902656));
#15529=CARTESIAN_POINT('Ctrl Pts',(-0.000479704801724841,-0.0188984297906503,
-0.0146933837415642));
#15530=CARTESIAN_POINT('Ctrl Pts',(-0.00096112004307815,-0.0188680494431272,
-0.014551894086947));
#15531=CARTESIAN_POINT('Ctrl Pts',(-0.00151506125314685,-0.0188263618747039,
-0.0141943035839131));
#15532=CARTESIAN_POINT('Ctrl Pts',(-0.00165431580166961,-0.018815090775692,
-0.0140817973026295));
#15533=CARTESIAN_POINT('Ctrl Pts',(-0.00211926443661562,-0.018773357645065,
-0.0136169330664543));
#15534=CARTESIAN_POINT('Ctrl Pts',(-0.00235961099893533,-0.0187428433006891,
-0.0131765788736037));
#15535=CARTESIAN_POINT('Ctrl Pts',(-0.00249854058101726,-0.0187011966212453,
-0.0125320589461935));
#15536=CARTESIAN_POINT('Ctrl Pts',(-0.00251747899192606,-0.0186899535052533,
-0.0123539416161887));
#15537=CARTESIAN_POINT('Ctrl Pts',(-0.00251755664288924,-0.0186484623083203,
-0.0116962330356729));
#15538=CARTESIAN_POINT('Ctrl Pts',(-0.00237606299894619,-0.0186183855843164,
-0.0112147502638011));
#15539=CARTESIAN_POINT('Ctrl Pts',(-0.00201845434901466,-0.0185771189445961,
-0.0106608047389055));
#15540=CARTESIAN_POINT('Ctrl Pts',(-0.00190598884271828,-0.0185659656408752,
-0.0105215951671963));
#15541=CARTESIAN_POINT('Ctrl Pts',(-0.00144124441175641,-0.0185246278682585,
-0.0100567188361891));
#15542=CARTESIAN_POINT('Ctrl Pts',(-0.0010009741369636,-0.0184943299457318,
-0.00981635764190458));
#15543=CARTESIAN_POINT('Ctrl Pts',(-0.000356395749972991,-0.0184527046799012,
-0.00967733079535345));
#15544=CARTESIAN_POINT('Ctrl Pts',(-0.000178150455788198,-0.0184414340252707,
-0.0096583696678918));
#15545=CARTESIAN_POINT('Ctrl Pts',(0.000477888567463474,-0.0183998548353155,
-0.00965830930438933));
#15546=CARTESIAN_POINT('Ctrl Pts',(0.000957709402945352,-0.0183695109173314,
-0.00979879367698402));
#15547=CARTESIAN_POINT('Ctrl Pts',(0.00151241638113353,-0.0183276938099204,
-0.0101552602800974));
#15548=CARTESIAN_POINT('Ctrl Pts',(0.00165318713052002,-0.0183162711544142,
-0.0102687684694766));
#15549=CARTESIAN_POINT('Ctrl Pts',(0.0021243490727292,-0.018273819192397,
-0.0107398907053701));
#15550=CARTESIAN_POINT('Ctrl Pts',(0.00236651757367148,-0.018242731147569,
-0.0111878560810346));
#15551=CARTESIAN_POINT('Ctrl Pts',(0.00250002625799525,-0.0182006750806357,
-0.0118338865874667));
#15552=CARTESIAN_POINT('Ctrl Pts',(0.0025175002847659,-0.0181897612054126,
-0.0120049301415805));
#15553=CARTESIAN_POINT('Ctrl Pts',(0.00251749999999651,-0.0181788400336509,
-0.0121758574807786));
#15554=CARTESIAN_POINT('',(0.0025174996618868,-0.0171788333650338,-0.012176768974368));
#15555=CARTESIAN_POINT('Ctrl Pts',(0.00251749978208517,-0.0181787743898821,
-0.0121769007602343));
#15556=CARTESIAN_POINT('Ctrl Pts',(0.00251729665938466,-0.0181479131488603,
-0.0126650861589615));
#15557=CARTESIAN_POINT('Ctrl Pts',(0.00237080747747283,-0.0181170519078386,
-0.0131531919847914));
#15558=CARTESIAN_POINT('Ctrl Pts',(0.00210238256047418,-0.0180861906668169,
-0.0135606976169483));
#15559=CARTESIAN_POINT('Ctrl Pts',(0.00200844187027922,-0.0180753901557679,
-0.0137033123964226));
#15560=CARTESIAN_POINT('Ctrl Pts',(0.00190002070867247,-0.018064589644719,
-0.0138362025487504));
#15561=CARTESIAN_POINT('Ctrl Pts',(0.0017794943310653,-0.0180537891336701,
-0.0139566413637044));
#15562=CARTESIAN_POINT('Ctrl Pts',(0.00144144917271534,-0.0180234965077712,
-0.0142944409315743));
#15563=CARTESIAN_POINT('Ctrl Pts',(0.00100284143968462,-0.0179932038818723,
-0.0145342429641631));
#15564=CARTESIAN_POINT('Ctrl Pts',(0.000534299314744759,-0.0179629112559734,
-0.014636001756115));
#15565=CARTESIAN_POINT('Ctrl Pts',(0.000358450758299624,-0.0179515421298016,
-0.0146741928508275));
#15566=CARTESIAN_POINT('Ctrl Pts',(0.000178653920795057,-0.0179401730036298,
-0.0146934089138742));
#15567=CARTESIAN_POINT('Ctrl Pts',(-7.82159575315025E-7,-0.017928803877458,
-0.0146933531650539));
#15568=CARTESIAN_POINT('Ctrl Pts',(-0.000480651474567896,-0.0178983992075785,
-0.0146932040749257));
#15569=CARTESIAN_POINT('Ctrl Pts',(-0.000962018237753669,-0.017867994537699,
-0.0145515316086698));
#15570=CARTESIAN_POINT('Ctrl Pts',(-0.0013661713923947,-0.0178375898678195,
-0.0142904175387392));
#15571=CARTESIAN_POINT('Ctrl Pts',(-0.0015158058168978,-0.0178263327856283,
-0.0141937421741279));
#15572=CARTESIAN_POINT('Ctrl Pts',(-0.00165499872077991,-0.0178150757034371,
-0.014081201916579));
#15573=CARTESIAN_POINT('Ctrl Pts',(-0.00178060053003004,-0.0178038186212459,
-0.0139555352813135));
#15574=CARTESIAN_POINT('Ctrl Pts',(-0.00211977937025927,-0.0177734196635815,
-0.0136161813829952));
#15575=CARTESIAN_POINT('Ctrl Pts',(-0.00235997606698392,-0.017743020705917,
-0.0131757254849616));
#15576=CARTESIAN_POINT('Ctrl Pts',(-0.00246117097680353,-0.0177126217482525,
-0.0127054226143519));
#15577=CARTESIAN_POINT('Ctrl Pts',(-0.002498663626283,-0.0177013589538463,
-0.0125311757010596));
#15578=CARTESIAN_POINT('Ctrl Pts',(-0.00251753643997218,-0.0176900961594401,
-0.0123530901387271));
#15579=CARTESIAN_POINT('Ctrl Pts',(-0.00251749994694553,-0.0176788333650338,
-0.0121753364410923));
#15580=CARTESIAN_POINT('Ctrl Pts',(-0.0025174014500777,-0.0176484344073693,
-0.0116955685491982));
#15581=CARTESIAN_POINT('Ctrl Pts',(-0.00237583737863047,-0.0176180354497047,
-0.011214271138594));
#15582=CARTESIAN_POINT('Ctrl Pts',(-0.00211485669286262,-0.0175876364920402,
-0.0108101346410626));
#15583=CARTESIAN_POINT('Ctrl Pts',(-0.00201816351541162,-0.017576373697634,
-0.0106604023267525));
#15584=CARTESIAN_POINT('Ctrl Pts',(-0.00190558679701245,-0.0175651109032279,
-0.0105211191169428));
#15585=CARTESIAN_POINT('Ctrl Pts',(-0.00177986963867943,-0.0175538481088218,
-0.0103954403234208));
#15586=CARTESIAN_POINT('Ctrl Pts',(-0.00144048772692144,-0.0175234434389423,
-0.0100561619800467));
#15587=CARTESIAN_POINT('Ctrl Pts',(-0.00099996244018008,-0.0174930387690628,
-0.00981589679331808));
#15588=CARTESIAN_POINT('Ctrl Pts',(-0.000529570110150823,-0.0174626340991833,
-0.00971468247809419));
#15589=CARTESIAN_POINT('Ctrl Pts',(-0.000355411168703594,-0.0174513770169921,
-0.00967720869956213));
#15590=CARTESIAN_POINT('Ctrl Pts',(-0.00017741619453138,-0.0174401199348009,
-0.00965833554778184));
#15591=CARTESIAN_POINT('Ctrl Pts',(2.51531350274394E-7,-0.0174288628526097,
-0.00965835329912374));
#15592=CARTESIAN_POINT('Ctrl Pts',(0.000478352504853852,-0.0173985702267108,
-0.00965840106769734));
#15593=CARTESIAN_POINT('Ctrl Pts',(0.000958129698327566,-0.0173682776008119,
-0.00979896659453205));
#15594=CARTESIAN_POINT('Ctrl Pts',(0.00136136532735725,-0.0173379849749131,
-0.0100581916763216));
#15595=CARTESIAN_POINT('Ctrl Pts',(0.00151270370121509,-0.0173266158487412,
-0.0101554814481495));
#15596=CARTESIAN_POINT('Ctrl Pts',(0.00165340570642434,-0.0173152467225694,
-0.0102689643764695));
#15597=CARTESIAN_POINT('Ctrl Pts',(0.00178022537647008,-0.0173038775963976,
-0.010395796023723));
#15598=CARTESIAN_POINT('Ctrl Pts',(0.0021244745601289,-0.017273016355376,
-0.0107400777192469));
#15599=CARTESIAN_POINT('Ctrl Pts',(0.00236660208174994,-0.0172421551143543,
-0.0111880604961051));
#15600=CARTESIAN_POINT('Ctrl Pts',(0.00246544689552489,-0.0172112938733326,
-0.0116665617636101));
#15601=CARTESIAN_POINT('Ctrl Pts',(0.00250003962310081,-0.0172004933622836,
-0.0118340228914061));
#15602=CARTESIAN_POINT('Ctrl Pts',(0.00251749906459384,-0.0171896928512346,
-0.0120049892050111));
#15603=CARTESIAN_POINT('Ctrl Pts',(0.00251749999996227,-0.0171788923401855,
-0.0121758395037901));
#15604=CARTESIAN_POINT('',(0.00251749963321368,-0.0161787130482344,-0.0121748985097519));
#15605=CARTESIAN_POINT('Ctrl Pts',(0.00251749932381133,-0.0171787743898821,
-0.012177698444946));
#15606=CARTESIAN_POINT('Ctrl Pts',(0.00251714151439738,-0.0171479040308582,
-0.0126658868647471));
#15607=CARTESIAN_POINT('Ctrl Pts',(0.00237049591654825,-0.0171170336718345,
-0.0131539488348971));
#15608=CARTESIAN_POINT('Ctrl Pts',(0.00210193894734248,-0.0170861633128106,
-0.0135613708474879));
#15609=CARTESIAN_POINT('Ctrl Pts',(0.00200801637077188,-0.0170753670051678,
-0.0137038587720697));
#15610=CARTESIAN_POINT('Ctrl Pts',(0.00189963613076377,-0.0170645706975249,
-0.0138366307209233));
#15611=CARTESIAN_POINT('Ctrl Pts',(0.00177916928923548,-0.0170537743898821,
-0.0139569661101157));
#15612=CARTESIAN_POINT('Ctrl Pts',(0.00144105763519167,-0.0170234726289297,
-0.0142947088197582));
#15613=CARTESIAN_POINT('Ctrl Pts',(0.00100239963061137,-0.0169931708679771,
-0.0145344318790767));
#15614=CARTESIAN_POINT('Ctrl Pts',(0.000533832953673381,-0.0169628691070247,
-0.0146361029949358));
#15615=CARTESIAN_POINT('Ctrl Pts',(0.000358093460758483,-0.0169515042013105,
-0.0146742355195573));
#15616=CARTESIAN_POINT('Ctrl Pts',(0.000178414513428729,-0.0169401392955963,
-0.0146934174733652));
#15617=CARTESIAN_POINT('Ctrl Pts',(-9.03414161335177E-7,-0.0169287743898821,
-0.0146933531244613));
#15618=CARTESIAN_POINT('Ctrl Pts',(-0.000480779152462688,-0.016898360573519,
-0.0146931809192714));
#15619=CARTESIAN_POINT('Ctrl Pts',(-0.000962144144701767,-0.016867946757156,
-0.0145514816527625));
#15620=CARTESIAN_POINT('Ctrl Pts',(-0.00136628727402242,-0.016837532940793,
-0.0142903426657805));
#15621=CARTESIAN_POINT('Ctrl Pts',(-0.00151581675369036,-0.0168262800904893,
-0.01419372348804));
#15622=CARTESIAN_POINT('Ctrl Pts',(-0.00165491782093178,-0.0168150272401857,
-0.0140812611991804));
#15623=CARTESIAN_POINT('Ctrl Pts',(-0.00178044714873814,-0.0168037743898821,
-0.0139556887285443));
#15624=CARTESIAN_POINT('Ctrl Pts',(-0.00211965965503896,-0.016773366296242,
-0.0136163596392294));
#15625=CARTESIAN_POINT('Ctrl Pts',(-0.00235989530171396,-0.0167429582026018,
-0.0131759184826837));
#15626=CARTESIAN_POINT('Ctrl Pts',(-0.00246112875058267,-0.0167125501089617,
-0.0127056188224845));
#15627=CARTESIAN_POINT('Ctrl Pts',(-0.00249861035631251,-0.0167012915359351,
-0.012531490738976));
#15628=CARTESIAN_POINT('Ctrl Pts',(-0.00251749729511135,-0.0166900329629087,
-0.0123535276339294));
#15629=CARTESIAN_POINT('Ctrl Pts',(-0.0025174999997082,-0.0166787743898821,
-0.0121758916167497));
#15630=CARTESIAN_POINT('Ctrl Pts',(-0.0025175073045091,-0.0166483662962419,
-0.011696117436527));
#15631=CARTESIAN_POINT('Ctrl Pts',(-0.00237604584935783,-0.0166179582026016,
-0.0112147838942784));
#15632=CARTESIAN_POINT('Ctrl Pts',(-0.0021151489841834,-0.0165875501089614,
-0.0108105873693435));
#15633=CARTESIAN_POINT('Ctrl Pts',(-0.00201855212271358,-0.0165762915359349,
-0.0106609339202703));
#15634=CARTESIAN_POINT('Ctrl Pts',(-0.00190609068656835,-0.0165650329629086,
-0.0105217122176387));
#15635=CARTESIAN_POINT('Ctrl Pts',(-0.00178050134567524,-0.0165537743898821,
-0.0103960720617867));
#15636=CARTESIAN_POINT('Ctrl Pts',(-0.00144123533548841,-0.0165233605735191,
-0.010056668780489));
#15637=CARTESIAN_POINT('Ctrl Pts',(-0.00100078923118645,-0.0164929467571562,
-0.00981624624970903));
#15638=CARTESIAN_POINT('Ctrl Pts',(-0.000530427177695476,-0.0164625329407932,
-0.00971486704946492));
#15639=CARTESIAN_POINT('Ctrl Pts',(-0.000356397265983295,-0.0164512800904895,
-0.00967735761787496));
#15640=CARTESIAN_POINT('Ctrl Pts',(-0.000178529965730701,-0.0164400272401858,
-0.00965842259834124));
#15641=CARTESIAN_POINT('Ctrl Pts',(-9.80074539332744E-7,-0.0164287743898821,
-0.0096583534773319));
#15642=CARTESIAN_POINT('Ctrl Pts',(0.000477127623938968,-0.0163984726289296,
-0.00965816734775183));
#15643=CARTESIAN_POINT('Ctrl Pts',(0.000956978853136251,-0.0163681708679771,
-0.00979850192424106));
#15644=CARTESIAN_POINT('Ctrl Pts',(0.00136034396970021,-0.0163378691070246,
-0.010057535431726));
#15645=CARTESIAN_POINT('Ctrl Pts',(0.00151162912191674,-0.0163265042013105,
-0.0101546879171538));
#15646=CARTESIAN_POINT('Ctrl Pts',(0.00165229984926619,-0.0163151392955962,
-0.0102680171781157));
#15647=CARTESIAN_POINT('Ctrl Pts',(0.00177911505175044,-0.0163037743898821,
-0.0103946862863487));
#15648=CARTESIAN_POINT('Ctrl Pts',(0.00212358168691954,-0.0162729040308583,
-0.0107387560874303));
#15649=CARTESIAN_POINT('Ctrl Pts',(0.00236598895617194,-0.0162420336718344,
-0.0111865914635291));
#15650=CARTESIAN_POINT('Ctrl Pts',(0.00246513082529533,-0.0162111633128106,
-0.0116650340776605));
#15651=CARTESIAN_POINT('Ctrl Pts',(0.00249980376572062,-0.0162003670051677,
-0.0118323600762862));
#15652=CARTESIAN_POINT('Ctrl Pts',(0.00251736893054138,-0.0161895706975249,
-0.0120031970670941));
#15653=CARTESIAN_POINT('Ctrl Pts',(0.00251749926645723,-0.0161787743898821,
-0.0121739314678082));
#15654=CARTESIAN_POINT('',(0.00251755538663573,-0.015178857044612,-0.0121751343114423));
#15655=CARTESIAN_POINT('Ctrl Pts',(0.00251749999997012,-0.0161786517065868,
-0.0121758655516955));
#15656=CARTESIAN_POINT('Ctrl Pts',(0.00251749762155505,-0.0161477908369676,
-0.0126640508647007));
#15657=CARTESIAN_POINT('Ctrl Pts',(0.00237120923608777,-0.0161169299673483,
-0.0131522167799313));
#15658=CARTESIAN_POINT('Ctrl Pts',(0.00210295203127188,-0.0160860690977291,
-0.0135598326954257));
#15659=CARTESIAN_POINT('Ctrl Pts',(0.0020090673912971,-0.0160752684124856,
-0.0137024900883574));
#15660=CARTESIAN_POINT('Ctrl Pts',(0.00190069746994918,-0.0160644677272422,
-0.0138354282650385));
#15661=CARTESIAN_POINT('Ctrl Pts',(0.00178021660930023,-0.0160536670419987,
-0.0139559193173478));
#15662=CARTESIAN_POINT('Ctrl Pts',(0.00144230871570574,-0.0160233747882719,
-0.0142938557950883));
#15663=CARTESIAN_POINT('Ctrl Pts',(0.00100379856888952,-0.0159930825345452,
-0.0145338356963433));
#15664=CARTESIAN_POINT('Ctrl Pts',(0.000535298010146728,-0.0159627902808184,
-0.0146357846454242));
#15665=CARTESIAN_POINT('Ctrl Pts',(0.000359460187621698,-0.0159514209796825,
-0.0146740481669517));
#15666=CARTESIAN_POINT('Ctrl Pts',(0.000179666165241272,-0.0159400516785465,
-0.014693337223714));
#15667=CARTESIAN_POINT('Ctrl Pts',(2.25215308823281E-7,-0.0159286823774106,
-0.0146933532764842));
#15668=CARTESIAN_POINT('Ctrl Pts',(-0.000479643856273245,-0.0158982780801603,
-0.0146933962055256));
#15669=CARTESIAN_POINT('Ctrl Pts',(-0.000961067062991505,-0.0158678737829099,
-0.0145519165176877));
#15670=CARTESIAN_POINT('Ctrl Pts',(-0.00136532456468596,-0.0158374694856596,
-0.0142909644143869));
#15671=CARTESIAN_POINT('Ctrl Pts',(-0.00151500178961346,-0.0158262122280472,
-0.014194346326912));
#15672=CARTESIAN_POINT('Ctrl Pts',(-0.00165424327245194,-0.0158149549704349,
-0.014081858293453));
#15673=CARTESIAN_POINT('Ctrl Pts',(-0.00177989809173394,-0.0158036977128225,
-0.0139562378048692));
#15674=CARTESIAN_POINT('Ctrl Pts',(-0.00211921063967702,-0.0157732991273554,
-0.0136170179619792));
#15675=CARTESIAN_POINT('Ctrl Pts',(-0.00235958108989582,-0.0157429005418882,
-0.0131766571301363));
#15676=CARTESIAN_POINT('Ctrl Pts',(-0.0024609616650532,-0.0157125019564211,
-0.0127063944566275));
#15677=CARTESIAN_POINT('Ctrl Pts',(-0.00249852414691729,-0.0157012389870255,
-0.0125321575959901));
#15678=CARTESIAN_POINT('Ctrl Pts',(-0.00251746728692474,-0.01568997601763,
-0.0123540745231461));
#15679=CARTESIAN_POINT('Ctrl Pts',(-0.00251749995748017,-0.0156787130482344,
-0.0121763159823111));
#15680=CARTESIAN_POINT('Ctrl Pts',(-0.00251758813481925,-0.0156483144627673,
-0.0116965483467703));
#15681=CARTESIAN_POINT('Ctrl Pts',(-0.00237621148852556,-0.0156179158773003,
-0.0112151960937125));
#15682=CARTESIAN_POINT('Ctrl Pts',(-0.00211538828755822,-0.0155875172918331,
-0.0108109581833133));
#15683=CARTESIAN_POINT('Ctrl Pts',(-0.00201875077350902,-0.0155762543224375,
-0.0106611841348371));
#15684=CARTESIAN_POINT('Ctrl Pts',(-0.00190622477840748,-0.0155649913530419,
-0.0105218535800564));
#15685=CARTESIAN_POINT('Ctrl Pts',(-0.00178055241147931,-0.0155537283836464,
-0.0103961231497185));
#15686=CARTESIAN_POINT('Ctrl Pts',(-0.00144130084592552,-0.0155233240863961,
-0.0100567148424469));
#15687=CARTESIAN_POINT('Ctrl Pts',(-0.00100086800023652,-0.0154929197891457,
-0.00981628074575207));
#15688=CARTESIAN_POINT('Ctrl Pts',(-0.000530514760432268,-0.0154625154918954,
-0.00971488592818791));
#15689=CARTESIAN_POINT('Ctrl Pts',(-0.000356365443784941,-0.015451258234283,
-0.00967734427503011));
#15690=CARTESIAN_POINT('Ctrl Pts',(-0.000178372744225681,-0.0154400009766707,
-0.00965840279886414));
#15691=CARTESIAN_POINT('Ctrl Pts',(-7.00176193161934E-7,-0.0154287437190583,
-0.00965835338392586));
#15692=CARTESIAN_POINT('Ctrl Pts',(0.000477400503071805,-0.0153984514653315,
-0.00965822041283291));
#15693=CARTESIAN_POINT('Ctrl Pts',(0.000957230582051071,-0.0153681592116047,
-0.009798604400552));
#15694=CARTESIAN_POINT('Ctrl Pts',(0.00136056406704873,-0.0153378669578779,
-0.0100576767902633));
#15695=CARTESIAN_POINT('Ctrl Pts',(0.00151194335663502,-0.015326497656742,
-0.0101549119461942));
#15696=CARTESIAN_POINT('Ctrl Pts',(0.00165269182272679,-0.0153151283556061,
-0.0102683451667279));
#15697=CARTESIAN_POINT('Ctrl Pts',(0.00177956216610836,-0.0153037590544702,
-0.0103951329977548));
#15698=CARTESIAN_POINT('Ctrl Pts',(0.0021239394571007,-0.0152728981848508,
-0.0107392863169314));
#15699=CARTESIAN_POINT('Ctrl Pts',(0.00236623382097467,-0.0152420373152316,
-0.0111871787171439));
#15700=CARTESIAN_POINT('Ctrl Pts',(0.00246525692736654,-0.0152111764456122,
-0.0116656430043496));
#15701=CARTESIAN_POINT('Ctrl Pts',(0.00249991302802582,-0.0152003757603689,
-0.0118330959060355));
#15702=CARTESIAN_POINT('Ctrl Pts',(0.0025174361894798,-0.0151895750751254,
-0.0120040605760843));
#15703=CARTESIAN_POINT('Ctrl Pts',(0.00251749982538233,-0.0151787743898821,
-0.012174915629931));
#15704=CARTESIAN_POINT('',(0.00251749939328164,-0.0141788271636735,-0.0121772344157477));
#15705=CARTESIAN_POINT('Ctrl Pts',(0.00251749999999728,-0.0151787156439641,
-0.0121758495859091));
#15706=CARTESIAN_POINT('Ctrl Pts',(0.00251750071291988,-0.0151481640251222,
-0.0126608409072188));
#15707=CARTESIAN_POINT('Ctrl Pts',(0.00237305979471814,-0.0151175938090383,
-0.0131460901801096));
#15708=CARTESIAN_POINT('Ctrl Pts',(0.00210809033725665,-0.0150870046971682,
-0.0135519933157576));
#15709=CARTESIAN_POINT('Ctrl Pts',(0.00201298073055038,-0.015076024871692,
-0.0136976904385964));
#15710=CARTESIAN_POINT('Ctrl Pts',(0.00190281808401211,-0.0150650426116467,
-0.0138333165509995));
#15711=CARTESIAN_POINT('Ctrl Pts',(0.00178015071638259,-0.0150540579032255,
-0.0139559852134002));
#15712=CARTESIAN_POINT('Ctrl Pts',(0.00144068287806857,-0.0150236589854504,
-0.0142954566348445));
#15713=CARTESIAN_POINT('Ctrl Pts',(0.000999660018196464,-0.0149932413169844,
-0.0145361596170759));
#15714=CARTESIAN_POINT('Ctrl Pts',(0.000528147072577002,-0.014962805775685,
-0.0146373298596191));
#15715=CARTESIAN_POINT('Ctrl Pts',(0.000354599300466907,-0.0149516034949533,
-0.0146745671621372));
#15716=CARTESIAN_POINT('Ctrl Pts',(0.000177183293706389,-0.0149403987929458,
-0.0146933526631847));
#15717=CARTESIAN_POINT('Ctrl Pts',(8.8573912000701E-9,-0.014929191713435,
-0.0146933532865425));
#15718=CARTESIAN_POINT('Ctrl Pts',(-0.000329261486051471,-0.0149083638841147,
-0.0146933544450236));
#15719=CARTESIAN_POINT('Ctrl Pts',(-0.000658847952640571,-0.0148875278432613,
-0.0146278709517489));
#15720=CARTESIAN_POINT('Ctrl Pts',(-0.000963399403632745,-0.0148666807812065,
-0.0145017225518179));
#15721=CARTESIAN_POINT('Ctrl Pts',(-0.00126795085462492,-0.0148458337191516,
-0.0143755741518868));
#15722=CARTESIAN_POINT('Ctrl Pts',(-0.00154719964135841,-0.0148249756358953,
-0.0141889354689233));
#15723=CARTESIAN_POINT('Ctrl Pts',(-0.00178013819010309,-0.0148041179574223,
-0.0139559977397238));
#15724=CARTESIAN_POINT('Ctrl Pts',(-0.00189660746447543,-0.0147936891181858,
-0.013839528875124));
#15725=CARTESIAN_POINT('Ctrl Pts',(-0.00200162166373276,-0.0147832603801451,
-0.0137115946618794));
#15726=CARTESIAN_POINT('Ctrl Pts',(-0.00209322290365292,-0.0147728170861969,
-0.0135745041098957));
#15727=CARTESIAN_POINT('Ctrl Pts',(-0.00218482414357308,-0.0147623737922487,
-0.0134374135579119));
#15728=CARTESIAN_POINT('Ctrl Pts',(-0.00226296456431943,-0.0147519159423931,
-0.0132911176945691));
#15729=CARTESIAN_POINT('Ctrl Pts',(-0.002325865875714,-0.0147415032420826,
-0.0131392608732986));
#15730=CARTESIAN_POINT('Ctrl Pts',(-0.00238876718710857,-0.0147310905417721,
-0.0129874040520281));
#15731=CARTESIAN_POINT('Ctrl Pts',(-0.00243667461938459,-0.0147207229910068,
-0.0128301416474611));
#15732=CARTESIAN_POINT('Ctrl Pts',(-0.00246912672741954,-0.0147101764250794,
-0.0126669942581156));
#15733=CARTESIAN_POINT('Ctrl Pts',(-0.00248535278143701,-0.0147049031421157,
-0.0125854205634429));
#15734=CARTESIAN_POINT('Ctrl Pts',(-0.00249752695350485,-0.0146995851053614,
-0.0125023196953955));
#15735=CARTESIAN_POINT('Ctrl Pts',(-0.00250537749513714,-0.0146945081517445,
-0.0124226119882493));
#15736=CARTESIAN_POINT('Ctrl Pts',(-0.00250930276595329,-0.014691969674936,
-0.0123827581346762));
#15737=CARTESIAN_POINT('Ctrl Pts',(-0.00251228671057559,-0.0146894914689118,
-0.0123437732872266));
#15738=CARTESIAN_POINT('Ctrl Pts',(-0.00251446754741514,-0.0146866727988687,
-0.0122993814331324));
#15739=CARTESIAN_POINT('Ctrl Pts',(-0.00251664838425469,-0.0146838541288256,
-0.0122549895790381));
#15740=CARTESIAN_POINT('Ctrl Pts',(-0.0025175,-0.0146806949947635,-0.0122051596879933));
#15741=CARTESIAN_POINT('Ctrl Pts',(-0.0025175,-0.0146788366351873,-0.0121758532865581));
#15742=CARTESIAN_POINT('Ctrl Pts',(-0.0025175,-0.0146769782756111,-0.0121465468851228));
#15743=CARTESIAN_POINT('Ctrl Pts',(-0.00251725426100465,-0.0146764206905208,
-0.0121377557191278));
#15744=CARTESIAN_POINT('Ctrl Pts',(-0.00251694772361996,-0.0146754929894721,
-0.0121231237259275));
#15745=CARTESIAN_POINT('Ctrl Pts',(-0.00251664118623527,-0.0146745652884234,
-0.0121084917327271));
#15746=CARTESIAN_POINT('Ctrl Pts',(-0.00251604607189495,-0.0146732674714164,
-0.0120880271427794));
#15747=CARTESIAN_POINT('Ctrl Pts',(-0.00251519594101278,-0.0146720075132562,
-0.012068170287376));
#15748=CARTESIAN_POINT('Ctrl Pts',(-0.00251349567924844,-0.0146694875969357,
-0.0120284565765692));
#15749=CARTESIAN_POINT('Ctrl Pts',(-0.00251102772241131,-0.0146671191160024,
-0.0119911552048106));
#15750=CARTESIAN_POINT('Ctrl Pts',(-0.00250750307707114,-0.0146646110693223,
-0.0119517225914742));
#15751=CARTESIAN_POINT('Ctrl Pts',(-0.00250045378639079,-0.0146595949759621,
-0.0118728573648014));
#15752=CARTESIAN_POINT('Ctrl Pts',(-0.00248880263071647,-0.0146540206196144,
-0.0117855188015991));
#15753=CARTESIAN_POINT('Ctrl Pts',(-0.00247095694289093,-0.0146481162154468,
-0.0116940047248926));
#15754=CARTESIAN_POINT('Ctrl Pts',(-0.0024531112550654,-0.0146422118112792,
-0.0116024906481861));
#15755=CARTESIAN_POINT('Ctrl Pts',(-0.00242921266780654,-0.0146359773592916,
-0.0115067594572136));
#15756=CARTESIAN_POINT('Ctrl Pts',(-0.0023972519619071,-0.0146293520735607,
-0.0114070950143213));
#15757=CARTESIAN_POINT('Ctrl Pts',(-0.00236529125600766,-0.0146227267878298,
-0.0113074305714289));
#15758=CARTESIAN_POINT('Ctrl Pts',(-0.00232522920184558,-0.0146157106683554,
-0.0112038539433981));
#15759=CARTESIAN_POINT('Ctrl Pts',(-0.0022751852637213,-0.0146083186436641,
-0.01109819922994));
#15760=CARTESIAN_POINT('Ctrl Pts',(-0.00217509738747274,-0.0145935345942814,
-0.0108868898030238));
#15761=CARTESIAN_POINT('Ctrl Pts',(-0.00203504218911522,-0.0145772469240307,
-0.0106673103909374));
#15762=CARTESIAN_POINT('Ctrl Pts',(-0.00184324713000241,-0.0145594439198393,
-0.0104611386549829));
#15763=CARTESIAN_POINT('Ctrl Pts',(-0.0016514520708896,-0.014541640915648,
-0.0102549669190285));
#15764=CARTESIAN_POINT('Ctrl Pts',(-0.00140748406223656,-0.0145223225775161,
-0.0100626956686912));
#15765=CARTESIAN_POINT('Ctrl Pts',(-0.00111175942872558,-0.0145014920439725,
-0.00991713745169976));
#15766=CARTESIAN_POINT('Ctrl Pts',(-0.000816034795214608,-0.014480661510429,
-0.00977157923470835));
#15767=CARTESIAN_POINT('Ctrl Pts',(-0.000468174670655183,-0.014458318781474,
-0.00967362327560147));
#15768=CARTESIAN_POINT('Ctrl Pts',(-9.0880954173227E-5,-0.0144344630160636,
-0.00965999420819767));
#15769=CARTESIAN_POINT('Ctrl Pts',(0.000286412762308729,-0.0144106072506532,
-0.00964636514079386));
#15770=CARTESIAN_POINT('Ctrl Pts',(0.000693089871217907,-0.0143852384487876,
-0.00971851511006437));
#15771=CARTESIAN_POINT('Ctrl Pts',(0.00107766354684713,-0.0143583568361125,
-0.00990067251796038));
#15772=CARTESIAN_POINT('Ctrl Pts',(0.00146223722247635,-0.0143314752234374,
-0.0100828299258564));
#15773=CARTESIAN_POINT('Ctrl Pts',(0.00182358312527259,-0.014303080799953,
-0.0103768885650704));
#15774=CARTESIAN_POINT('Ctrl Pts',(0.00208795759600706,-0.0142731735041193,
-0.0107693543255644));
#15775=CARTESIAN_POINT('Ctrl Pts',(0.00233330315158756,-0.0142454188495498,
-0.0111335715277292));
#15776=CARTESIAN_POINT('Ctrl Pts',(0.00249357887136464,-0.0142163612692967,
-0.0115834060038655));
#15777=CARTESIAN_POINT('Ctrl Pts',(0.00251499973632202,-0.0141860007797548,
-0.012063681203132));
#15778=CARTESIAN_POINT('Ctrl Pts',(0.00251666095110628,-0.0141836462859384,
-0.012100927143626));
#15779=CARTESIAN_POINT('Ctrl Pts',(0.0025175001312269,-0.0141812839561704,
-0.0121383331360715));
#15780=CARTESIAN_POINT('Ctrl Pts',(0.00251749999998461,-0.0141789137904583,
-0.0121758620904934));
#15781=CARTESIAN_POINT('',(0.0025175,-0.0131787743898721,-0.012175853286558));
#15782=CARTESIAN_POINT('Ctrl Pts',(0.00251749902367291,-0.0141787743898821,
-0.0121780704482395));
#15783=CARTESIAN_POINT('Ctrl Pts',(0.00251706907769517,-0.0141479071685421,
-0.012666257028528));
#15784=CARTESIAN_POINT('Ctrl Pts',(0.00237035237263466,-0.0141170399472022,
-0.013154295843589));
#15785=CARTESIAN_POINT('Ctrl Pts',(0.00210173688987106,-0.0140861727258623,
-0.0135616773359075));
#15786=CARTESIAN_POINT('Ctrl Pts',(0.00200775699488553,-0.0140753732805355,
-0.0137042069826473));
#15787=CARTESIAN_POINT('Ctrl Pts',(0.00189930957625436,-0.0140645738352088,
-0.0138370109335702));
#15788=CARTESIAN_POINT('Ctrl Pts',(0.00177876899422965,-0.0140537743898821,
-0.0139573658784775));
#15789=CARTESIAN_POINT('Ctrl Pts',(0.00144058422971941,-0.0140234758148021,
-0.0142950298254853));
#15790=CARTESIAN_POINT('Ctrl Pts',(0.00100187609621577,-0.0139931772397221,
-0.0145346536854798));
#15791=CARTESIAN_POINT('Ctrl Pts',(0.000533290013078261,-0.013962878664642,
-0.0146362207412183));
#15792=CARTESIAN_POINT('Ctrl Pts',(0.00035747549060425,-0.0139515105730554,
-0.0146743289225031));
#15793=CARTESIAN_POINT('Ctrl Pts',(0.00017772270395627,-0.0139401424814687,
-0.0146934712260336));
#15794=CARTESIAN_POINT('Ctrl Pts',(-1.66287135762318E-6,-0.0139287743898821,
-0.0146933527373741));
#15795=CARTESIAN_POINT('Ctrl Pts',(-0.000481534852372283,-0.0138983637583667,
-0.0146930357699276));
#15796=CARTESIAN_POINT('Ctrl Pts',(-0.000962854182385809,-0.0138679531268514,
-0.0145511933676515));
#15797=CARTESIAN_POINT('Ctrl Pts',(-0.00136691705462027,-0.013837542495336,
-0.0142899355971099));
#15798=CARTESIAN_POINT('Ctrl Pts',(-0.00151647481342291,-0.0138262864601847,
-0.0141932349860988));
#15799=CARTESIAN_POINT('Ctrl Pts',(-0.00165559143238043,-0.0138150304250334,
-0.014080682226469));
#15800=CARTESIAN_POINT('Ctrl Pts',(-0.00178112090832962,-0.0138037743898821,
-0.0139550144821531));
#15801=CARTESIAN_POINT('Ctrl Pts',(-0.00212020238086612,-0.0137733694754573,
-0.0136155595177253));
#15802=CARTESIAN_POINT('Ctrl Pts',(-0.00236027068215153,-0.0137429645610325,
-0.0131750308481881));
#15803=CARTESIAN_POINT('Ctrl Pts',(-0.00246132719935155,-0.0137125596466076,
-0.0127046960493263));
#15804=CARTESIAN_POINT('Ctrl Pts',(-0.00249875777531793,-0.0137012978943658,
-0.0125304875677141));
#15805=CARTESIAN_POINT('Ctrl Pts',(-0.00251757800760962,-0.013690036142124,
-0.0123524481141251));
#15806=CARTESIAN_POINT('Ctrl Pts',(-0.00251749975591821,-0.0136787743898821,
-0.0121747447056049));
#15807=CARTESIAN_POINT('Ctrl Pts',(-0.00251728848897417,-0.0136483694754573,
-0.0116949741678561));
#15808=CARTESIAN_POINT('Ctrl Pts',(-0.00237560978566041,-0.0136179645610324,
-0.0112137079417602));
#15809=CARTESIAN_POINT('Ctrl Pts',(-0.00211453184685873,-0.0135875596466076,
-0.0108096317384115));
#15810=CARTESIAN_POINT('Ctrl Pts',(-0.00201783053661956,-0.0135762978943657,
-0.0106599649435852));
#15811=CARTESIAN_POINT('Ctrl Pts',(-0.00190525722781884,-0.013565036142124,
-0.0105207450621084));
#15812=CARTESIAN_POINT('Ctrl Pts',(-0.00177955331071196,-0.0135537743898821,
-0.0103951241481617));
#15813=CARTESIAN_POINT('Ctrl Pts',(-0.00144010919747922,-0.0135233637583667,
-0.010055904172209));
#15814=CARTESIAN_POINT('Ctrl Pts',(-0.000999538623246463,-0.0134929531268514,
-0.00981571681272789));
#15815=CARTESIAN_POINT('Ctrl Pts',(-0.00052912589697104,-0.013462542495336,
-0.00971458693868865));
#15816=CARTESIAN_POINT('Ctrl Pts',(-0.000355009743549373,-0.0134512864601847,
-0.00967715524587891));
#15817=CARTESIAN_POINT('Ctrl Pts',(-0.000177063097394015,-0.0134400304250334,
-0.00965831424067397));
#15818=CARTESIAN_POINT('Ctrl Pts',(5.54290495030118E-7,-0.0134287743898821,
-0.00965835334757854));
#15819=CARTESIAN_POINT('Ctrl Pts',(0.000478658142352042,-0.0133984758148021,
-0.00965845861408386));
#15820=CARTESIAN_POINT('Ctrl Pts',(0.000958420702075833,-0.013368177239722,
-0.00979908345595051));
#15821=CARTESIAN_POINT('Ctrl Pts',(0.0013616263130965,-0.0133378786646419,
-0.0100583594770079));
#15822=CARTESIAN_POINT('Ctrl Pts',(0.00151290993954471,-0.0133265105730553,
-0.0101556404067483));
#15823=CARTESIAN_POINT('Ctrl Pts',(0.00165356124644845,-0.0133151424814687,
-0.010269103995322));
#15824=CARTESIAN_POINT('Ctrl Pts',(0.00178033728213873,-0.0133037743898821,
-0.0103959079469965));
#15825=CARTESIAN_POINT('Ctrl Pts',(0.00212456603191952,-0.0132729071685422,
-0.0107402124956799));
#15826=CARTESIAN_POINT('Ctrl Pts',(0.00236666557989477,-0.0132420399472021,
-0.0111882120610907));
#15827=CARTESIAN_POINT('Ctrl Pts',(0.0024654797540446,-0.0132111727258622,
-0.0116667208554597));
#15828=CARTESIAN_POINT('Ctrl Pts',(0.00250005164697466,-0.0132003732805357,
-0.0118341356514375));
#15829=CARTESIAN_POINT('Ctrl Pts',(0.00251750000000004,-0.0131895738352092,
-0.0120050524791417));
#15830=CARTESIAN_POINT('Ctrl Pts',(0.0025175,-0.0131787743898827,-0.0121758532865587));
#15831=CARTESIAN_POINT('',(0.00178084802570376,-0.013178793072307,-0.0139565263307246));
#15832=CARTESIAN_POINT('Origin',(0.,-0.0131787743898824,-0.012175853286568));
#15833=CARTESIAN_POINT('',(0.00251749951162147,-0.0133037004643823,-0.0121747621479011));
#15834=CARTESIAN_POINT('Ctrl Pts',(0.00178027729478665,-0.0131787974308209,
-0.0139558586246588));
#15835=CARTESIAN_POINT('Ctrl Pts',(0.00213502811265273,-0.0132107157510099,
-0.013601053606474));
#15836=CARTESIAN_POINT('Ctrl Pts',(0.00237986623540055,-0.0132435981229686,
-0.013138028295549));
#15837=CARTESIAN_POINT('Ctrl Pts',(0.00247338372893183,-0.0132748262662687,
-0.0126450858296061));
#15838=CARTESIAN_POINT('Ctrl Pts',(0.00250270547493553,-0.0132846176288409,
-0.0124905272199275));
#15839=CARTESIAN_POINT('Ctrl Pts',(0.00251750034288861,-0.0132942463656009,
-0.0123332009389632));
#15840=CARTESIAN_POINT('Ctrl Pts',(0.00251749999999402,-0.0133036317703176,
-0.0121758478005721));
#15841=CARTESIAN_POINT('',(0.0025174998365065,-0.0143038157113684,-0.0121764859784127));
#15842=CARTESIAN_POINT('Ctrl Pts',(0.00251749898605663,-0.0133037743898821,
-0.0121735938167424));
#15843=CARTESIAN_POINT('Ctrl Pts',(0.00251706083443314,-0.0133346442943258,
-0.0116854057204819));
#15844=CARTESIAN_POINT('Ctrl Pts',(0.00237033506334122,-0.0133655141987695,
-0.0111973681052421));
#15845=CARTESIAN_POINT('Ctrl Pts',(0.00210171129165819,-0.0133963841032132,
-0.0107899904158106));
#15846=CARTESIAN_POINT('Ctrl Pts',(0.00200776001313763,-0.0134071808654362,
-0.010647509895479));
#15847=CARTESIAN_POINT('Ctrl Pts',(0.00189935103424433,-0.0134179776276591,
-0.0105147488285564));
#15848=CARTESIAN_POINT('Ctrl Pts',(0.00177885628403369,-0.0134287743898821,
-0.0103944278542837));
#15849=CARTESIAN_POINT('Ctrl Pts',(0.0014406856893849,-0.0134590756892734,
-0.0100567449648021));
#15850=CARTESIAN_POINT('Ctrl Pts',(0.0010019861077406,-0.0134893769886648,
-0.00981709907992996));
#15851=CARTESIAN_POINT('Ctrl Pts',(0.000533402069157638,-0.0135196782880561,
-0.00971551012296925));
#15852=CARTESIAN_POINT('Ctrl Pts',(0.000357646249941188,-0.0135310436553314,
-0.00967740628484457));
#15853=CARTESIAN_POINT('Ctrl Pts',(0.000177953861841114,-0.0135424090226068,
-0.00965825579838605));
#15854=CARTESIAN_POINT('Ctrl Pts',(-1.37385441371961E-6,-0.0135537743898821,
-0.00965835366142921));
#15855=CARTESIAN_POINT('Ctrl Pts',(-0.00048124901856916,-0.0135841877448327,
-0.00965861553976505));
#15856=CARTESIAN_POINT('Ctrl Pts',(-0.000962587104117076,-0.0136146010997832,
-0.00980040445547009));
#15857=CARTESIAN_POINT('Ctrl Pts',(-0.0013666812162148,-0.0136450144547338,
-0.0100616185069639));
#15858=CARTESIAN_POINT('Ctrl Pts',(-0.00151620095888938,-0.0136562677664499,
-0.0101582708871721));
#15859=CARTESIAN_POINT('Ctrl Pts',(-0.00165528817767921,-0.013667521078166,
-0.0102707661943849));
#15860=CARTESIAN_POINT('Ctrl Pts',(-0.00178079954929275,-0.0136787743898821,
-0.0103963704360538));
#15861=CARTESIAN_POINT('Ctrl Pts',(-0.00211994448965385,-0.0137091820229257,
-0.0107357663210824));
#15862=CARTESIAN_POINT('Ctrl Pts',(-0.00236009283512154,-0.0137395896559693,
-0.011176254544861));
#15863=CARTESIAN_POINT('Ctrl Pts',(-0.00246123332061233,-0.0137699972890129,
-0.0116465737843028));
#15864=CARTESIAN_POINT('Ctrl Pts',(-0.00249868260596648,-0.0137812563226359,
-0.0118207188788209));
#15865=CARTESIAN_POINT('Ctrl Pts',(-0.00251753440491855,-0.013792515356259,
-0.0119986957463653));
#15866=CARTESIAN_POINT('Ctrl Pts',(-0.00251749995265597,-0.0138037743898821,
-0.0121763415253998));
#15867=CARTESIAN_POINT('Ctrl Pts',(-0.00251740690632599,-0.0138341820229257,
-0.0126561151757386));
#15868=CARTESIAN_POINT('Ctrl Pts',(-0.00237584506952176,-0.0138645896559693,
-0.0131374187103319));
#15869=CARTESIAN_POINT('Ctrl Pts',(-0.00211486410742613,-0.0138949972890129,
-0.013541560450309));
#15870=CARTESIAN_POINT('Ctrl Pts',(-0.00201823069228971,-0.0139062563226359,
-0.0136912020035456));
#15871=CARTESIAN_POINT('Ctrl Pts',(-0.00190573312061065,-0.013917515356259,
-0.0138304073426009));
#15872=CARTESIAN_POINT('Ctrl Pts',(-0.00178010919676054,-0.0139287743898821,
-0.0139560267324921));
#15873=CARTESIAN_POINT('Ctrl Pts',(-0.00144076879560054,-0.0139591877448326,
-0.0142953548863397));
#15874=CARTESIAN_POINT('Ctrl Pts',(-0.00100027024108851,-0.0139896010997831,
-0.0145356802908132));
#15875=CARTESIAN_POINT('Ctrl Pts',(-0.000529886334566621,-0.0140200144547337,
-0.0146369560317598));
#15876=CARTESIAN_POINT('Ctrl Pts',(-0.000355838560653692,-0.0140312677664498,
-0.0146744292892815));
#15877=CARTESIAN_POINT('Ctrl Pts',(-0.000177957055843198,-0.0140425210781659,
-0.0146933252281468));
#15878=CARTESIAN_POINT('Ctrl Pts',(-3.97376790599182E-7,-0.0140537743898821,
-0.014693353255196));
#15879=CARTESIAN_POINT('Ctrl Pts',(0.000477709791170785,-0.0140840756892734,
-0.0146934287224032));
#15880=CARTESIAN_POINT('Ctrl Pts',(0.000957528083984738,-0.0141143769886648,
-0.0145529833977446));
#15881=CARTESIAN_POINT('Ctrl Pts',(0.00136083300869463,-0.0141446782880562,
-0.0142938570099843));
#15882=CARTESIAN_POINT('Ctrl Pts',(0.00151210403288667,-0.0141560436553315,
-0.0141966642615945));
#15883=CARTESIAN_POINT('Ctrl Pts',(0.00165275572478575,-0.0141674090226068,
-0.0140832954048709));
#15884=CARTESIAN_POINT('Ctrl Pts',(0.00177954712227563,-0.0141787743898821,
-0.0139565886092831));
#15885=CARTESIAN_POINT('Ctrl Pts',(0.00212393003837453,-0.0142096442943259,
-0.0136124354836143));
#15886=CARTESIAN_POINT('Ctrl Pts',(0.0023662286154867,-0.0142405141987698,
-0.013164541615454));
#15887=CARTESIAN_POINT('Ctrl Pts',(0.00246525451638777,-0.0142713841032136,
-0.0126860752181033));
#15888=CARTESIAN_POINT('Ctrl Pts',(0.00249988886739057,-0.0142821808654364,
-0.0125187313919113));
#15889=CARTESIAN_POINT('Ctrl Pts',(0.00251741265685568,-0.0142929776276592,
-0.0123478803200529));
#15890=CARTESIAN_POINT('Ctrl Pts',(0.00251749967307457,-0.0143037743898821,
-0.0121771362789318));
#15891=CARTESIAN_POINT('',(0.00251749973816877,-0.0153038253093176,-0.0121766683770049));
#15892=CARTESIAN_POINT('Ctrl Pts',(0.00251749999993842,-0.0143038570328546,
-0.0121758356778936));
#15893=CARTESIAN_POINT('Ctrl Pts',(0.0025174965853186,-0.0143347205377646,
-0.0116876495701149));
#15894=CARTESIAN_POINT('Ctrl Pts',(0.002371206713351,-0.0143655840426746,
-0.011199483304505));
#15895=CARTESIAN_POINT('Ctrl Pts',(0.00210294789098424,-0.0143964475475845,
-0.0107918675865579));
#15896=CARTESIAN_POINT('Ctrl Pts',(0.00200907910578422,-0.014407247265884,
-0.0106492352140807));
#15897=CARTESIAN_POINT('Ctrl Pts',(0.0019007301047126,-0.0144180469841836,
-0.0105163187080229));
#15898=CARTESIAN_POINT('Ctrl Pts',(0.00178027394343148,-0.014428846702483,
-0.0103958445965965));
#15899=CARTESIAN_POINT('Ctrl Pts',(0.00144237569619611,-0.0144591415902266,
-0.0100578959964145));
#15900=CARTESIAN_POINT('Ctrl Pts',(0.0010038716150532,-0.0144894364779702,
-0.00981790169375985));
#15901=CARTESIAN_POINT('Ctrl Pts',(0.000535372809709038,-0.0145197313657138,
-0.0097159382057831));
#15902=CARTESIAN_POINT('Ctrl Pts',(0.000359565867310013,-0.0145310997011797,
-0.00967767580499775));
#15903=CARTESIAN_POINT('Ctrl Pts',(0.000179803488936402,-0.0145424680366456,
-0.00965838130553472));
#15904=CARTESIAN_POINT('Ctrl Pts',(3.92733717786047E-7,-0.0145538363721115,
-0.00965835331719161));
#15905=CARTESIAN_POINT('Ctrl Pts',(-0.000479477977530979,-0.0145842433074097,
-0.00965827845665108));
#15906=CARTESIAN_POINT('Ctrl Pts',(-0.000960911889368447,-0.0146146502427079,
-0.0097997270328723));
#15907=CARTESIAN_POINT('Ctrl Pts',(-0.00136518740714128,-0.014645057178006,
-0.0100606536285157));
#15908=CARTESIAN_POINT('Ctrl Pts',(-0.00151484542360727,-0.0146563134659173,
-0.0101572455689882));
#15909=CARTESIAN_POINT('Ctrl Pts',(-0.00165407229727665,-0.0146675697538286,
-0.0102697027086086));
#15910=CARTESIAN_POINT('Ctrl Pts',(-0.00177971848881848,-0.0146788260417399,
-0.010395289232513));
#15911=CARTESIAN_POINT('Ctrl Pts',(-0.00211906638382967,-0.0147092272625128,
-0.0107344759759053));
#15912=CARTESIAN_POINT('Ctrl Pts',(-0.00235948150774078,-0.0147396284832857,
-0.0111748140816622));
#15913=CARTESIAN_POINT('Ctrl Pts',(-0.00246090901105393,-0.0147700297040585,
-0.0116450679351084));
#15914=CARTESIAN_POINT('Ctrl Pts',(-0.00249848239660917,-0.0147812917064951,
-0.0118192714673577));
#15915=CARTESIAN_POINT('Ctrl Pts',(-0.00251744317698114,-0.0147925537089318,
-0.0119973217499119));
#15916=CARTESIAN_POINT('Ctrl Pts',(-0.00251749987191038,-0.0148038157113684,
-0.0121750502104685));
#15917=CARTESIAN_POINT('Ctrl Pts',(-0.0025176529170789,-0.0148342169321413,
-0.0126548194342313));
#15918=CARTESIAN_POINT('Ctrl Pts',(-0.00237634045289419,-0.0148646181529143,
-0.0131361920566667));
#15919=CARTESIAN_POINT('Ctrl Pts',(-0.0021155705531048,-0.0148950193736872,
-0.0135404658633856));
#15920=CARTESIAN_POINT('Ctrl Pts',(-0.00201896945709177,-0.0149062813761238,
-0.013690227369027));
#15921=CARTESIAN_POINT('Ctrl Pts',(-0.00190648390638609,-0.0149175433785602,
-0.0138295510692772));
#15922=CARTESIAN_POINT('Ctrl Pts',(-0.00178085411735329,-0.0149288053809968,
-0.0139552815269505));
#15923=CARTESIAN_POINT('Ctrl Pts',(-0.00144165894418808,-0.014959212316295,
-0.0142947485012323));
#15924=CARTESIAN_POINT('Ctrl Pts',(-0.00100126530635152,-0.0149896192515932,
-0.0145352575277486));
#15925=CARTESIAN_POINT('Ctrl Pts',(-0.000530927814105084,-0.0150200261868913,
-0.0146367315659961));
#15926=CARTESIAN_POINT('Ctrl Pts',(-0.000356814435815436,-0.0150312824748026,
-0.0146742960551113));
#15927=CARTESIAN_POINT('Ctrl Pts',(-0.000178855863209009,-0.0150425387627139,
-0.0146932673716284));
#15928=CARTESIAN_POINT('Ctrl Pts',(-1.21341844005783E-6,-0.0150537950506252,
-0.0146933529941282));
#15929=CARTESIAN_POINT('Ctrl Pts',(0.000476888951114326,-0.0150840899383688,
-0.0146935834363522));
#15930=CARTESIAN_POINT('Ctrl Pts',(0.000956749001387523,-0.0151143848261125,
-0.0145532963079935));
#15931=CARTESIAN_POINT('Ctrl Pts',(0.00136013598984903,-0.0151446797138561,
-0.0142943046877277));
#15932=CARTESIAN_POINT('Ctrl Pts',(0.00151150933858718,-0.015156048049322,
-0.0141971165533154));
#15933=CARTESIAN_POINT('Ctrl Pts',(0.0016522587497757,-0.0151674163847878,
-0.0140837337046568));
#15934=CARTESIAN_POINT('Ctrl Pts',(0.00177913794469099,-0.0151787847202537,
-0.0139569974199063));
#15935=CARTESIAN_POINT('Ctrl Pts',(0.0021235979289153,-0.0152096482251635,
-0.0136129254175978));
#15936=CARTESIAN_POINT('Ctrl Pts',(0.00236599908946475,-0.0152405117300734,
-0.0131650898075971));
#15937=CARTESIAN_POINT('Ctrl Pts',(0.00246513583155777,-0.0152713752349833,
-0.0126866483354475));
#15938=CARTESIAN_POINT('Ctrl Pts',(0.00249982563399178,-0.0152821749532829,
-0.012519232705332));
#15939=CARTESIAN_POINT('Ctrl Pts',(0.00251738929573821,-0.0152929746715825,
-0.0123483024723817));
#15940=CARTESIAN_POINT('Ctrl Pts',(0.00251749947634573,-0.0153037743898821,
-0.0121774770473163));
#15941=CARTESIAN_POINT('',(0.00251749964728232,-0.0163037152489246,-0.0121749072438898));
#15942=CARTESIAN_POINT('Ctrl Pts',(0.00251749999999181,-0.0153038762287532,
-0.0121758597066935));
#15943=CARTESIAN_POINT('Ctrl Pts',(0.00251750124987346,-0.015334773828238,
-0.0116857490092181));
#15944=CARTESIAN_POINT('Ctrl Pts',(0.00237009877551313,-0.0153656931543452,
-0.0111958220961543));
#15945=CARTESIAN_POINT('Ctrl Pts',(0.00209985358181042,-0.0153966188415361,
-0.0107871772318362));
#15946=CARTESIAN_POINT('Ctrl Pts',(0.00200668698258001,-0.0154072804228392,
-0.0106462975670405));
#15947=CARTESIAN_POINT('Ctrl Pts',(0.0018993619470655,-0.0154179427601664,
-0.0105149344514446));
#15948=CARTESIAN_POINT('Ctrl Pts',(0.00178015521674487,-0.0154286052239324,
-0.0103957258601372));
#15949=CARTESIAN_POINT('Ctrl Pts',(0.0014437994054449,-0.0154586906196211,
-0.010059364797844));
#15950=CARTESIAN_POINT('Ctrl Pts',(0.00100771648424144,-0.0154887770219555,
-0.0098200625804111));
#15951=CARTESIAN_POINT('Ctrl Pts',(0.000541997348581827,-0.0155189068606704,
-0.00971738930998039));
#15952=CARTESIAN_POINT('Ctrl Pts',(0.000363889698180644,-0.015530429588361,
-0.00967812338003418));
#15953=CARTESIAN_POINT('Ctrl Pts',(0.000181723932839053,-0.015541958668931,
-0.00965835423216842));
#15954=CARTESIAN_POINT('Ctrl Pts',(1.31004198167687E-8,-0.015553496475643,
-0.00965835328659218));
#15955=CARTESIAN_POINT('Ctrl Pts',(-0.000471589952940902,-0.0155834411124158,
-0.00965835083249169));
#15956=CARTESIAN_POINT('Ctrl Pts',(-0.000945830025214709,-0.0156134445270603,
-0.00979520887204593));
#15957=CARTESIAN_POINT('Ctrl Pts',(-0.00134601620199894,-0.0156433545931743,
-0.0100484025505935));
#15958=CARTESIAN_POINT('Ctrl Pts',(-0.0015032117943325,-0.0156551034511616,
-0.0101478585852677));
#15959=CARTESIAN_POINT('Ctrl Pts',(-0.00164912550741972,-0.0156668379057812,
-0.0102646968324588));
#15960=CARTESIAN_POINT('Ctrl Pts',(-0.00178013668995606,-0.0156785487368522,
-0.0103957073332519));
#15961=CARTESIAN_POINT('Ctrl Pts',(-0.00201240543112207,-0.0156993107812687,
-0.0106279748657605));
#15962=CARTESIAN_POINT('Ctrl Pts',(-0.00219837348351843,-0.0157199985733812,
-0.0109046529700258));
#15963=CARTESIAN_POINT('Ctrl Pts',(-0.00232586546977604,-0.0157411352460187,
-0.0112124447197997));
#15964=CARTESIAN_POINT('Ctrl Pts',(-0.00244671118957433,-0.0157611700458049,
-0.0115041910219888));
#15965=CARTESIAN_POINT('Ctrl Pts',(-0.00251113007154686,-0.015781608144953,
-0.0118262264809469));
#15966=CARTESIAN_POINT('Ctrl Pts',(-0.00251701645338492,-0.015800635682678,
-0.0121265134102956));
#15967=CARTESIAN_POINT('Ctrl Pts',(-0.00251734019229965,-0.0158016821581841,
-0.0121430285748379));
#15968=CARTESIAN_POINT('Ctrl Pts',(-0.0025175,-0.0158027243670605,-0.0121594779400862));
#15969=CARTESIAN_POINT('Ctrl Pts',(-0.0025175,-0.0158037620075599,-0.0121758532865581));
#15970=CARTESIAN_POINT('Ctrl Pts',(-0.0025175,-0.015823666543301,-0.0124899733207367));
#15971=CARTESIAN_POINT('Ctrl Pts',(-0.0024630951558248,-0.0158418900616207,
-0.0127769085051407));
#15972=CARTESIAN_POINT('Ctrl Pts',(-0.00235775854945272,-0.0158608768294718,
-0.0130583389082441));
#15973=CARTESIAN_POINT('Ctrl Pts',(-0.00225242194308064,-0.0158798635973229,
-0.0133397693113476));
#15974=CARTESIAN_POINT('Ctrl Pts',(-0.00209100657981397,-0.0158996136147054,
-0.0136125856001859));
#15975=CARTESIAN_POINT('Ctrl Pts',(-0.0018823955451073,-0.0159195265353501,
-0.0138474971666235));
#15976=CARTESIAN_POINT('Ctrl Pts',(-0.00155812287986674,-0.0159504799116144,
-0.0142126523457428));
#15977=CARTESIAN_POINT('Ctrl Pts',(-0.00111876532461567,-0.0159818269067479,
-0.0144870957714781));
#15978=CARTESIAN_POINT('Ctrl Pts',(-0.000629171305823964,-0.0160137889809416,
-0.0146134647646095));
#15979=CARTESIAN_POINT('Ctrl Pts',(-0.00048883424627106,-0.0160229505787908,
-0.0146496871289236));
#15980=CARTESIAN_POINT('Ctrl Pts',(-0.000344620800036344,-0.0160321627129445,
-0.014673952015472));
#15981=CARTESIAN_POINT('Ctrl Pts',(-0.000198603736845032,-0.016041430599005,
-0.0146855072080603));
#15982=CARTESIAN_POINT('Ctrl Pts',(0.000259338701600219,-0.0160704967796899,
-0.0147217468978262));
#15983=CARTESIAN_POINT('Ctrl Pts',(0.000738899690729382,-0.0161001113311382,
-0.0146292770516161));
#15984=CARTESIAN_POINT('Ctrl Pts',(0.00116198117812939,-0.0161302303745341,
-0.0144091481599846));
#15985=CARTESIAN_POINT('Ctrl Pts',(0.0013444321136084,-0.0161432190015645,
-0.0143142191134528));
#15986=CARTESIAN_POINT('Ctrl Pts',(0.00151628576184183,-0.016156301449233,
-0.0141962146500593));
#15987=CARTESIAN_POINT('Ctrl Pts',(0.00167165393585948,-0.0161694741985248,
-0.0140582399016628));
#15988=CARTESIAN_POINT('Ctrl Pts',(0.00202224925129645,-0.0161991991033988,
-0.0137468936382325));
#15989=CARTESIAN_POINT('Ctrl Pts',(0.00229094624963296,-0.01622938382382,
-0.0133274201072613));
#15990=CARTESIAN_POINT('Ctrl Pts',(0.00242300216787857,-0.0162600418379914,
-0.0128591297638758));
#15991=CARTESIAN_POINT('Ctrl Pts',(0.0024851695147177,-0.0162744745678965,
-0.0126386749097094));
#15992=CARTESIAN_POINT('Ctrl Pts',(0.00251750068801699,-0.0162890121891569,
-0.0124080172334331));
#15993=CARTESIAN_POINT('Ctrl Pts',(0.00251749999998895,-0.016303656107967,
-0.0121758458260761));
#15994=CARTESIAN_POINT('',(0.00251749991915687,-0.0173037452241442,-0.0121754098665498));
#15995=CARTESIAN_POINT('Ctrl Pts',(0.0025174992945757,-0.0163037743898821,
-0.0121739686617036));
#15996=CARTESIAN_POINT('Ctrl Pts',(0.00251713383351018,-0.0163346391685405,
-0.0116857823935164));
#15997=CARTESIAN_POINT('Ctrl Pts',(0.00237048180168344,-0.0163655039471989,
-0.0111977245059383));
#15998=CARTESIAN_POINT('Ctrl Pts',(0.00210192047764992,-0.0163963687258573,
-0.0107903077060607));
#15999=CARTESIAN_POINT('Ctrl Pts',(0.00200795198867354,-0.0164071681833874,
-0.0106477542642877));
#16000=CARTESIAN_POINT('Ctrl Pts',(0.00189951237851906,-0.0164179676409175,
-0.0105149261596554));
#16001=CARTESIAN_POINT('Ctrl Pts',(0.00177897624077857,-0.0164287670984476,
-0.0103945476460951));
#16002=CARTESIAN_POINT('Ctrl Pts',(0.00144083133054195,-0.016459063254153,
-0.0100568449253566));
#16003=CARTESIAN_POINT('Ctrl Pts',(0.00100215184109577,-0.0164893594098584,
-0.00981717015499711));
#16004=CARTESIAN_POINT('Ctrl Pts',(0.000533578279319637,-0.0165196555655639,
-0.00971554833191562));
#16005=CARTESIAN_POINT('Ctrl Pts',(0.000357754586890734,-0.016531023646047,
-0.00967741659418416));
#16006=CARTESIAN_POINT('Ctrl Pts',(0.000177989795265128,-0.0165423917265301,
-0.00965825322864707));
#16007=CARTESIAN_POINT('Ctrl Pts',(-1.40964375676471E-6,-0.0165537598070132,
-0.00965835368121463));
#16008=CARTESIAN_POINT('Ctrl Pts',(-0.000481280900188044,-0.0165841680128269,
-0.00965862237937818));
#16009=CARTESIAN_POINT('Ctrl Pts',(-0.000962613902861325,-0.0166145762186406,
-0.00980041594245372));
#16010=CARTESIAN_POINT('Ctrl Pts',(-0.00136670275312918,-0.0166449844244543,
-0.0100616324289869));
#16011=CARTESIAN_POINT('Ctrl Pts',(-0.00151628199501565,-0.0166562404548291,
-0.0101583254310283));
#16012=CARTESIAN_POINT('Ctrl Pts',(-0.00165542006449945,-0.0166674964852039,
-0.0102708741266331));
#16013=CARTESIAN_POINT('Ctrl Pts',(-0.00178096996615074,-0.0166787525155787,
-0.010396540995343));
#16014=CARTESIAN_POINT('Ctrl Pts',(-0.00212007971698423,-0.0167091550057883,
-0.0107359666737049));
#16015=CARTESIAN_POINT('Ctrl Pts',(-0.00236018527371475,-0.0167395574959981,
-0.0111764742764784));
#16016=CARTESIAN_POINT('Ctrl Pts',(-0.00246128192528678,-0.0167699599862077,
-0.0116467998542314));
#16017=CARTESIAN_POINT('Ctrl Pts',(-0.002498730331699,-0.0167812217321866,
-0.0118210187141826));
#16018=CARTESIAN_POINT('Ctrl Pts',(-0.00251756580689056,-0.0167924834781653,
-0.0119990707375693));
#16019=CARTESIAN_POINT('Ctrl Pts',(-0.00251749982649569,-0.0168037452241442,
-0.012176787949167));
#16020=CARTESIAN_POINT('Ctrl Pts',(-0.00251732170417675,-0.016834147714354,
-0.0126565577642434));
#16021=CARTESIAN_POINT('Ctrl Pts',(-0.00237567666252507,-0.0168645502045637,
-0.0131378331996337));
#16022=CARTESIAN_POINT('Ctrl Pts',(-0.00211462726198308,-0.0168949526947735,
-0.0135419271472545));
#16023=CARTESIAN_POINT('Ctrl Pts',(-0.00201792886601202,-0.0169062144407522,
-0.0136916123657435));
#16024=CARTESIAN_POINT('Ctrl Pts',(-0.00190535525634474,-0.016917476186731,
-0.0138308501418363));
#16025=CARTESIAN_POINT('Ctrl Pts',(-0.00177964827831328,-0.0169287379327098,
-0.0139564875149993));
#16026=CARTESIAN_POINT('Ctrl Pts',(-0.0014402227871498,-0.0169591461385235,
-0.0142957250637988));
#16027=CARTESIAN_POINT('Ctrl Pts',(-0.000999665739556573,-0.0169895543443372,
-0.0145359357992138));
#16028=CARTESIAN_POINT('Ctrl Pts',(-0.000529259072253469,-0.0170199625501508,
-0.0146370910004812));
#16029=CARTESIAN_POINT('Ctrl Pts',(-0.000355131346068953,-0.0170312185805257,
-0.014674535038614));
#16030=CARTESIAN_POINT('Ctrl Pts',(-0.000177171522077231,-0.0170424746109005,
-0.0146933856790558));
#16031=CARTESIAN_POINT('Ctrl Pts',(4.59681427768803E-7,-0.0170537306412753,
-0.0146933532445905));
#16032=CARTESIAN_POINT('Ctrl Pts',(0.000478562744435762,-0.0170840267969807,
-0.0146932659456422));
#16033=CARTESIAN_POINT('Ctrl Pts',(0.000958329964371957,-0.017114322952686,
-0.014552659577419));
#16034=CARTESIAN_POINT('Ctrl Pts',(0.00136154500052124,-0.0171446191083914,
-0.0142933993808747));
#16035=CARTESIAN_POINT('Ctrl Pts',(0.00151284409693271,-0.0171559871888745,
-0.0141961167154086));
#16036=CARTESIAN_POINT('Ctrl Pts',(0.00165350983650716,-0.0171673552693577,
-0.0140826484617815));
#16037=CARTESIAN_POINT('Ctrl Pts',(0.00178029842734652,-0.0171787233498408,
-0.0139558374886193));
#16038=CARTESIAN_POINT('Ctrl Pts',(0.00212453436044685,-0.0172095881284993,
-0.0136115407866458));
#16039=CARTESIAN_POINT('Ctrl Pts',(0.00236664363537164,-0.0172404529071577,
-0.0131635469362518));
#16040=CARTESIAN_POINT('Ctrl Pts',(0.00246546840766923,-0.0172713176858162,
-0.0126850406595211));
#16041=CARTESIAN_POINT('Ctrl Pts',(0.00250004678398457,-0.0172821171433462,
-0.0125176133058185));
#16042=CARTESIAN_POINT('Ctrl Pts',(0.00251749896185189,-0.0172929166008763,
-0.0123466829765938));
#16043=CARTESIAN_POINT('Ctrl Pts',(0.00251749999995351,-0.0173037160584063,
-0.0121758685863278));
#16044=CARTESIAN_POINT('',(0.00251749947371737,-0.018303848443002,-0.0121770002512912));
#16045=CARTESIAN_POINT('Ctrl Pts',(0.00251749983836023,-0.0173037743898821,
-0.0121749511467718));
#16046=CARTESIAN_POINT('Ctrl Pts',(0.00251732489744756,-0.0173346436410567,
-0.0116867632560798));
#16047=CARTESIAN_POINT('Ctrl Pts',(0.00237086248730374,-0.0173655128922312,
-0.0111986469117092));
#16048=CARTESIAN_POINT('Ctrl Pts',(0.00210245874673254,-0.0173963821434057,
-0.0107911246242246));
#16049=CARTESIAN_POINT('Ctrl Pts',(0.00200857675749333,-0.0174071795588979,
-0.0106485818901817));
#16050=CARTESIAN_POINT('Ctrl Pts',(0.00190022947733341,-0.01741797697439,
-0.0105157523906493));
#16051=CARTESIAN_POINT('Ctrl Pts',(0.00177978797063945,-0.0174287743898821,
-0.0103953586840481));
#16052=CARTESIAN_POINT('Ctrl Pts',(0.00144179465482541,-0.0174590750259716,
-0.0100574995089659));
#16053=CARTESIAN_POINT('Ctrl Pts',(0.0010032212774398,-0.0174893756620611,
-0.00981762428598563));
#16054=CARTESIAN_POINT('Ctrl Pts',(0.000534691162055855,-0.0175196762981507,
-0.00971578995175971));
#16055=CARTESIAN_POINT('Ctrl Pts',(0.000358941464853777,-0.0175310423287278,
-0.0096775910125297));
#16056=CARTESIAN_POINT('Ctrl Pts',(0.000179244643635947,-0.0175424083593049,
-0.00965834636490786));
#16057=CARTESIAN_POINT('Ctrl Pts',(-9.71885758251945E-8,-0.0175537743898821,
-0.00965835328843409));
#16058=CARTESIAN_POINT('Ctrl Pts',(-0.000479971656978348,-0.0175841870817443,
-0.00965837181408103));
#16059=CARTESIAN_POINT('Ctrl Pts',(-0.000961380981430865,-0.0176145997736064,
-0.00979991618612311));
#16060=CARTESIAN_POINT('Ctrl Pts',(-0.00136560720305024,-0.0176450124654686,
-0.0100609246312656));
#16061=CARTESIAN_POINT('Ctrl Pts',(-0.0015151879022545,-0.0176562664402731,
-0.0101575087310457));
#16062=CARTESIAN_POINT('Ctrl Pts',(-0.00165434246006101,-0.0176675204150776,
-0.0102699435837089));
#16063=CARTESIAN_POINT('Ctrl Pts',(-0.00177992543801329,-0.0176787743898821,
-0.0103954961074749));
#16064=CARTESIAN_POINT('Ctrl Pts',(-0.00211923648598154,-0.0177091813610098,
-0.0107347248716651));
#16065=CARTESIAN_POINT('Ctrl Pts',(-0.0023596010059073,-0.0177395883321375,
-0.011175094395759));
#16066=CARTESIAN_POINT('Ctrl Pts',(-0.00246097268831098,-0.0177699953032652,
-0.0116453632514138));
#16067=CARTESIAN_POINT('Ctrl Pts',(-0.00249851060273674,-0.0177812549988042,
-0.0118195037178842));
#16068=CARTESIAN_POINT('Ctrl Pts',(-0.00251744995374564,-0.0177925146943431,
-0.0119974857147075));
#16069=CARTESIAN_POINT('Ctrl Pts',(-0.00251749990051083,-0.0178037743898821,
-0.0121751455239136));
#16070=CARTESIAN_POINT('Ctrl Pts',(-0.0025176347824747,-0.0178341813610099,
-0.0126549184156753));
#16071=CARTESIAN_POINT('Ctrl Pts',(-0.00237630203724782,-0.0178645883321375,
-0.0131362885610932));
#16072=CARTESIAN_POINT('Ctrl Pts',(-0.00211551373521293,-0.0178949953032653,
-0.013540553944624));
#16073=CARTESIAN_POINT('Ctrl Pts',(-0.00201894387731103,-0.0179062549988042,
-0.0136902533381075));
#16074=CARTESIAN_POINT('Ctrl Pts',(-0.00190650237038634,-0.0179175146943432,
-0.0138295224041051));
#16075=CARTESIAN_POINT('Ctrl Pts',(-0.00178092620551187,-0.0179287743898821,
-0.0139552093781039));
#16076=CARTESIAN_POINT('Ctrl Pts',(-0.00144174214903808,-0.0179591870817443,
-0.0142946927325241));
#16077=CARTESIAN_POINT('Ctrl Pts',(-0.00100135469175334,-0.0179895997736064,
-0.014535220201561));
#16078=CARTESIAN_POINT('Ctrl Pts',(-0.000531018002186749,-0.0180200124654686,
-0.0146367121064325));
#16079=CARTESIAN_POINT('Ctrl Pts',(-0.000356973649979874,-0.0180312664402731,
-0.0146742683788421));
#16080=CARTESIAN_POINT('Ctrl Pts',(-0.000179086413295556,-0.0180425204150776,
-0.0146932461316884));
#16081=CARTESIAN_POINT('Ctrl Pts',(-1.5127137924576E-6,-0.0180537743898821,
-0.0146933528320788));
#16082=CARTESIAN_POINT('Ctrl Pts',(0.000476593567870745,-0.0180840750259716,
-0.0146936401163279));
#16083=CARTESIAN_POINT('Ctrl Pts',(0.00095647340039854,-0.0181143756620611,
-0.014553407831921));
#16084=CARTESIAN_POINT('Ctrl Pts',(0.00135989276293095,-0.0181446762981507,
-0.014294460830047));
#16085=CARTESIAN_POINT('Ctrl Pts',(0.00151121885378951,-0.0181560423287278,
-0.0141973275707826));
#16086=CARTESIAN_POINT('Ctrl Pts',(0.00165193110895003,-0.0181674083593049,
-0.0140840109266131));
#16087=CARTESIAN_POINT('Ctrl Pts',(0.00177878656316556,-0.0181787743898821,
-0.0139573483364254));
#16088=CARTESIAN_POINT('Ctrl Pts',(0.00212331606732685,-0.0182096436410565,
-0.0136133426358977));
#16089=CARTESIAN_POINT('Ctrl Pts',(0.00236580582515884,-0.0182405128922309,
-0.0131655527105787));
#16090=CARTESIAN_POINT('Ctrl Pts',(0.00246503618344002,-0.0182713821434054,
-0.0126871290089735));
#16091=CARTESIAN_POINT('Ctrl Pts',(0.00249974487791892,-0.0182821795588976,
-0.012519786449921));
#16092=CARTESIAN_POINT('Ctrl Pts',(0.00251734172976889,-0.0182929769743899,
-0.0123489287571923));
#16093=CARTESIAN_POINT('Ctrl Pts',(0.00251749893315368,-0.0183037743898821,
-0.0121781709513438));
#16094=CARTESIAN_POINT('',(0.00251749999999994,-0.0193037658457995,-0.0121758527464904));
#16095=CARTESIAN_POINT('Ctrl Pts',(0.00251749999998966,-0.0183039205383097,
-0.0121758605021413));
#16096=CARTESIAN_POINT('Ctrl Pts',(0.00251750139920864,-0.0183347784818584,
-0.0116876762924853));
#16097=CARTESIAN_POINT('Ctrl Pts',(0.00237121741640988,-0.0183656364254071,
-0.0111995101627397));
#16098=CARTESIAN_POINT('Ctrl Pts',(0.00210296441023168,-0.0183964943689557,
-0.0107918926876612));
#16099=CARTESIAN_POINT('Ctrl Pts',(0.00200905844461261,-0.0184072966523197,
-0.0106492001111798));
#16100=CARTESIAN_POINT('Ctrl Pts',(0.0019006601175944,-0.0184180989356836,
-0.0105162313326969));
#16101=CARTESIAN_POINT('Ctrl Pts',(0.00178014554476341,-0.0184289012190475,
-0.0103957161880573));
#16102=CARTESIAN_POINT('Ctrl Pts',(0.00144222588007803,-0.0184591905349901,
-0.0100577949200357));
#16103=CARTESIAN_POINT('Ctrl Pts',(0.00100370846356905,-0.0184894798509328,
-0.00981783290983037));
#16104=CARTESIAN_POINT('Ctrl Pts',(0.000535205959966458,-0.0185197691668754,
-0.0097159018987424));
#16105=CARTESIAN_POINT('Ctrl Pts',(0.000359325452537379,-0.0185311400778453,
-0.00967763598166606));
#16106=CARTESIAN_POINT('Ctrl Pts',(0.000179487594139983,-0.0185425109888153,
-0.0096583536237291));
#16107=CARTESIAN_POINT('Ctrl Pts',(4.72923594120771E-9,-0.0185538818997853,
-0.00965835328656254));
#16108=CARTESIAN_POINT('Ctrl Pts',(-0.00047986206250833,-0.0185842832563119,
-0.00965835238511138));
#16109=CARTESIAN_POINT('Ctrl Pts',(-0.000961271083096095,-0.0186146846128386,
-0.00979987295396124));
#16110=CARTESIAN_POINT('Ctrl Pts',(-0.00136550482274316,-0.0186450859693652,
-0.0100608585279203));
#16111=CARTESIAN_POINT('Ctrl Pts',(-0.00151520917150609,-0.0186563448397512,
-0.0101575122001749));
#16112=CARTESIAN_POINT('Ctrl Pts',(-0.00165447146738626,-0.0186676037101371,
-0.0102700424587043));
#16113=CARTESIAN_POINT('Ctrl Pts',(-0.00178013885661713,-0.0186788625805231,
-0.0103957094999044));
#16114=CARTESIAN_POINT('Ctrl Pts',(-0.00211940395598334,-0.0187092582289377,
-0.0107349736596895));
#16115=CARTESIAN_POINT('Ctrl Pts',(-0.00235971449685064,-0.0187396538773524,
-0.0111753648807987));
#16116=CARTESIAN_POINT('Ctrl Pts',(-0.00246103217853601,-0.0187700495257671,
-0.0116456393050277));
#16117=CARTESIAN_POINT('Ctrl Pts',(-0.00249858034868863,-0.018781314104265,
-0.0118199222515544));
#16118=CARTESIAN_POINT('Ctrl Pts',(-0.00251749984159334,-0.018792578682763,
-0.0119980507507866));
#16119=CARTESIAN_POINT('Ctrl Pts',(-0.002517499999999,-0.0188038432612609,
-0.0121758510436694));
#16120=CARTESIAN_POINT('Ctrl Pts',(-0.00251750042743114,-0.0188342389096755,
-0.0126556164597899));
#16121=CARTESIAN_POINT('Ctrl Pts',(-0.00237603699480804,-0.0188646345580901,
-0.0131369410996882));
#16122=CARTESIAN_POINT('Ctrl Pts',(-0.00211514174614456,-0.0188950302065047,
-0.0135411304172962));
#16123=CARTESIAN_POINT('Ctrl Pts',(-0.00201845438589362,-0.0189062947850027,
-0.0136909223294194));
#16124=CARTESIAN_POINT('Ctrl Pts',(-0.00190587290559756,-0.0189175593635007,
-0.0138302629243774));
#16125=CARTESIAN_POINT('Ctrl Pts',(-0.00178014202854226,-0.0189288239419987,
-0.0139559939012898));
#16126=CARTESIAN_POINT('Ctrl Pts',(-0.00144081382194874,-0.0189592252985253,
-0.0142953223773822));
#16127=CARTESIAN_POINT('Ctrl Pts',(-0.00100032772075606,-0.0189896266550519,
-0.0145356545566116));
#16128=CARTESIAN_POINT('Ctrl Pts',(-0.000529953127711334,-0.0190200280115784,
-0.0146369416499512));
#16129=CARTESIAN_POINT('Ctrl Pts',(-0.000355754105659654,-0.0190312868819645,
-0.0146744524187451));
#16130=CARTESIAN_POINT('Ctrl Pts',(-0.000177714129453871,-0.0190425457523505,
-0.0146933533037442));
#16131=CARTESIAN_POINT('Ctrl Pts',(2.43458683768248E-10,-0.0190538046227365,
-0.0146933532865581));
#16132=CARTESIAN_POINT('Ctrl Pts',(0.000478098543211599,-0.0190840939386791,
-0.0146933532403229));
#16133=CARTESIAN_POINT('Ctrl Pts',(0.00095788765689851,-0.0191143832546218,
-0.0145528371021288));
#16134=CARTESIAN_POINT('Ctrl Pts',(0.00136114808352063,-0.0191446725705644,
-0.0142936545389725));
#16135=CARTESIAN_POINT('Ctrl Pts',(0.00151253606525985,-0.0191560434815344,
-0.014196354822591));
#16136=CARTESIAN_POINT('Ctrl Pts',(0.00165328373806845,-0.0191674143925042,
-0.0140828523415883));
#16137=CARTESIAN_POINT('Ctrl Pts',(0.00178014237284466,-0.0191787853034742,
-0.0139559935569871));
#16138=CARTESIAN_POINT('Ctrl Pts',(0.00212440648315945,-0.0192096432466914,
-0.0136117290400828));
#16139=CARTESIAN_POINT('Ctrl Pts',(0.00236655471500398,-0.0192405011899086,
-0.0131637590122813));
#16140=CARTESIAN_POINT('Ctrl Pts',(0.00246542235843722,-0.0192713591331258,
-0.0126852635775003));
#16141=CARTESIAN_POINT('Ctrl Pts',(0.00250003230517401,-0.0192821613706837,
-0.0125177598226167));
#16142=CARTESIAN_POINT('Ctrl Pts',(0.00251750003666136,-0.0192929636082416,
-0.0123467481863637));
#16143=CARTESIAN_POINT('Ctrl Pts',(0.00251749999999994,-0.0193037658457995,
-0.0121758527464904));
#16144=CARTESIAN_POINT('',(0.00251749947628337,-0.0203037041496287,-0.012174691451596));
#16145=CARTESIAN_POINT('Ctrl Pts',(0.0025174999963034,-0.0193037743898821,
-0.0121757168592769));
#16146=CARTESIAN_POINT('Ctrl Pts',(0.00251747354082491,-0.0193346329618525,
-0.0116875324843154));
#16147=CARTESIAN_POINT('Ctrl Pts',(0.00237116161052997,-0.0193654915338229,
-0.011199374563954));
#16148=CARTESIAN_POINT('Ctrl Pts',(0.0021028851898957,-0.0193963501057933,
-0.0107917723177859));
#16149=CARTESIAN_POINT('Ctrl Pts',(0.0020089744578595,-0.0194071522145902,
-0.0106490902839838));
#16150=CARTESIAN_POINT('Ctrl Pts',(0.00190057297331317,-0.0194179543233872,
-0.0105161321686755));
#16151=CARTESIAN_POINT('Ctrl Pts',(0.00178005673749341,-0.0194287564321841,
-0.0103956273847961));
#16152=CARTESIAN_POINT('Ctrl Pts',(0.00144211995671279,-0.0194590463748431,
-0.0100577227161358));
#16153=CARTESIAN_POINT('Ctrl Pts',(0.00100359022221706,-0.0194893363175022,
-0.00981778252450338));
#16154=CARTESIAN_POINT('Ctrl Pts',(0.00053508231450667,-0.0195196262601613,
-0.00971587500073885));
#16155=CARTESIAN_POINT('Ctrl Pts',(0.000359206091161296,-0.0195309969982695,
-0.0096776192741754));
#16156=CARTESIAN_POINT('Ctrl Pts',(0.000179373751020931,-0.0195423677363778,
-0.00965834595937489));
#16157=CARTESIAN_POINT('Ctrl Pts',(-1.02807121700726E-7,-0.019553738474486,
-0.00965835328865726));
#16158=CARTESIAN_POINT('Ctrl Pts',(-0.000479969941798783,-0.0195841404588545,
-0.00965837288498654));
#16159=CARTESIAN_POINT('Ctrl Pts',(-0.000961373186645005,-0.0196145424432232,
-0.0097999142102839));
#16160=CARTESIAN_POINT('Ctrl Pts',(-0.00136559591408811,-0.0196449444275917,
-0.0100609173420373));
#16161=CARTESIAN_POINT('Ctrl Pts',(-0.00151529077974533,-0.0196562031239905,
-0.0101575740268089));
#16162=CARTESIAN_POINT('Ctrl Pts',(-0.00165454365490057,-0.0196674618203892,
-0.010270105715057));
#16163=CARTESIAN_POINT('Ctrl Pts',(-0.00178020212969005,-0.019678720516788,
-0.0103957727750511));
#16164=CARTESIAN_POINT('Ctrl Pts',(-0.00211945540596841,-0.0197091167924575,
-0.0107350492297008));
#16165=CARTESIAN_POINT('Ctrl Pts',(-0.00235975034622185,-0.0197395130681269,
-0.0111754493104245));
#16166=CARTESIAN_POINT('Ctrl Pts',(-0.00246105120592157,-0.0197699093437964,
-0.0116457276299143));
#16167=CARTESIAN_POINT('Ctrl Pts',(-0.00249859178927552,-0.0197811737488942,
-0.0118200057407289));
#16168=CARTESIAN_POINT('Ctrl Pts',(-0.00251750488525685,-0.0197924381539921,
-0.0119981284624587));
#16169=CARTESIAN_POINT('Ctrl Pts',(-0.00251749999904929,-0.01980370255909,
-0.0121759224735203));
#16170=CARTESIAN_POINT('Ctrl Pts',(-0.00251748681393115,-0.0198340988347594,
-0.0126556882246331));
#16171=CARTESIAN_POINT('Ctrl Pts',(-0.00237600953633413,-0.019864495110429,
-0.0131370091134419));
#16172=CARTESIAN_POINT('Ctrl Pts',(-0.00211510253618663,-0.0198948913860984,
-0.0135411911610115));
#16173=CARTESIAN_POINT('Ctrl Pts',(-0.00201841430455986,-0.0199061557911963,
-0.0136909749821151));
#16174=CARTESIAN_POINT('Ctrl Pts',(-0.00190583338544541,-0.0199174201962941,
-0.0138303077751249));
#16175=CARTESIAN_POINT('Ctrl Pts',(-0.00178010428520308,-0.0199286846013919,
-0.0139560316438587));
#16176=CARTESIAN_POINT('Ctrl Pts',(-0.00144076864279242,-0.0199590865857605,
-0.0142953531667276));
#16177=CARTESIAN_POINT('Ctrl Pts',(-0.00100027711999404,-0.0199894885701291,
-0.0145356760614747));
#16178=CARTESIAN_POINT('Ctrl Pts',(-0.00052990007681995,-0.0200198905544978,
-0.0146369530729516));
#16179=CARTESIAN_POINT('Ctrl Pts',(-0.000355706436766571,-0.0200311492508965,
-0.0146744587538493));
#16180=CARTESIAN_POINT('Ctrl Pts',(-0.00017767251696946,-0.0200424079472952,
-0.0146933557969358));
#16181=CARTESIAN_POINT('Ctrl Pts',(3.55668027982208E-8,-0.0200536666436939,
-0.0146933532863069));
#16182=CARTESIAN_POINT('Ctrl Pts',(0.00047813422732945,-0.0200839565863528,
-0.014693346531812));
#16183=CARTESIAN_POINT('Ctrl Pts',(0.000957921653604442,-0.0201142465290118,
-0.0145528234596369));
#16184=CARTESIAN_POINT('Ctrl Pts',(0.00136117858854318,-0.0201445364716708,
-0.014293634932548));
#16185=CARTESIAN_POINT('Ctrl Pts',(0.0015125598258468,-0.0201559072097791,
-0.0141963364696422));
#16186=CARTESIAN_POINT('Ctrl Pts',(0.00165330127616514,-0.0201672779478875,
-0.0140828365438326));
#16187=CARTESIAN_POINT('Ctrl Pts',(0.00178015458459382,-0.0201786486859959,
-0.0139559813451397));
#16188=CARTESIAN_POINT('Ctrl Pts',(0.00212441648830734,-0.0202095072579661,
-0.0136117143115169));
#16189=CARTESIAN_POINT('Ctrl Pts',(0.00236656167233786,-0.0202403658299364,
-0.0131637424207738));
#16190=CARTESIAN_POINT('Ctrl Pts',(0.00246542596178269,-0.0202712244019067,
-0.0126852461378702));
#16191=CARTESIAN_POINT('Ctrl Pts',(0.00250003361672395,-0.0202820265107037,
-0.0125177474956164));
#16192=CARTESIAN_POINT('Ctrl Pts',(0.00251750013213901,-0.0202928286195008,
-0.0123467413196633));
#16193=CARTESIAN_POINT('Ctrl Pts',(0.00251749999999925,-0.0203036307282978,
-0.0121758513399147));
#16194=CARTESIAN_POINT('',(0.00251749986350914,-0.0213038121901123,-0.01217643077317));
#16195=CARTESIAN_POINT('Ctrl Pts',(0.00251749897525818,-0.0203037743898821,
-0.0121735818169921));
#16196=CARTESIAN_POINT('Ctrl Pts',(0.00251705849677081,-0.0203346440943988,
-0.0116853938363173));
#16197=CARTESIAN_POINT('Ctrl Pts',(0.00237033046382402,-0.0203655137989155,
-0.0111973570147749));
#16198=CARTESIAN_POINT('Ctrl Pts',(0.0021017048578511,-0.0203963835034322,
-0.0107899806587582));
#16199=CARTESIAN_POINT('Ctrl Pts',(0.00200775058956061,-0.0204071804655822,
-0.0106474970436546));
#16200=CARTESIAN_POINT('Ctrl Pts',(0.00189933794761061,-0.0204179774277321,
-0.0105147334340231));
#16201=CARTESIAN_POINT('Ctrl Pts',(0.00177883905851618,-0.0204287743898821,
-0.010394410653775));
#16202=CARTESIAN_POINT('Ctrl Pts',(0.00144066537566995,-0.020459075486276,
-0.0100567312109801));
#16203=CARTESIAN_POINT('Ctrl Pts',(0.00100196371446668,-0.02048937658267,
-0.00981708960752238));
#16204=CARTESIAN_POINT('Ctrl Pts',(0.000533378912095895,-0.0205196776790639,
-0.00971550510263546));
#16205=CARTESIAN_POINT('Ctrl Pts',(0.000357618489739118,-0.0205310432493366,
-0.00967740199857939));
#16206=CARTESIAN_POINT('Ctrl Pts',(0.00017792148625705,-0.0205424088196094,
-0.00965825320302302));
#16207=CARTESIAN_POINT('Ctrl Pts',(-1.41054041913628E-6,-0.0205537743898821,
-0.00965835368171687));
#16208=CARTESIAN_POINT('Ctrl Pts',(-0.000481285466023079,-0.0205841875419004,
-0.0096586225528529));
#16209=CARTESIAN_POINT('Ctrl Pts',(-0.000962621300933848,-0.0206146006939189,
-0.00980041835081507));
#16210=CARTESIAN_POINT('Ctrl Pts',(-0.00136671151339475,-0.0206450138459373,
-0.01006163809194));
#16211=CARTESIAN_POINT('Ctrl Pts',(-0.00151623350711667,-0.0206562673605856,
-0.0101582949653016));
#16212=CARTESIAN_POINT('Ctrl Pts',(-0.00165532223979631,-0.0206675208752338,
-0.0102707953898936));
#16213=CARTESIAN_POINT('Ctrl Pts',(-0.00178083420496772,-0.0206787743898821,
-0.0103964051180471));
#16214=CARTESIAN_POINT('Ctrl Pts',(-0.00211997237410261,-0.0207091818203525,
-0.0107358074465291));
#16215=CARTESIAN_POINT('Ctrl Pts',(-0.00236011210471939,-0.0207395892508229,
-0.0111763001296675));
#16216=CARTESIAN_POINT('Ctrl Pts',(-0.0024612435032972,-0.0207699966812933,
-0.0116466211376127));
#16217=CARTESIAN_POINT('Ctrl Pts',(-0.00249869034723741,-0.0207812559174896,
-0.011820771180369));
#16218=CARTESIAN_POINT('Ctrl Pts',(-0.00251753872390049,-0.0207925151536858,
-0.0119987528246532));
#16219=CARTESIAN_POINT('Ctrl Pts',(-0.00251749994000549,-0.0208037743898821,
-0.0121764028976655));
#16220=CARTESIAN_POINT('Ctrl Pts',(-0.00251739519767926,-0.0208341818203525,
-0.0126561763164846));
#16221=CARTESIAN_POINT('Ctrl Pts',(-0.00237582175629021,-0.0208645892508229,
-0.0131374762202163));
#16222=CARTESIAN_POINT('Ctrl Pts',(-0.00211483113574972,-0.0208949966812933,
-0.0135416115072046));
#16223=CARTESIAN_POINT('Ctrl Pts',(-0.00201819176187889,-0.0209062559174896,
-0.0136912543603186));
#16224=CARTESIAN_POINT('Ctrl Pts',(-0.0019056877099657,-0.0209175151536858,
-0.0138304601068289));
#16225=CARTESIAN_POINT('Ctrl Pts',(-0.00178005707040119,-0.0209287743898821,
-0.0139560788554439));
#16226=CARTESIAN_POINT('Ctrl Pts',(-0.00144070689844957,-0.0209591875419005,
-0.0142953969078761));
#16227=CARTESIAN_POINT('Ctrl Pts',(-0.00100020153004592,-0.020989600693919,
-0.0145357093764282));
#16228=CARTESIAN_POINT('Ctrl Pts',(-0.000529814865194679,-0.0210200138459375,
-0.0146369714183467));
#16229=CARTESIAN_POINT('Ctrl Pts',(-0.000355761770664609,-0.0210312673605856,
-0.0146744405327399));
#16230=CARTESIAN_POINT('Ctrl Pts',(-0.000177875298078815,-0.0210425208752339,
-0.0146933313094496));
#16231=CARTESIAN_POINT('Ctrl Pts',(-3.11318268668838E-7,-0.0210537743898821,
-0.014693353267309));
#16232=CARTESIAN_POINT('Ctrl Pts',(0.000477795605346852,-0.021084075486276,
-0.0146934123908128));
#16233=CARTESIAN_POINT('Ctrl Pts',(0.000957608902555014,-0.02111437658267,
-0.0145529508021383));
#16234=CARTESIAN_POINT('Ctrl Pts',(0.0013609048698769,-0.0211446776790639,
-0.0142938108369224));
#16235=CARTESIAN_POINT('Ctrl Pts',(0.00151217624955624,-0.0211560432493366,
-0.0141966106086916));
#16236=CARTESIAN_POINT('Ctrl Pts',(0.00165282723223209,-0.0211674088196094,
-0.0140832338478495));
#16237=CARTESIAN_POINT('Ctrl Pts',(0.00177961672460848,-0.0211787743898821,
-0.0139565190506738));
#16238=CARTESIAN_POINT('Ctrl Pts',(0.00212398608501294,-0.0212096440943986,
-0.0136123525677949));
#16239=CARTESIAN_POINT('Ctrl Pts',(0.00236626713873879,-0.021240513798915,
-0.0131644493631118));
#16240=CARTESIAN_POINT('Ctrl Pts',(0.00246527438524578,-0.0212713835034315,
-0.0126859792077296));
#16241=CARTESIAN_POINT('Ctrl Pts',(0.00249990307735264,-0.0212821804655817,
-0.0125186298845476));
#16242=CARTESIAN_POINT('Ctrl Pts',(0.0025174202199173,-0.0212929774277319,
-0.0123477738068224));
#16243=CARTESIAN_POINT('Ctrl Pts',(0.00251749972707755,-0.0213037743898821,
-0.0121770255341664));
#16244=CARTESIAN_POINT('',(0.00251780046414957,-0.0223033403968196,-0.0121761624005998));
#16245=CARTESIAN_POINT('Ctrl Pts',(0.00251749999994073,-0.0213038499903425,
-0.0121758360121736));
#16246=CARTESIAN_POINT('Ctrl Pts',(0.00251749665014283,-0.0213347138852245,
-0.0116876498063799));
#16247=CARTESIAN_POINT('Ctrl Pts',(0.00237120678745751,-0.0213655777801066,
-0.0111994834398425));
#16248=CARTESIAN_POINT('Ctrl Pts',(0.00210294792643045,-0.0213964416749887,
-0.010791867640418));
#16249=CARTESIAN_POINT('Ctrl Pts',(0.00200908115279786,-0.0214072412967541,
-0.010649238316536));
#16250=CARTESIAN_POINT('Ctrl Pts',(0.0019007347840987,-0.0214180409185194,
-0.0105163244402839));
#16251=CARTESIAN_POINT('Ctrl Pts',(0.00178028171630679,-0.0214288405402849,
-0.010395852370664));
#16252=CARTESIAN_POINT('Ctrl Pts',(0.00144238479207546,-0.0214591358166468,
-0.0100579021421928));
#16253=CARTESIAN_POINT('Ctrl Pts',(0.00100388155370561,-0.0214894310930088,
-0.00981790589049112));
#16254=CARTESIAN_POINT('Ctrl Pts',(0.000535383004862202,-0.0215197263693707,
-0.00971594042466548));
#16255=CARTESIAN_POINT('Ctrl Pts',(0.000359579885819401,-0.0215310946096563,
-0.00967767809285879));
#16256=CARTESIAN_POINT('Ctrl Pts',(0.000179821417535125,-0.0215424628499418,
-0.00965838285146188));
#16257=CARTESIAN_POINT('Ctrl Pts',(4.14386135004118E-7,-0.0215538310902274,
-0.00965835332066254));
#16258=CARTESIAN_POINT('Ctrl Pts',(-0.000479456527140519,-0.0215842384148768,
-0.00965827433283503));
#16259=CARTESIAN_POINT('Ctrl Pts',(-0.000960891814846311,-0.0216146457395262,
-0.00979971888222035));
#16260=CARTESIAN_POINT('Ctrl Pts',(-0.00136516965727927,-0.0216450530641756,
-0.0100606421725451));
#16261=CARTESIAN_POINT('Ctrl Pts',(-0.00151482534279141,-0.0216563092561736,
-0.0101572308296049));
#16262=CARTESIAN_POINT('Ctrl Pts',(-0.00165405045888319,-0.0216675654481718,
-0.0102696841045556));
#16263=CARTESIAN_POINT('Ctrl Pts',(-0.00177969563557523,-0.0216788216401698,
-0.0103952663904156));
#16264=CARTESIAN_POINT('Ctrl Pts',(-0.00211904802334732,-0.0217092232499438,
-0.0107344489176758));
#16265=CARTESIAN_POINT('Ctrl Pts',(-0.00235946883020976,-0.0217396248597177,
-0.0111747841255715));
#16266=CARTESIAN_POINT('Ctrl Pts',(-0.00246090230640666,-0.0217700264694917,
-0.0116450368509399));
#16267=CARTESIAN_POINT('Ctrl Pts',(-0.00249847710495456,-0.0217812883763652,
-0.011819236258126));
#16268=CARTESIAN_POINT('Ctrl Pts',(-0.00251744013055233,-0.0217925502832388,
-0.0119972824892468));
#16269=CARTESIAN_POINT('Ctrl Pts',(-0.00251749985783616,-0.0218038121901123,
-0.0121750072399159));
#16270=CARTESIAN_POINT('Ctrl Pts',(-0.00251766109212767,-0.0218342137998863,
-0.0126547766588689));
#16271=CARTESIAN_POINT('Ctrl Pts',(-0.00237635673330881,-0.0218646154096603,
-0.0131361518485057));
#16272=CARTESIAN_POINT('Ctrl Pts',(-0.00211559356671986,-0.0218950170194343,
-0.0135404301845208));
#16273=CARTESIAN_POINT('Ctrl Pts',(-0.00201899702068176,-0.0219062789263078,
-0.0136901901809495));
#16274=CARTESIAN_POINT('Ctrl Pts',(-0.00190651651240216,-0.0219175408331812,
-0.0138295130796314));
#16275=CARTESIAN_POINT('Ctrl Pts',(-0.00178089202362918,-0.0219288027400547,
-0.0139552435894917));
#16276=CARTESIAN_POINT('Ctrl Pts',(-0.0014417039396801,-0.0219592100647042,
-0.0142947179320342));
#16277=CARTESIAN_POINT('Ctrl Pts',(-0.00100131523292127,-0.0219896173893536,
-0.0145352363725553));
#16278=CARTESIAN_POINT('Ctrl Pts',(-0.000530979723704272,-0.022020024714003,
-0.0146367203660679));
#16279=CARTESIAN_POINT('Ctrl Pts',(-0.000356870792507748,-0.0220312809060011,
-0.0146742877393531));
#16280=CARTESIAN_POINT('Ctrl Pts',(-0.000178916436407483,-0.0220425370979991,
-0.0146932628053001));
#16281=CARTESIAN_POINT('Ctrl Pts',(-1.27770712460287E-6,-0.0220537932899972,
-0.0146933529623206));
#16282=CARTESIAN_POINT('Ctrl Pts',(0.000476824869407315,-0.0220840885663592,
-0.014693595613819));
#16283=CARTESIAN_POINT('Ctrl Pts',(0.000956688669868174,-0.0221143838427211,
-0.0145533206203796));
#16284=CARTESIAN_POINT('Ctrl Pts',(0.00136008235768505,-0.0221446791190831,
-0.0142943391209015));
#16285=CARTESIAN_POINT('Ctrl Pts',(0.00151145501122909,-0.0221560473593686,
-0.0141971568446816));
#16286=CARTESIAN_POINT('Ctrl Pts',(0.00165220458265205,-0.0221674155996541,
-0.0140837802632861));
#16287=CARTESIAN_POINT('Ctrl Pts',(0.00177908491797799,-0.0221787838399396,
-0.0139570503853159));
#16288=CARTESIAN_POINT('Ctrl Pts',(0.00212355523473457,-0.0222096477348218,
-0.0136129885486668));
#16289=CARTESIAN_POINT('Ctrl Pts',(0.00236596974171468,-0.022240511629704,
-0.0131651600397046));
#16290=CARTESIAN_POINT('Ctrl Pts',(0.00246512068629229,-0.0222713755245862,
-0.0126867214221996));
#16291=CARTESIAN_POINT('Ctrl Pts',(0.00249981470994674,-0.0222821751463515,
-0.0125193104027319));
#16292=CARTESIAN_POINT('Ctrl Pts',(0.00251738343267912,-0.0222929747681168,
-0.0123483844243074));
#16293=CARTESIAN_POINT('Ctrl Pts',(0.00251749941967471,-0.0223037743898821,
-0.0121775626541275));
#16294=CARTESIAN_POINT('',(0.00251749967473612,-0.0233037176099892,-0.0121749448086545));
#16295=CARTESIAN_POINT('Ctrl Pts',(0.00251749999999092,-0.0223038816194607,
-0.0121758600475192));
#16296=CARTESIAN_POINT('Ctrl Pts',(0.0025175013076005,-0.0223345812349272,
-0.0116889607629736));
#16297=CARTESIAN_POINT('Ctrl Pts',(0.0023719606845788,-0.0223652878514534,
-0.0112019687080946));
#16298=CARTESIAN_POINT('Ctrl Pts',(0.0021050319083829,-0.0223960166366596,
-0.010795039427021));
#16299=CARTESIAN_POINT('Ctrl Pts',(0.00201064111538942,-0.0224068828851198,
-0.0106511419496481));
#16300=CARTESIAN_POINT('Ctrl Pts',(0.00190153428401059,-0.0224177519056763,
-0.0105171068557753));
#16301=CARTESIAN_POINT('Ctrl Pts',(0.0017801554621912,-0.0224286243690166,
-0.0103957261055874));
#16302=CARTESIAN_POINT('Ctrl Pts',(0.00144142058921467,-0.0224589664207296,
-0.0100569858510652));
#16303=CARTESIAN_POINT('Ctrl Pts',(0.00100161012373136,-0.0224893352853389,
-0.00981665712105438));
#16304=CARTESIAN_POINT('Ctrl Pts',(0.000531596077416871,-0.022519687231543,
-0.00971511927808115));
#16305=CARTESIAN_POINT('Ctrl Pts',(0.000356906568067011,-0.0225309680999166,
-0.00967738084003122));
#16306=CARTESIAN_POINT('Ctrl Pts',(0.00017830964556315,-0.0225422466312219,
-0.00965835423079078));
#16307=CARTESIAN_POINT('Ctrl Pts',(1.33318343165638E-8,-0.0225535205802314,
-0.0096583532865934));
#16308=CARTESIAN_POINT('Ctrl Pts',(-0.000487515190307265,-0.022584347755423,
-0.00965835070480611));
#16309=CARTESIAN_POINT('Ctrl Pts',(-0.00097570005348263,-0.0226151406697395,
-0.0098042645785878));
#16310=CARTESIAN_POINT('Ctrl Pts',(-0.00138377394701436,-0.022646067631192,
-0.0100727660526174));
#16311=CARTESIAN_POINT('Ctrl Pts',(-0.00152647526742239,-0.0226568826289301,
-0.0101666596230782));
#16312=CARTESIAN_POINT('Ctrl Pts',(-0.00165951649133449,-0.0226677140188173,
-0.0102750877733898));
#16313=CARTESIAN_POINT('Ctrl Pts',(-0.0017801366081372,-0.0226785689981989,
-0.0103957072514335));
#16314=CARTESIAN_POINT('Ctrl Pts',(-0.00208925477812789,-0.0227063875035252,
-0.01070482378445));
#16315=CARTESIAN_POINT('Ctrl Pts',(-0.0023182875516416,-0.0227343609362434,
-0.0111011289644275));
#16316=CARTESIAN_POINT('Ctrl Pts',(-0.00243164824112718,-0.0227620377754448,
-0.0115240150540011));
#16317=CARTESIAN_POINT('Ctrl Pts',(-0.00248901528948984,-0.0227760438526854,
-0.0117380198105225));
#16318=CARTESIAN_POINT('Ctrl Pts',(-0.00251749999999999,-0.0227899739739923,
-0.0119583162425569));
#16319=CARTESIAN_POINT('Ctrl Pts',(-0.0025175,-0.022803769622919,-0.012175853286558));
#16320=CARTESIAN_POINT('Ctrl Pts',(-0.00251750000000002,-0.02284482629222,
-0.0128232564296606));
#16321=CARTESIAN_POINT('Ctrl Pts',(-0.00226454183273898,-0.0228846919492015,
-0.0134500557724457));
#16322=CARTESIAN_POINT('Ctrl Pts',(-0.00182003347813458,-0.0229253542607035,
-0.0139151877536659));
#16323=CARTESIAN_POINT('Ctrl Pts',(-0.00150076880653732,-0.0229545596499691,
-0.014249265184822));
#16324=CARTESIAN_POINT('Ctrl Pts',(-0.00108140438732256,-0.022984176010916,
-0.0144976113812731));
#16325=CARTESIAN_POINT('Ctrl Pts',(-0.000624780936849887,-0.0230140057534222,
-0.0146145937464982));
#16326=CARTESIAN_POINT('Ctrl Pts',(-0.000445653060287442,-0.0230257076019102,
-0.0146604845185476));
#16327=CARTESIAN_POINT('Ctrl Pts',(-0.000261162728481951,-0.0230374422876512,
-0.0146866080241517));
#16328=CARTESIAN_POINT('Ctrl Pts',(-7.60742024150088E-5,-0.0230491978823017,
-0.0146922036130681));
#16329=CARTESIAN_POINT('Ctrl Pts',(0.000394806181150458,-0.0230791050787968,
-0.0147064392499884));
#16330=CARTESIAN_POINT('Ctrl Pts',(0.000875641029012556,-0.0231091476051378,
-0.0145843270790017));
#16331=CARTESIAN_POINT('Ctrl Pts',(0.00128748301215453,-0.0231393790289019,
-0.0143392288303353));
#16332=CARTESIAN_POINT('Ctrl Pts',(0.00145018545103835,-0.0231513222658196,
-0.0142424002299097));
#16333=CARTESIAN_POINT('Ctrl Pts',(0.00160218063497924,-0.0231632949844648,
-0.0141269606956049));
#16334=CARTESIAN_POINT('Ctrl Pts',(0.00173934420262757,-0.0231753004877138,
-0.0139958774607893));
#16335=CARTESIAN_POINT('Ctrl Pts',(0.00208806524676423,-0.02320582296318,
-0.0136626148948074));
#16336=CARTESIAN_POINT('Ctrl Pts',(0.00234152922365597,-0.023236557347308,
-0.0132226449996777));
#16337=CARTESIAN_POINT('Ctrl Pts',(0.00245239154138134,-0.023267485547987,
-0.0127446959517664));
#16338=CARTESIAN_POINT('Ctrl Pts',(0.00249551121723139,-0.0232795150095323,
-0.0125587986293792));
#16339=CARTESIAN_POINT('Ctrl Pts',(0.00251750054521379,-0.0232915737917502,
-0.0123675108385863));
#16340=CARTESIAN_POINT('Ctrl Pts',(0.00251749999998981,-0.0233036608300962,
-0.0121758461250867));
#16341=CARTESIAN_POINT('',(0.00251749989572715,-0.0243037413029277,-0.012175349188554));
#16342=CARTESIAN_POINT('Ctrl Pts',(0.00251749934948243,-0.0233037743898821,
-0.0121740434922223));
#16343=CARTESIAN_POINT('Ctrl Pts',(0.00251714839939817,-0.0233346387771943,
-0.0116858572981548));
#16344=CARTESIAN_POINT('Ctrl Pts',(0.00237051092282184,-0.0233655031645063,
-0.0111977951221388));
#16345=CARTESIAN_POINT('Ctrl Pts',(0.00210196178929609,-0.0233963675518184,
-0.0107903703792874));
#16346=CARTESIAN_POINT('Ctrl Pts',(0.00200799581241252,-0.0234071670739267,
-0.0106478114982889));
#16347=CARTESIAN_POINT('Ctrl Pts',(0.00189955788753691,-0.0234179665960352,
-0.0105149778851826));
#16348=CARTESIAN_POINT('Ctrl Pts',(0.0017790226651697,-0.0234287661181435,
-0.0103945940109858));
#16349=CARTESIAN_POINT('Ctrl Pts',(0.00144088668856546,-0.0234590618846693,
-0.010056882609542));
#16350=CARTESIAN_POINT('Ctrl Pts',(0.00100221362327,-0.0234893576511951,
-0.00981719643570375));
#16351=CARTESIAN_POINT('Ctrl Pts',(0.000533642873359993,-0.0235196534177209,
-0.00971556234162657));
#16352=CARTESIAN_POINT('Ctrl Pts',(0.00035781701212283,-0.0235310215606156,
-0.00967742530015393));
#16353=CARTESIAN_POINT('Ctrl Pts',(0.000178049411175644,-0.0235423897035102,
-0.00965825721461444));
#16354=CARTESIAN_POINT('Ctrl Pts',(-1.35325041630699E-6,-0.0235537578464049,
-0.00965835365026948));
#16355=CARTESIAN_POINT('Ctrl Pts',(-0.000481224337450019,-0.0235841656622088,
-0.00965861159896546));
#16356=CARTESIAN_POINT('Ctrl Pts',(-0.00096256037853341,-0.0236145734780127,
-0.00980039428131228));
#16357=CARTESIAN_POINT('Ctrl Pts',(-0.00136665501056534,-0.0236449812938166,
-0.0100616015673684));
#16358=CARTESIAN_POINT('Ctrl Pts',(-0.00151623915161095,-0.0236562373874332,
-0.0101582929471155));
#16359=CARTESIAN_POINT('Ctrl Pts',(-0.00165538209716498,-0.0236674934810497,
-0.0102708408343145));
#16360=CARTESIAN_POINT('Ctrl Pts',(-0.0017809366237846,-0.0236787495746663,
-0.0103965076225392));
#16361=CARTESIAN_POINT('Ctrl Pts',(-0.00212005261448095,-0.0237091516751793,
-0.0107359268257637));
#16362=CARTESIAN_POINT('Ctrl Pts',(-0.002360166398731,-0.0237395537756923,
-0.0111764297667141));
#16363=CARTESIAN_POINT('Ctrl Pts',(-0.00246127191791879,-0.0237699558762053,
-0.0116467532997273));
#16364=CARTESIAN_POINT('Ctrl Pts',(-0.00249872429842445,-0.0237812176851127,
-0.0118209746089168));
#16365=CARTESIAN_POINT('Ctrl Pts',(-0.00251756314240969,-0.0237924794940202,
-0.0119990295727695));
#16366=CARTESIAN_POINT('Ctrl Pts',(-0.00251749984030139,-0.0238037413029277,
-0.0121767499930103));
#16367=CARTESIAN_POINT('Ctrl Pts',(-0.00251732895149704,-0.0238341434034407,
-0.0126565196395877));
#16368=CARTESIAN_POINT('Ctrl Pts',(-0.00237569126217508,-0.0238645455039536,
-0.013137797076297));
#16369=CARTESIAN_POINT('Ctrl Pts',(-0.00211464809887879,-0.0238949476044665,
-0.0135418948920403));
#16370=CARTESIAN_POINT('Ctrl Pts',(-0.00201795023353186,-0.023906209413374,
-0.0136915842984982));
#16371=CARTESIAN_POINT('Ctrl Pts',(-0.00190537641728073,-0.0239174712222816,
-0.0138308261240018));
#16372=CARTESIAN_POINT('Ctrl Pts',(-0.00177966860435043,-0.0239287330311891,
-0.013956467199985));
#16373=CARTESIAN_POINT('Ctrl Pts',(-0.0014402471089149,-0.0239591408469931,
-0.0142957085001418));
#16374=CARTESIAN_POINT('Ctrl Pts',(-0.000999692969905732,-0.023989548662797,
-0.0145359242365833));
#16375=CARTESIAN_POINT('Ctrl Pts',(-0.000529287611887201,-0.0240199564786011,
-0.0146370848632089));
#16376=CARTESIAN_POINT('Ctrl Pts',(-0.000355157158661542,-0.0240312125722175,
-0.0146745316002892));
#16377=CARTESIAN_POINT('Ctrl Pts',(-0.000177194252723598,-0.024042468665834,
-0.0146933843058751));
#16378=CARTESIAN_POINT('Ctrl Pts',(4.40162458844756E-7,-0.0240537247594505,
-0.0146933532480789));
#16379=CARTESIAN_POINT('Ctrl Pts',(0.000478543041901331,-0.0240840205259763,
-0.0146932696560462));
#16380=CARTESIAN_POINT('Ctrl Pts',(0.000958311206875898,-0.0241143162925021,
-0.0145526671107832));
#16381=CARTESIAN_POINT('Ctrl Pts',(0.00136152817913595,-0.0241446120590279,
-0.014293410196636));
#16382=CARTESIAN_POINT('Ctrl Pts',(0.00151283077629276,-0.0241559802019226,
-0.0141961269790634));
#16383=CARTESIAN_POINT('Ctrl Pts',(0.00165349975956908,-0.0241673483448172,
-0.0140826575027536));
#16384=CARTESIAN_POINT('Ctrl Pts',(0.00178029114450994,-0.0241787164877119,
-0.0139558447727118));
#16385=CARTESIAN_POINT('Ctrl Pts',(0.0021245284090231,-0.024209580875024,
-0.013611549556476));
#16386=CARTESIAN_POINT('Ctrl Pts',(0.00236663950474416,-0.0242404452623361,
-0.0131635567966713));
#16387=CARTESIAN_POINT('Ctrl Pts',(0.00246546627037973,-0.0242713096496483,
-0.0126850510080965));
#16388=CARTESIAN_POINT('Ctrl Pts',(0.00250004598938024,-0.0242821091717566,
-0.0125176207011081));
#16389=CARTESIAN_POINT('Ctrl Pts',(0.00251749888842494,-0.0242929086938649,
-0.0123466872160051));
#16390=CARTESIAN_POINT('Ctrl Pts',(0.0025174999999467,-0.0243037082159733,
-0.0121758696681072));
#16391=CARTESIAN_POINT('',(0.00251749947769908,-0.0253038475563787,-0.0121769984087159));
#16392=CARTESIAN_POINT('Ctrl Pts',(0.0025174997915076,-0.0243037743898821,
-0.0121748287090009));
#16393=CARTESIAN_POINT('Ctrl Pts',(0.00251730110768886,-0.0243346438561,
-0.0116866407053165));
#16394=CARTESIAN_POINT('Ctrl Pts',(0.00237081488912746,-0.0243655133223179,
-0.0111985313831862));
#16395=CARTESIAN_POINT('Ctrl Pts',(0.00210239121357112,-0.0243963827885358,
-0.0107910220928385));
#16396=CARTESIAN_POINT('Ctrl Pts',(0.00200850477544109,-0.0244071799889846,
-0.0106484877366705));
#16397=CARTESIAN_POINT('Ctrl Pts',(0.00190015429315438,-0.0244179771894333,
-0.0105156667991757));
#16398=CARTESIAN_POINT('Ctrl Pts',(0.00177971076513969,-0.0244287743898821,
-0.0103952815125355));
#16399=CARTESIAN_POINT('Ctrl Pts',(0.00144170260947175,-0.0244590752443175,
-0.0100574368032553));
#16400=CARTESIAN_POINT('Ctrl Pts',(0.0010031185756684,-0.0244893760987529,
-0.00981758055491305));
#16401=CARTESIAN_POINT('Ctrl Pts',(0.000534583810026133,-0.0245196769531884,
-0.00971576662140625));
#16402=CARTESIAN_POINT('Ctrl Pts',(0.000358837011154647,-0.0245310427654196,
-0.00967757634353048));
#16403=CARTESIAN_POINT('Ctrl Pts',(0.000179144120941101,-0.0245424085776508,
-0.00965833954017976));
#16404=CARTESIAN_POINT('Ctrl Pts',(-1.9307286565947E-7,-0.0245537743898821,
-0.0096583532939617));
#16405=CARTESIAN_POINT('Ctrl Pts',(-0.000480067792651366,-0.0245841873000199,
-0.00965839009665786));
#16406=CARTESIAN_POINT('Ctrl Pts',(-0.000961471924135367,-0.0246146002101576,
-0.00979995294595022));
#16407=CARTESIAN_POINT('Ctrl Pts',(-0.00136568830462723,-0.0246450131202954,
-0.0100609770006718));
#16408=CARTESIAN_POINT('Ctrl Pts',(-0.001515261387586,-0.0246562668768243,
-0.0101575643100321));
#16409=CARTESIAN_POINT('Ctrl Pts',(-0.00165440826965524,-0.0246675206333532,
-0.0102700011398836));
#16410=CARTESIAN_POINT('Ctrl Pts',(-0.00177998385649334,-0.0246787743898821,
-0.0103955545137048));
#16411=CARTESIAN_POINT('Ctrl Pts',(-0.00211928394665964,-0.0247091815788996,
-0.0107347945852096));
#16412=CARTESIAN_POINT('Ctrl Pts',(-0.0023596340554676,-0.024739588767917,
-0.0111751722301901));
#16413=CARTESIAN_POINT('Ctrl Pts',(-0.00246099022860495,-0.0247699959569346,
-0.0116454446283417));
#16414=CARTESIAN_POINT('Ctrl Pts',(-0.00249852140471561,-0.0247812554345837,
-0.0118195817888982));
#16415=CARTESIAN_POINT('Ctrl Pts',(-0.002517454866124,-0.024792514912233,
-0.0119975596639281));
#16416=CARTESIAN_POINT('Ctrl Pts',(-0.00251749991904762,-0.0248037743898821,
-0.0121752148547111));
#16417=CARTESIAN_POINT('Ctrl Pts',(-0.00251762158834767,-0.0248341815788995,
-0.0126549879964489));
#16418=CARTESIAN_POINT('Ctrl Pts',(-0.00237627544809769,-0.024864588767917,
-0.0131363544427929));
#16419=CARTESIAN_POINT('Ctrl Pts',(-0.00211547580451566,-0.0248949959569345,
-0.0135406127417401));
#16420=CARTESIAN_POINT('Ctrl Pts',(-0.00201890430768491,-0.0249062554345837,
-0.0136903055423107));
#16421=CARTESIAN_POINT('Ctrl Pts',(-0.00190646228399861,-0.0249175149122329,
-0.0138295681218715));
#16422=CARTESIAN_POINT('Ctrl Pts',(-0.00178088658635174,-0.0249287743898821,
-0.0139552490313413));
#16423=CARTESIAN_POINT('Ctrl Pts',(-0.00144169479371151,-0.0249591873000199,
-0.0142947250110296));
#16424=CARTESIAN_POINT('Ctrl Pts',(-0.00100130174122861,-0.0249896002101577,
-0.0145352427148896));
#16425=CARTESIAN_POINT('Ctrl Pts',(-0.000530962569348486,-0.0250200131202955,
-0.0146367240673897));
#16426=CARTESIAN_POINT('Ctrl Pts',(-0.000356921923374615,-0.0250312668768244,
-0.0146742754371232));
#16427=CARTESIAN_POINT('Ctrl Pts',(-0.000179039012638287,-0.0250425206333532,
-0.0146932491770583));
#16428=CARTESIAN_POINT('Ctrl Pts',(-1.46993648989972E-6,-0.0250537743898821,
-0.0146933528574194));
#16429=CARTESIAN_POINT('Ctrl Pts',(0.000476636615291263,-0.0250840752443175,
-0.0146936320178509));
#16430=CARTESIAN_POINT('Ctrl Pts',(0.000956514274019615,-0.0251143760987529,
-0.0145533914309386));
#16431=CARTESIAN_POINT('Ctrl Pts',(0.00135992934321918,-0.0251446769531883,
-0.0142944373494292));
#16432=CARTESIAN_POINT('Ctrl Pts',(0.00151124982619627,-0.0251560427654196,
-0.0141973040004925));
#16433=CARTESIAN_POINT('Ctrl Pts',(0.001651956748588,-0.0251674085776508,
-0.0140839882941535));
#16434=CARTESIAN_POINT('Ctrl Pts',(0.00177880743895631,-0.0251787743898821,
-0.0139573274921288));
#16435=CARTESIAN_POINT('Ctrl Pts',(0.0021233330233452,-0.0252096438560999,
-0.0136133176431479));
#16436=CARTESIAN_POINT('Ctrl Pts',(0.00236581755152097,-0.0252405133223177,
-0.01316552473233));
#16437=CARTESIAN_POINT('Ctrl Pts',(0.00246504225247071,-0.0252713827885355,
-0.0126870997472149));
#16438=CARTESIAN_POINT('Ctrl Pts',(0.0024997480351387,-0.0252821799889844,
-0.0125197612377771));
#16439=CARTESIAN_POINT('Ctrl Pts',(0.00251734284924451,-0.0252929771894332,
-0.0123489079867308));
#16440=CARTESIAN_POINT('Ctrl Pts',(0.00251749894803741,-0.0253037743898821,
-0.0121781547275306));
#16441=CARTESIAN_POINT('',(0.00251749999991786,-0.0263037743898821,-0.0121758329495021));
#16442=CARTESIAN_POINT('Ctrl Pts',(0.00251749999999526,-0.0253039197054202,
-0.0121758581696978));
#16443=CARTESIAN_POINT('Ctrl Pts',(0.00251750094691551,-0.0253347779048283,
-0.011687673954906));
#16444=CARTESIAN_POINT('Ctrl Pts',(0.00237121650892537,-0.0253656361042366,
-0.0111995079564218));
#16445=CARTESIAN_POINT('Ctrl Pts',(0.00210296312023231,-0.0253964943036448,
-0.0107918907274754));
#16446=CARTESIAN_POINT('Ctrl Pts',(0.00200905712677098,-0.0254072966643753,
-0.010649198398321));
#16447=CARTESIAN_POINT('Ctrl Pts',(0.00190065881351593,-0.0254180990251058,
-0.0105162298587498));
#16448=CARTESIAN_POINT('Ctrl Pts',(0.00178014429023032,-0.0254289013858364,
-0.0103957149335191));
#16449=CARTESIAN_POINT('Ctrl Pts',(0.00144222437939734,-0.0254591909532291,
-0.0100577938956416));
#16450=CARTESIAN_POINT('Ctrl Pts',(0.00100370678302795,-0.0254894805206217,
-0.00981783219268631));
#16451=CARTESIAN_POINT('Ctrl Pts',(0.00053520419770457,-0.0255197700880144,
-0.0097159015153318));
#16452=CARTESIAN_POINT('Ctrl Pts',(0.000359323854807006,-0.0255311410807605,
-0.00967763576601365));
#16453=CARTESIAN_POINT('Ctrl Pts',(0.00017948618320112,-0.0255425120735066,
-0.00965835353703899));
#16454=CARTESIAN_POINT('Ctrl Pts',(3.51331674627921E-9,-0.0255538830662527,
-0.00965835328656055));
#16455=CARTESIAN_POINT('Ctrl Pts',(-0.000479863289043699,-0.0255842846751225,
-0.00965835261687869));
#16456=CARTESIAN_POINT('Ctrl Pts',(-0.000961272249621784,-0.0256146862839923,
-0.00979987342420779));
#16457=CARTESIAN_POINT('Ctrl Pts',(-0.0013655058674309,-0.0256450878928621,
-0.0100608592024028));
#16458=CARTESIAN_POINT('Ctrl Pts',(-0.0015152100039348,-0.025656346844131,
-0.0101575128423852));
#16459=CARTESIAN_POINT('Ctrl Pts',(-0.00165447210278662,-0.0256676057954,
-0.010270043028446));
#16460=CARTESIAN_POINT('Ctrl Pts',(-0.00178013932165148,-0.0256788647466689,
-0.0103957099649376));
#16461=CARTESIAN_POINT('Ctrl Pts',(-0.00211940433969015,-0.0257092606473649,
-0.0107349742206502));
#16462=CARTESIAN_POINT('Ctrl Pts',(-0.00235971476715102,-0.0257396565480609,
-0.0111753655143751));
#16463=CARTESIAN_POINT('Ctrl Pts',(-0.00246103232269861,-0.0257700524487569,
-0.0116456399741708));
#16464=CARTESIAN_POINT('Ctrl Pts',(-0.00249858040427162,-0.0257813171081996,
-0.0118199227397062));
#16465=CARTESIAN_POINT('Ctrl Pts',(-0.00251749984861343,-0.0257925817676425,
-0.0119980510444317));
#16466=CARTESIAN_POINT('Ctrl Pts',(-0.00251749999999909,-0.0258038464270852,
-0.0121758511430643));
#16467=CARTESIAN_POINT('Ctrl Pts',(-0.00251750040848933,-0.0258342423277812,
-0.0126556165695495));
#16468=CARTESIAN_POINT('Ctrl Pts',(-0.00237603695104173,-0.0258646382284771,
-0.0131369412119922));
#16469=CARTESIAN_POINT('Ctrl Pts',(-0.00211514167765687,-0.0258950341291731,
-0.0135411305234001));
#16470=CARTESIAN_POINT('Ctrl Pts',(-0.00201845441596638,-0.0259062987886159,
-0.013690922266338));
#16471=CARTESIAN_POINT('Ctrl Pts',(-0.00190587306977369,-0.0259175634480587,
-0.013830262714367));
#16472=CARTESIAN_POINT('Ctrl Pts',(-0.00178014235301023,-0.0259288281075014,
-0.0139559935768215));
#16473=CARTESIAN_POINT('Ctrl Pts',(-0.00144081420080273,-0.0259592297163713,
-0.0142953221222273));
#16474=CARTESIAN_POINT('Ctrl Pts',(-0.00100032813333106,-0.025989631325241,
-0.0145356543834411));
#16475=CARTESIAN_POINT('Ctrl Pts',(-0.000529953549387098,-0.0260200329341109,
-0.0146369415591505));
#16476=CARTESIAN_POINT('Ctrl Pts',(-0.000355754725191628,-0.0260312918853798,
-0.0146744523165701));
#16477=CARTESIAN_POINT('Ctrl Pts',(-0.0001777149521045,-0.0260425508366488,
-0.0146933532319434));
#16478=CARTESIAN_POINT('Ctrl Pts',(-7.73670714469243E-10,-0.0260538097879177,
-0.014693353286558));
#16479=CARTESIAN_POINT('Ctrl Pts',(0.0004780975372398,-0.0260840993553103,
-0.0146933534334858));
#16480=CARTESIAN_POINT('Ctrl Pts',(0.00095788671648783,-0.026114388922703,
-0.0145528374828911));
#16481=CARTESIAN_POINT('Ctrl Pts',(0.00136114725230904,-0.0261446784900957,
-0.0142936550732066));
#16482=CARTESIAN_POINT('Ctrl Pts',(0.00151253510701687,-0.0261560494828417,
-0.0141963555224329));
#16483=CARTESIAN_POINT('Ctrl Pts',(0.00165328268251051,-0.0261674204755878,
-0.0140828532383766));
#16484=CARTESIAN_POINT('Ctrl Pts',(0.0017801412588749,-0.0261787914683339,
-0.0139559946709575));
#16485=CARTESIAN_POINT('Ctrl Pts',(0.00212440559213063,-0.026209649667664,
-0.0136117303619771));
#16486=CARTESIAN_POINT('Ctrl Pts',(0.00236655410612732,-0.0262405078669941,
-0.0131637604750869));
#16487=CARTESIAN_POINT('Ctrl Pts',(0.0024654220453634,-0.0262713660663242,
-0.0126852650926994));
#16488=CARTESIAN_POINT('Ctrl Pts',(0.00250003216847695,-0.0262821684162683,
-0.0125177610036929));
#16489=CARTESIAN_POINT('Ctrl Pts',(0.00251750000546539,-0.0262929707662124,
-0.0123467490079382));
#16490=CARTESIAN_POINT('Ctrl Pts',(0.0025175,-0.0263037731161565,-0.0121758532060463));
#16491=CARTESIAN_POINT('',(0.00178014132163718,-0.0271787743898721,-0.0139559946081952));
#16492=CARTESIAN_POINT('Ctrl Pts',(0.00251749999991786,-0.0263037743898821,
-0.0121758329495021));
#16493=CARTESIAN_POINT('Ctrl Pts',(0.00251749603863613,-0.0263347748696889,
-0.0116854705911618));
#16494=CARTESIAN_POINT('Ctrl Pts',(0.00236996703968252,-0.0263657753494956,
-0.011195464878576));
#16495=CARTESIAN_POINT('Ctrl Pts',(0.00209960641145874,-0.0263967758293024,
-0.0107868035513213));
#16496=CARTESIAN_POINT('Ctrl Pts',(0.00205200751242907,-0.0264022336828289,
-0.0107148558369625));
#16497=CARTESIAN_POINT('Ctrl Pts',(0.00200072463137587,-0.0264076915363556,
-0.010645383814245));
#16498=CARTESIAN_POINT('Ctrl Pts',(0.00194604252731177,-0.0264131493898821,
-0.0105787544380537));
#16499=CARTESIAN_POINT('Ctrl Pts',(0.00163987935158639,-0.026443707719649,
-0.0102056989062584));
#16500=CARTESIAN_POINT('Ctrl Pts',(0.00122255791486552,-0.0264742660494157,
-0.00992269456928358));
#16501=CARTESIAN_POINT('Ctrl Pts',(0.000761937724844168,-0.0265048243791826,
-0.00977642478096363));
#16502=CARTESIAN_POINT('Ctrl Pts',(0.000673004174330689,-0.0265107243827491,
-0.00974818396154244));
#16503=CARTESIAN_POINT('Ctrl Pts',(0.000582539135272105,-0.0265166243863156,
-0.00972490620853916));
#16504=CARTESIAN_POINT('Ctrl Pts',(0.0004911249259527,-0.0265225243898821,
-0.00970672336751618));
#16505=CARTESIAN_POINT('Ctrl Pts',(1.61855418273218E-5,-0.0265531776557264,
-0.00961225504162464));
#16506=CARTESIAN_POINT('Ctrl Pts',(-0.000487496367874373,-0.0265838309215706,
-0.00965888445140582));
#16507=CARTESIAN_POINT('Ctrl Pts',(-0.000937385750862611,-0.0266144841874148,
-0.00983937854796585));
#16508=CARTESIAN_POINT('Ctrl Pts',(-0.00102258509778175,-0.0266202892549039,
-0.00987356023735698));
#16509=CARTESIAN_POINT('Ctrl Pts',(-0.00110587625694516,-0.026626094322393,
-0.00991239272061271));
#16510=CARTESIAN_POINT('Ctrl Pts',(-0.00118675249474565,-0.0266318993898821,
-0.00995562249535306));
#16511=CARTESIAN_POINT('Ctrl Pts',(-0.00161367118635103,-0.0266625424054887,
-0.0101838180614731));
#16512=CARTESIAN_POINT('Ctrl Pts',(-0.00197335343554593,-0.0266931854210953,
-0.0105392410064605));
#16513=CARTESIAN_POINT('Ctrl Pts',(-0.00220661996526684,-0.0267238284367018,
-0.0109639809422554));
#16514=CARTESIAN_POINT('Ctrl Pts',(-0.00225088842117747,-0.0267296437544286,
-0.0110445865102454));
#16515=CARTESIAN_POINT('Ctrl Pts',(-0.00229071598306191,-0.0267354590721554,
-0.0111275853827044));
#16516=CARTESIAN_POINT('Ctrl Pts',(-0.00232587061440539,-0.0267412743898821,
-0.0112124571400818));
#16517=CARTESIAN_POINT('Ctrl Pts',(-0.00251111310114769,-0.0267719174054887,
-0.0116596771731171));
#16518=CARTESIAN_POINT('Ctrl Pts',(-0.00256368021268813,-0.0268025604210954,
-0.0121625998300799));
#16519=CARTESIAN_POINT('Ctrl Pts',(-0.00247454555743809,-0.0268332034367019,
-0.0126389197333705));
#16520=CARTESIAN_POINT('Ctrl Pts',(-0.00245762991351471,-0.0268390187544287,
-0.0127293139560785));
#16521=CARTESIAN_POINT('Ctrl Pts',(-0.00243576286496692,-0.0268448340721554,
-0.0128187413173178));
#16522=CARTESIAN_POINT('Ctrl Pts',(-0.00240909508136888,-0.0268506493898821,
-0.0129066522595488));
#16523=CARTESIAN_POINT('Ctrl Pts',(-0.00226852586425637,-0.0268813026557263,
-0.0133700418127002));
#16524=CARTESIAN_POINT('Ctrl Pts',(-0.00198997083433534,-0.0269119559215704,
-0.0137922697976542));
#16525=CARTESIAN_POINT('Ctrl Pts',(-0.00161871280581066,-0.0269426091874145,
-0.0141039547108365));
#16526=CARTESIAN_POINT('Ctrl Pts',(-0.00154840454167825,-0.0269484142549037,
-0.014162981111664));
#16527=CARTESIAN_POINT('Ctrl Pts',(-0.00147489407355667,-0.0269542193223929,
-0.0142181323018698));
#16528=CARTESIAN_POINT('Ctrl Pts',(-0.00139864383421296,-0.0269600243898821,
-0.0142690808601912));
#16529=CARTESIAN_POINT('Ctrl Pts',(-0.000997256604347869,-0.026990582719649,
-0.0145372780601776));
#16530=CARTESIAN_POINT('Ctrl Pts',(-0.000515707761662423,-0.0270211410494158,
-0.014686894119793));
#16531=CARTESIAN_POINT('Ctrl Pts',(-3.25563712997477E-5,-0.0270516993791827,
-0.0146931427678629));
#16532=CARTESIAN_POINT('Ctrl Pts',(6.07273568369965E-5,-0.0270575993827492,
-0.0146943492161923));
#16533=CARTESIAN_POINT('Ctrl Pts',(0.000154031385954281,-0.0270634993863156,
-0.0146903637196954));
#16534=CARTESIAN_POINT('Ctrl Pts',(0.000246760680670542,-0.0270693993898821,
-0.0146812305867816));
#16535=CARTESIAN_POINT('Ctrl Pts',(0.000733989645193602,-0.0271003998696892,
-0.0146332422255406));
#16536=CARTESIAN_POINT('Ctrl Pts',(0.00120721401569154,-0.0271314003494962,
-0.0144388319660053));
#16537=CARTESIAN_POINT('Ctrl Pts',(0.00158787431793346,-0.0271624008293032,
-0.0141294298528711));
#16538=CARTESIAN_POINT('Ctrl Pts',(0.00165489225397286,-0.0271678586828295,
-0.0140749574245502));
#16539=CARTESIAN_POINT('Ctrl Pts',(0.00171909554998313,-0.0271733165363559,
-0.0140170403798492));
#16540=CARTESIAN_POINT('Ctrl Pts',(0.00178014132163675,-0.0271787743898821,
-0.0139559946081956));
#16541=CARTESIAN_POINT('',(0.00251838520168631,-0.027178765100316,-0.0121758301112765));
#16542=CARTESIAN_POINT('Origin',(0.,-0.0271787743898824,-0.0121758532865681));
#16543=CARTESIAN_POINT('',(0.00251749968591618,-0.0261786840658975,-0.0121751178742672));
#16544=CARTESIAN_POINT('Ctrl Pts',(0.00251749999997412,-0.0271787629041013,
-0.0121758647020315));
#16545=CARTESIAN_POINT('Ctrl Pts',(0.00251749778631676,-0.0271478961171008,
-0.0126640514115256));
#16546=CARTESIAN_POINT('Ctrl Pts',(0.00237120877539461,-0.0271170293301002,
-0.0131522185239118));
#16547=CARTESIAN_POINT('Ctrl Pts',(0.00210295040354148,-0.0270861625430997,
-0.0135598351687534));
#16548=CARTESIAN_POINT('Ctrl Pts',(0.00200909565457378,-0.0270753632732563,
-0.0137024467771531));
#16549=CARTESIAN_POINT('Ctrl Pts',(0.00190076493421896,-0.027064564003413,
-0.0138353454145956));
#16550=CARTESIAN_POINT('Ctrl Pts',(0.00178033019948072,-0.0270537647335697,
-0.0139558057103091));
#16551=CARTESIAN_POINT('Ctrl Pts',(0.00144244168384373,-0.0270234665868992,
-0.014293765939144));
#16552=CARTESIAN_POINT('Ctrl Pts',(0.00100394391224188,-0.0269931684402286,
-0.0145337743131699));
#16553=CARTESIAN_POINT('Ctrl Pts',(0.000535447156400708,-0.0269628702935582,
-0.0146357521854363));
#16554=CARTESIAN_POINT('Ctrl Pts',(0.000359664149981759,-0.0269515022333864,
-0.0146740149412649));
#16555=CARTESIAN_POINT('Ctrl Pts',(0.000179926162149245,-0.0269401341732146,
-0.0146933148536184));
#16556=CARTESIAN_POINT('Ctrl Pts',(5.38553941159415E-7,-0.0269287661130429,
-0.0146933532289533));
#16557=CARTESIAN_POINT('Ctrl Pts',(-0.00047933341202766,-0.0268983559111435,
-0.0146934558851377));
#16558=CARTESIAN_POINT('Ctrl Pts',(-0.000960776506469032,-0.0268679457092441,
-0.0145520344873474));
#16559=CARTESIAN_POINT('Ctrl Pts',(-0.00136506763759191,-0.0268375355073446,
-0.0142911302411906));
#16560=CARTESIAN_POINT('Ctrl Pts',(-0.00151471159540945,-0.0268262795024018,
-0.0141945593767794));
#16561=CARTESIAN_POINT('Ctrl Pts',(-0.0016539280448862,-0.0268150234974589,
-0.0140821268795949));
#16562=CARTESIAN_POINT('Ctrl Pts',(-0.00177956848708172,-0.0268037674925161,
-0.0139565672584766));
#16563=CARTESIAN_POINT('Ctrl Pts',(-0.00211894582072311,-0.0267733630074777,
-0.0136174082370379));
#16564=CARTESIAN_POINT('Ctrl Pts',(-0.00235939823293213,-0.0267429585224393,
-0.0131770892179304));
#16565=CARTESIAN_POINT('Ctrl Pts',(-0.00246086496060974,-0.0267125540374009,
-0.0127068428303753));
#16566=CARTESIAN_POINT('Ctrl Pts',(-0.00249844790463954,-0.026701292315597,
-0.0125326651066209));
#16567=CARTESIAN_POINT('Ctrl Pts',(-0.00251742343338017,-0.0266900305937932,
-0.0123546400921435));
#16568=CARTESIAN_POINT('Ctrl Pts',(-0.00251749976773793,-0.0266787688719893,
-0.0121769346927993));
#16569=CARTESIAN_POINT('Ctrl Pts',(-0.00251770585583697,-0.026648364386951,
-0.0116971642589626));
#16570=CARTESIAN_POINT('Ctrl Pts',(-0.0023764459218359,-0.0266179599019128,
-0.0112157750511857));
#16571=CARTESIAN_POINT('Ctrl Pts',(-0.00211571967966154,-0.0265875554168744,
-0.0108114719296447));
#16572=CARTESIAN_POINT('Ctrl Pts',(-0.00201914753240536,-0.0265762936950705,
-0.0106617193759164));
#16573=CARTESIAN_POINT('Ctrl Pts',(-0.00190669394497856,-0.0265650319732665,
-0.0105224001585939));
#16574=CARTESIAN_POINT('Ctrl Pts',(-0.00178109766155855,-0.0265537702514625,
-0.0103966688188902));
#16575=CARTESIAN_POINT('Ctrl Pts',(-0.00144194807119419,-0.0265233600495631,
-0.0100571545339503));
#16576=CARTESIAN_POINT('Ctrl Pts',(-0.00100158616073564,-0.0264929498476636,
-0.00981658502841946));
#16577=CARTESIAN_POINT('Ctrl Pts',(-0.000531261451121286,-0.0264625396457643,
-0.00971504701207152));
#16578=CARTESIAN_POINT('Ctrl Pts',(-0.000357175883597738,-0.0264512836408214,
-0.00967746382148041));
#16579=CARTESIAN_POINT('Ctrl Pts',(-0.000179243606041329,-0.0264400276358785,
-0.0096584684082667));
#16580=CARTESIAN_POINT('Ctrl Pts',(-1.62425849082956E-6,-0.0264287716309357,
-0.00965835381053346));
#16581=CARTESIAN_POINT('Ctrl Pts',(0.000476479391155565,-0.0263984734842652,
-0.00965804534416839));
#16582=CARTESIAN_POINT('Ctrl Pts',(0.000956363372561331,-0.0263681753375946,
-0.00979825490116403));
#16583=CARTESIAN_POINT('Ctrl Pts',(0.00135979315423783,-0.026337877190924,
-0.0100571818095027));
#16584=CARTESIAN_POINT('Ctrl Pts',(0.0015111626120142,-0.0263265091307523,
-0.0101543328565972));
#16585=CARTESIAN_POINT('Ctrl Pts',(0.00165191352108424,-0.0263151410705806,
-0.0102676761223036));
#16586=CARTESIAN_POINT('Ctrl Pts',(0.0017788003655274,-0.0263037730104089,
-0.0103943720181751));
#16587=CARTESIAN_POINT('Ctrl Pts',(0.00212332610501935,-0.0262729062223315,
-0.0107383792902235));
#16588=CARTESIAN_POINT('Ctrl Pts',(0.00236581221928291,-0.026242039434254,
-0.0111861696729781));
#16589=CARTESIAN_POINT('Ctrl Pts',(0.00246503937490897,-0.0262111726461765,
-0.0116645929515541));
#16590=CARTESIAN_POINT('Ctrl Pts',(0.00249975615864945,-0.0262003732274117,
-0.0118319797661205));
#16591=CARTESIAN_POINT('Ctrl Pts',(0.00251735203706798,-0.026189573808647,
-0.0120028834728062));
#16592=CARTESIAN_POINT('Ctrl Pts',(0.00251749906725531,-0.0261787743898821,
-0.0121736861758931));
#16593=CARTESIAN_POINT('',(0.00251749999999575,-0.0251788467684986,-0.0121758579128216));
#16594=CARTESIAN_POINT('Ctrl Pts',(0.00251749999998532,-0.0261786382120571,
-0.0121758446897297));
#16595=CARTESIAN_POINT('Ctrl Pts',(0.00251750166704566,-0.0261478195037794,
-0.0126640275621337));
#16596=CARTESIAN_POINT('Ctrl Pts',(0.00237121873593487,-0.0261169959543789,
-0.0131521924775708));
#16597=CARTESIAN_POINT('Ctrl Pts',(0.00200907480146766,-0.0260753702361943,
-0.0137024822819987));
#16598=CARTESIAN_POINT('Ctrl Pts',(0.00190069385417868,-0.0260645767719191,
-0.0138354341741625));
#16599=CARTESIAN_POINT('Ctrl Pts',(0.00144228680867142,-0.0260235087560348,
-0.0142938712727592));
#16600=CARTESIAN_POINT('Ctrl Pts',(0.00100377153889743,-0.0259932243669049,
-0.0145338478358197));
#16601=CARTESIAN_POINT('Ctrl Pts',(0.000359411550730674,-0.0259515769351503,
-0.0146740564015858));
#16602=CARTESIAN_POINT('Ctrl Pts',(0.000179599669795031,-0.0259402111956357,
-0.0146933431974975));
#16603=CARTESIAN_POINT('Ctrl Pts',(-0.000479728532090669,-0.0258984579692366,
-0.0146933802500336));
#16604=CARTESIAN_POINT('Ctrl Pts',(-0.00096114749117309,-0.02586807788922,
-0.0145518840146613));
#16605=CARTESIAN_POINT('Ctrl Pts',(-0.00151508659768241,-0.0258263868848362,
-0.0141942843912173));
#16606=CARTESIAN_POINT('Ctrl Pts',(-0.001654338303916,-0.0258151146282039,
-0.0140817776069311));
#16607=CARTESIAN_POINT('Ctrl Pts',(-0.00211924827589824,-0.0257733778097309,
-0.0136169416575881));
#16608=CARTESIAN_POINT('Ctrl Pts',(-0.00235957857502316,-0.0257428575514638,
-0.01317663284047));
#16609=CARTESIAN_POINT('Ctrl Pts',(-0.00249853586243591,-0.0257012067465951,
-0.0125321165801073));
#16610=CARTESIAN_POINT('Ctrl Pts',(-0.00251748166317325,-0.0256899602890659,
-0.0123539506799638));
#16611=CARTESIAN_POINT('Ctrl Pts',(-0.00251754944298543,-0.0256484646462054,
-0.0116961150930998));
#16612=CARTESIAN_POINT('Ctrl Pts',(-0.00237600299752491,-0.0256183952459406,
-0.011214565160755));
#16613=CARTESIAN_POINT('Ctrl Pts',(-0.00201834470620797,-0.0255771437662403,
-0.0106606690207983));
#16614=CARTESIAN_POINT('Ctrl Pts',(-0.00190592797971776,-0.0255659996184417,
-0.0105215342469508));
#16615=CARTESIAN_POINT('Ctrl Pts',(-0.00144127506136263,-0.0255246811609478,
-0.0100567496024728));
#16616=CARTESIAN_POINT('Ctrl Pts',(-0.00100104799894205,-0.0254943885822059,
-0.00981639652475952));
#16617=CARTESIAN_POINT('Ctrl Pts',(-0.000356473502259796,-0.0254527640577268,
-0.00967733905413254));
#16618=CARTESIAN_POINT('Ctrl Pts',(-0.000178188622811726,-0.0254414908164709,
-0.00965836961475007));
#16619=CARTESIAN_POINT('Ctrl Pts',(0.000477893330868105,-0.0253999078828381,
-0.00965830945616422));
#16620=CARTESIAN_POINT('Ctrl Pts',(0.000957717586045887,-0.0253695618264971,
-0.00979879622724106));
#16621=CARTESIAN_POINT('Ctrl Pts',(0.00151242291956161,-0.0253277393238667,
-0.0101552654986796));
#16622=CARTESIAN_POINT('Ctrl Pts',(0.00165319052650165,-0.0253163151440836,
-0.0102687717440038));
#16623=CARTESIAN_POINT('Ctrl Pts',(0.00212435153890391,-0.0252738555283969,
-0.0107398935001329));
#16624=CARTESIAN_POINT('Ctrl Pts',(0.00236652028836834,-0.02524275925144,
-0.0111878615075769));
#16625=CARTESIAN_POINT('Ctrl Pts',(0.00250002683427236,-0.0252006894127854,
-0.0118338920753196));
#16626=CARTESIAN_POINT('Ctrl Pts',(0.00251750031409437,-0.0251897718623775,
-0.0120049330891682));
#16627=CARTESIAN_POINT('Ctrl Pts',(0.00251749999999575,-0.0251788467684986,
-0.0121758579128216));
#16628=CARTESIAN_POINT('',(0.00251749969152233,-0.0241788307970502,-0.0121767269583493));
#16629=CARTESIAN_POINT('Ctrl Pts',(0.00251749973514484,-0.0251787743898821,
-0.0121770080790441));
#16630=CARTESIAN_POINT('Ctrl Pts',(0.00251727580147127,-0.0251479127705137,
-0.0126651935935195));
#16631=CARTESIAN_POINT('Ctrl Pts',(0.00237076574137828,-0.0251170511511452,
-0.0131532932779853));
#16632=CARTESIAN_POINT('Ctrl Pts',(0.00210232333480158,-0.0250861895317767,
-0.0135607875254116));
#16633=CARTESIAN_POINT('Ctrl Pts',(0.00200837910505686,-0.0250753891850758,
-0.0137033944022015));
#16634=CARTESIAN_POINT('Ctrl Pts',(0.0018999556107474,-0.025064588838375,
-0.0138362765659917));
#16635=CARTESIAN_POINT('Ctrl Pts',(0.00177942802041401,-0.0250537884916741,
-0.0139567076237136));
#16636=CARTESIAN_POINT('Ctrl Pts',(0.00144137008933471,-0.0250234954869726,
-0.0142944947984056));
#16637=CARTESIAN_POINT('Ctrl Pts',(0.00100275316589472,-0.024993202482271,
-0.0145342805422729));
#16638=CARTESIAN_POINT('Ctrl Pts',(0.000534207011796535,-0.0249629094775695,
-0.0146360218008163));
#16639=CARTESIAN_POINT('Ctrl Pts',(0.000358361691154154,-0.0249515405162017,
-0.0146742052840754));
#16640=CARTESIAN_POINT('Ctrl Pts',(0.000178569011540147,-0.0249401715548339,
-0.0146934145998264));
#16641=CARTESIAN_POINT('Ctrl Pts',(-8.62323990597464E-7,-0.0249288025934661,
-0.0146933531388714));
#16642=CARTESIAN_POINT('Ctrl Pts',(-0.000480731892182397,-0.02489839754428,
-0.0146931887682397));
#16643=CARTESIAN_POINT('Ctrl Pts',(-0.000962094346738138,-0.0248679924950939,
-0.0145515008288072));
#16644=CARTESIAN_POINT('Ctrl Pts',(-0.00136623928899328,-0.0248375874459078,
-0.0142903736707614));
#16645=CARTESIAN_POINT('Ctrl Pts',(-0.00151586660897812,-0.0248263305290246,
-0.0141936960861908));
#16646=CARTESIAN_POINT('Ctrl Pts',(-0.00165505246021516,-0.0248150736121414,
-0.0140811547956854));
#16647=CARTESIAN_POINT('Ctrl Pts',(-0.00178064760153243,-0.0248038166952582,
-0.0139554881842708));
#16648=CARTESIAN_POINT('Ctrl Pts',(-0.00211981764331208,-0.0247734173587111,
-0.0136161251372869));
#16649=CARTESIAN_POINT('Ctrl Pts',(-0.0023600027298034,-0.024743018022164,
-0.0131756626469667));
#16650=CARTESIAN_POINT('Ctrl Pts',(-0.00246118512021359,-0.024712618685617,
-0.012705356878651));
#16651=CARTESIAN_POINT('Ctrl Pts',(-0.00249867211522085,-0.0247013560560947,
-0.0125311136144103));
#16652=CARTESIAN_POINT('Ctrl Pts',(-0.0025175401703522,-0.0246900934265724,
-0.0123530324036204));
#16653=CARTESIAN_POINT('Ctrl Pts',(-0.00251749993550441,-0.0246788307970502,
-0.0121752834310746));
#16654=CARTESIAN_POINT('Ctrl Pts',(-0.00251739133629353,-0.0246484314605032,
-0.0116955152893069));
#16655=CARTESIAN_POINT('Ctrl Pts',(-0.00237581698877943,-0.0246180321239562,
-0.0112142206619956));
#16656=CARTESIAN_POINT('Ctrl Pts',(-0.00211482758018363,-0.0245876327874092,
-0.0108100895602516));
#16657=CARTESIAN_POINT('Ctrl Pts',(-0.00201813379169509,-0.0245763701578869,
-0.010660363303221));
#16658=CARTESIAN_POINT('Ctrl Pts',(-0.00190555753629768,-0.0245651075283645,
-0.0105210859285633));
#16659=CARTESIAN_POINT('Ctrl Pts',(-0.0017798417509926,-0.0245538448988422,
-0.0103954124446811));
#16660=CARTESIAN_POINT('Ctrl Pts',(-0.00144045434345245,-0.0245234398496561,
-0.0100561392357694));
#16661=CARTESIAN_POINT('Ctrl Pts',(-0.000999925048114809,-0.0244930348004701,
-0.00981588090801228));
#16662=CARTESIAN_POINT('Ctrl Pts',(-0.000529530905128816,-0.0244626297512839,
-0.00971467404267653));
#16663=CARTESIAN_POINT('Ctrl Pts',(-0.000355376022578128,-0.0244513728344007,
-0.00967720404010807));
#16664=CARTESIAN_POINT('Ctrl Pts',(-0.00017738560890287,-0.0244401159175175,
-0.00965833372630848));
#16665=CARTESIAN_POINT('Ctrl Pts',(2.77386968701596E-7,-0.0244288590006343,
-0.00965835330183983));
#16666=CARTESIAN_POINT('Ctrl Pts',(0.000478378631302506,-0.0243985659959327,
-0.00965840598071002));
#16667=CARTESIAN_POINT('Ctrl Pts',(0.000958154594833885,-0.0243682729912311,
-0.00979897658696198));
#16668=CARTESIAN_POINT('Ctrl Pts',(0.00136138767051821,-0.0243379799865295,
-0.0100582060400694));
#16669=CARTESIAN_POINT('Ctrl Pts',(0.001512720999939,-0.0243266110251618,
-0.0101554948256089));
#16670=CARTESIAN_POINT('Ctrl Pts',(0.00165341835785117,-0.0243152420637941,
-0.0102689757919928));
#16671=CARTESIAN_POINT('Ctrl Pts',(0.00178023405819179,-0.0243038731024263,
-0.010395804706307));
#16672=CARTESIAN_POINT('Ctrl Pts',(0.00212448167653426,-0.0242730114830577,
-0.0107400881946476));
#16673=CARTESIAN_POINT('Ctrl Pts',(0.00236660703117265,-0.0242421498636891,
-0.011188072299693));
#16674=CARTESIAN_POINT('Ctrl Pts',(0.00246544945886431,-0.0242112882443205,
-0.0116665741727259));
#16675=CARTESIAN_POINT('Ctrl Pts',(0.00250004040093587,-0.0242004878976197,
-0.0118340309112719));
#16676=CARTESIAN_POINT('Ctrl Pts',(0.00251749897647234,-0.0241896875509191,
-0.0120049925568173));
#16677=CARTESIAN_POINT('Ctrl Pts',(0.00251749999995483,-0.0241788872042183,
-0.0121758382050082));
#16678=CARTESIAN_POINT('',(0.00251749961839117,-0.0231787088666403,-0.0121748943155386));
#16679=CARTESIAN_POINT('Ctrl Pts',(0.00251749938308983,-0.0241787743898821,
-0.0121776157116905));
#16680=CARTESIAN_POINT('Ctrl Pts',(0.00251715761715276,-0.0241479040557949,
-0.0126658041288309));
#16681=CARTESIAN_POINT('Ctrl Pts',(0.00237052806672346,-0.0241170337217076,
-0.0131538709062047));
#16682=CARTESIAN_POINT('Ctrl Pts',(0.00210198450028724,-0.0240861633876204,
-0.0135613017376209));
#16683=CARTESIAN_POINT('Ctrl Pts',(0.00200806631828363,-0.024075367055041,
-0.013703793190634));
#16684=CARTESIAN_POINT('Ctrl Pts',(0.00189969006379212,-0.0240645707224615,
-0.0138365690828121));
#16685=CARTESIAN_POINT('Ctrl Pts',(0.0017792267323238,-0.0240537743898821,
-0.0139569087278581));
#16686=CARTESIAN_POINT('Ctrl Pts',(0.00144112599332246,-0.0240234726542492,
-0.0142946623199701));
#16687=CARTESIAN_POINT('Ctrl Pts',(0.00100247575010198,-0.0239931709186162,
-0.0145343995217319));
#16688=CARTESIAN_POINT('Ctrl Pts',(0.000533912379734766,-0.0239628691829833,
-0.0146360857594691));
#16689=CARTESIAN_POINT('Ctrl Pts',(0.000358173588608443,-0.0239515042519495,
-0.0146742240725006));
#16690=CARTESIAN_POINT('Ctrl Pts',(0.000178494707472031,-0.0239401393209158,
-0.0146934118272028));
#16691=CARTESIAN_POINT('Ctrl Pts',(-8.23759858439146E-7,-0.0239287743898821,
-0.0146933531517854));
#16692=CARTESIAN_POINT('Ctrl Pts',(-0.000480699474097822,-0.0238983605988304,
-0.0146931961299894));
#16693=CARTESIAN_POINT('Ctrl Pts',(-0.000962068926494477,-0.0238679468077788,
-0.0145515121105112));
#16694=CARTESIAN_POINT('Ctrl Pts',(-0.0013662203064985,-0.0238375330167271,
-0.0142903859356584));
#16695=CARTESIAN_POINT('Ctrl Pts',(-0.00151575329964231,-0.0238262801411121,
-0.0141937712005719));
#16696=CARTESIAN_POINT('Ctrl Pts',(-0.00165485831852499,-0.023815027265497,
-0.0140813129275911));
#16697=CARTESIAN_POINT('Ctrl Pts',(-0.00178039192185105,-0.0238037743898821,
-0.013955743972698));
#16698=CARTESIAN_POINT('Ctrl Pts',(-0.00211961493681556,-0.0237733663215084,
-0.0136164254290078));
#16699=CARTESIAN_POINT('Ctrl Pts',(-0.00235986424518859,-0.0237429582531347,
-0.0131759917540072));
#16700=CARTESIAN_POINT('Ctrl Pts',(-0.00246111229587264,-0.023712550184761,
-0.0127056952602677));
#16701=CARTESIAN_POINT('Ctrl Pts',(-0.00249859942318996,-0.0237012915864681,
-0.012531567813679));
#16702=CARTESIAN_POINT('Ctrl Pts',(-0.00251749188956349,-0.023690032988175,
-0.0123536047447747));
#16703=CARTESIAN_POINT('Ctrl Pts',(-0.0025174999973777,-0.0236787743898821,
-0.0121759681920881));
#16704=CARTESIAN_POINT('Ctrl Pts',(-0.00251752189557162,-0.0236483663215085,
-0.0116961940408852));
#16705=CARTESIAN_POINT('Ctrl Pts',(-0.00237607509735981,-0.0236179582531348,
-0.011214856218412));
#16706=CARTESIAN_POINT('Ctrl Pts',(-0.00211519055100145,-0.0235875501847612,
-0.0108106517692156));
#16707=CARTESIAN_POINT('Ctrl Pts',(-0.00201859795352949,-0.0235762915864682,
-0.0106609949259775));
#16708=CARTESIAN_POINT('Ctrl Pts',(-0.0019061403672986,-0.0235650329881751,
-0.0105217694096613));
#16709=CARTESIAN_POINT('Ctrl Pts',(-0.00178055439251249,-0.0235537743898821,
-0.0103961251316691));
#16710=CARTESIAN_POINT('Ctrl Pts',(-0.00144129851920226,-0.0235233605988305,
-0.0100567117590432));
#16711=CARTESIAN_POINT('Ctrl Pts',(-0.0010008596088619,-0.0234929468077789,
-0.0098162761052494));
#16712=CARTESIAN_POINT('Ctrl Pts',(-0.0005305006030715,-0.0234625330167273,
-0.00971488287630511));
#16713=CARTESIAN_POINT('Ctrl Pts',(-0.000356471282701629,-0.0234512801411122,
-0.00967736813861314));
#16714=CARTESIAN_POINT('Ctrl Pts',(-0.000178603996301796,-0.0234400272654971,
-0.00965842781167594));
#16715=CARTESIAN_POINT('Ctrl Pts',(-1.0535709026251E-6,-0.0234287743898821,
-0.00965835350701722));
#16716=CARTESIAN_POINT('Ctrl Pts',(0.000477054091173907,-0.0233984726542492,
-0.00965815341948388));
#16717=CARTESIAN_POINT('Ctrl Pts',(0.000956909392876984,-0.0233681709186163,
-0.00979847396983194));
#16718=CARTESIAN_POINT('Ctrl Pts',(0.00136028205916767,-0.0233378691829834,
-0.0100574956752218));
#16719=CARTESIAN_POINT('Ctrl Pts',(0.00151157050643154,-0.0233265042519496,
-0.0101546440317934));
#16720=CARTESIAN_POINT('Ctrl Pts',(0.00165224493730612,-0.0233151393209159,
-0.0102679695719795));
#16721=CARTESIAN_POINT('Ctrl Pts',(0.00177906414050594,-0.0233037743898821,
-0.0103946354352087));
#16722=CARTESIAN_POINT('Ctrl Pts',(0.00212354059705622,-0.0232729040557949,
-0.0107386953774739));
#16723=CARTESIAN_POINT('Ctrl Pts',(0.00236596066449794,-0.0232420337217078,
-0.0111865238080445));
#16724=CARTESIAN_POINT('Ctrl Pts',(0.0024651162146737,-0.0232111633876205,
-0.0116649635742397));
#16725=CARTESIAN_POINT('Ctrl Pts',(0.00249979404788967,-0.0232003670550411,
-0.0118322890984952));
#16726=CARTESIAN_POINT('Ctrl Pts',(0.00251736409974424,-0.0231895707224615,
-0.0120031261261098));
#16727=CARTESIAN_POINT('Ctrl Pts',(0.0025174992117169,-0.0231787743898821,
-0.0121738610504294));
#16728=CARTESIAN_POINT('Ctrl Pts',(0.00251749999997788,-0.0231786473855,
-0.0121758638389549));
#16729=CARTESIAN_POINT('Ctrl Pts',(0.00251749795369238,-0.0231477868810446,
-0.0126640490203062));
#16730=CARTESIAN_POINT('Ctrl Pts',(0.00237120997493988,-0.0231169263765892,
-0.0131522149255864));
#16731=CARTESIAN_POINT('Ctrl Pts',(0.0021029531720672,-0.0230860658721338,
-0.0135598309619895));
#16732=CARTESIAN_POINT('Ctrl Pts',(0.00200906595270055,-0.0230752650017718,
-0.0137024925303722));
#16733=CARTESIAN_POINT('Ctrl Pts',(0.00190069260959032,-0.0230644641314098,
-0.0138354343323198));
#16734=CARTESIAN_POINT('Ctrl Pts',(0.00178020769704895,-0.0230536632610477,
-0.0139559282303084));
#16735=CARTESIAN_POINT('Ctrl Pts',(0.00144229831669849,-0.0230233713735881,
-0.01429386281105));
#16736=CARTESIAN_POINT('Ctrl Pts',(0.00100378724406002,-0.0229930794861285,
-0.0145338404708914));
#16737=CARTESIAN_POINT('Ctrl Pts',(0.000535286428431861,-0.0229627875986689,
-0.0146357871656566));
#16738=CARTESIAN_POINT('Ctrl Pts',(0.000359443503242876,-0.0229514181113111,
-0.0146740509304631));
#16739=CARTESIAN_POINT('Ctrl Pts',(0.000179644245441134,-0.0229400486239533,
-0.0146933391444727));
#16740=CARTESIAN_POINT('Ctrl Pts',(1.98293912005771E-7,-0.0229286791365955,
-0.0146933532787487));
#16741=CARTESIAN_POINT('Ctrl Pts',(-0.000479670505837759,-0.0228982752060211,
-0.0146933910761913));
#16742=CARTESIAN_POINT('Ctrl Pts',(-0.00096109198559297,-0.0228678712754467,
-0.0145519063931369));
#16743=CARTESIAN_POINT('Ctrl Pts',(-0.0013653465885999,-0.0228374673448723,
-0.0142909501975763));
#16744=CARTESIAN_POINT('Ctrl Pts',(-0.00151502702686396,-0.0228262099006293,
-0.0141943278278402));
#16745=CARTESIAN_POINT('Ctrl Pts',(-0.00165427096627102,-0.0228149524563863,
-0.0140818347223467));
#16746=CARTESIAN_POINT('Ctrl Pts',(-0.00177992725547758,-0.0228036950121433,
-0.0139562086486159));
#16747=CARTESIAN_POINT('Ctrl Pts',(-0.00211923405946871,-0.0227732967929111,
-0.0136169834347829));
#16748=CARTESIAN_POINT('Ctrl Pts',(-0.00235959725416242,-0.022742898573679,
-0.0131766189178827));
#16749=CARTESIAN_POINT('Ctrl Pts',(-0.0024609702103146,-0.0227125003544468,
-0.0127063548171347));
#16750=CARTESIAN_POINT('Ctrl Pts',(-0.00249853094269033,-0.0227012371988616,
-0.0125321124481187));
#16751=CARTESIAN_POINT('Ctrl Pts',(-0.00251747121844593,-0.0226899740432763,
-0.0123540239500127));
#16752=CARTESIAN_POINT('Ctrl Pts',(-0.00251749996707782,-0.022678710887691,
-0.0121762604267775));
#16753=CARTESIAN_POINT('Ctrl Pts',(-0.00251757755698666,-0.0226483126684587,
-0.0116964930551988));
#16754=CARTESIAN_POINT('Ctrl Pts',(-0.00237619043761343,-0.0226179144492263,
-0.0112151441306248));
#16755=CARTESIAN_POINT('Ctrl Pts',(-0.00211535854080719,-0.022587516229994,
-0.0108109120812917));
#16756=CARTESIAN_POINT('Ctrl Pts',(-0.00201871504294884,-0.0225762530744089,
-0.0106611359240335));
#16757=CARTESIAN_POINT('Ctrl Pts',(-0.00190618239367656,-0.0225649899188239,
-0.0105218041976827));
#16758=CARTESIAN_POINT('Ctrl Pts',(-0.0017805030148144,-0.0225537267632388,
-0.0103960737316028));
#16759=CARTESIAN_POINT('Ctrl Pts',(-0.00144124222056347,-0.0225233228326644,
-0.0100566750317524));
#16760=CARTESIAN_POINT('Ctrl Pts',(-0.00100080296046634,-0.0224929189020899,
-0.00981625320281795));
#16761=CARTESIAN_POINT('Ctrl Pts',(-0.000530447146739297,-0.0224625149715155,
-0.00971487135356547));
#16762=CARTESIAN_POINT('Ctrl Pts',(-0.000356291889594958,-0.0224512575272725,
-0.00967733342693407));
#16763=CARTESIAN_POINT('Ctrl Pts',(-0.000178293543672711,-0.0224400000830296,
-0.0096583968363908));
#16764=CARTESIAN_POINT('Ctrl Pts',(-6.15986524236793E-7,-0.0224287426387866,
-0.00965835336191846));
#16765=CARTESIAN_POINT('Ctrl Pts',(0.000477484410783648,-0.022398450751327,
-0.00965823637943155));
#16766=CARTESIAN_POINT('Ctrl Pts',(0.000957309569357418,-0.0223681588638674,
-0.00979863625329785));
#16767=CARTESIAN_POINT('Ctrl Pts',(0.00136063427525223,-0.0223378669764078,
-0.0100577218886017));
#16768=CARTESIAN_POINT('Ctrl Pts',(0.00151201457966164,-0.02232649748905,
-0.0101549647843806));
#16769=CARTESIAN_POINT('Ctrl Pts',(0.00165276292502887,-0.0223151280016921,
-0.0102684063031234));
#16770=CARTESIAN_POINT('Ctrl Pts',(0.00177963184218455,-0.0223037585143343,
-0.0103952026312405));
#16771=CARTESIAN_POINT('Ctrl Pts',(0.00212399554653551,-0.0222728980098791,
-0.0107393693052175));
#16772=CARTESIAN_POINT('Ctrl Pts',(0.00236627236577061,-0.0222420375054239,
-0.01118727103047));
#16773=CARTESIAN_POINT('Ctrl Pts',(0.0024652768054868,-0.0222111770009687,
-0.0116657390617723));
#16774=CARTESIAN_POINT('Ctrl Pts',(0.00249992737706798,-0.0222003761306065,
-0.0118331981253807));
#16775=CARTESIAN_POINT('Ctrl Pts',(0.00251744388437495,-0.0221895752602443,
-0.0120041684931912));
#16776=CARTESIAN_POINT('Ctrl Pts',(0.00251749986487603,-0.0221787743898821,
-0.0121750284537333));
#16777=CARTESIAN_POINT('',(-0.00251750000001,-0.00883413153273949,-0.012175853286568));
#16778=CARTESIAN_POINT('Origin',(0.,-0.00883413153273949,-0.012175853286568));
#16779=CARTESIAN_POINT('Origin',(0.,0.0154212256101276,-0.012175853286558));
#16780=CARTESIAN_POINT('',(0.004,0.0153212256101276,-0.012175853286558));
#16781=CARTESIAN_POINT('Origin',(0.,0.0153212256101176,-0.012175853286568));
#16782=CARTESIAN_POINT('',(0.0042,0.0155212256101276,-0.012175853286558));
#16783=CARTESIAN_POINT('',(0.0041,0.0154212256101276,-0.012175853286558));
#16784=CARTESIAN_POINT('Origin',(0.,0.0155212256101176,-0.012175853286568));
#16785=CARTESIAN_POINT('Origin',(0.,0.0155212256101276,-0.012175853286558));
#16786=CARTESIAN_POINT('',(-0.0078,0.0155212256101276,-0.012175853286558));
#16787=CARTESIAN_POINT('Origin',(0.,0.0155212256101176,-0.012175853286568));
#16788=CARTESIAN_POINT('Origin',(0.,0.0155212256101279,-0.012175853286558));
#16789=CARTESIAN_POINT('',(0.004,0.00902122561010792,-0.012175853286558));
#16790=CARTESIAN_POINT('',(0.004,0.0155212256101279,-0.012175853286558));
#16791=CARTESIAN_POINT('',(-0.00400000000001,0.00902122561011792,-0.012175853286568));
#16792=CARTESIAN_POINT('Origin',(0.,0.00902122561011792,-0.012175853286568));
#16793=CARTESIAN_POINT('Origin',(0.,0.00902122561011792,-0.012175853286568));
#16794=CARTESIAN_POINT('Origin',(0.,0.0119212256101276,-0.012175853286558));
#16795=CARTESIAN_POINT('',(-0.008,0.0120212256101276,-0.012175853286558));
#16796=CARTESIAN_POINT('Origin',(0.,0.0120212256101176,-0.012175853286568));
#16797=CARTESIAN_POINT('',(-0.0078,0.0118212256101276,-0.012175853286558));
#16798=CARTESIAN_POINT('',(-0.0079,0.0119212256101276,-0.012175853286558));
#16799=CARTESIAN_POINT('Origin',(0.,0.0118212256101176,-0.012175853286568));
#16800=CARTESIAN_POINT('Origin',(0.,0.0188212256101277,-0.012175853286558));
#16801=CARTESIAN_POINT('',(-0.008,0.0153212256101276,-0.012175853286558));
#16802=CARTESIAN_POINT('',(-0.008,0.0188212256101277,-0.012175853286558));
#16803=CARTESIAN_POINT('Origin',(0.,0.0153212256101176,-0.012175853286568));
#16804=CARTESIAN_POINT('Origin',(0.,0.0118212256101276,-0.012175853286558));
#16805=CARTESIAN_POINT('',(0.006,0.0118212256101276,-0.012175853286558));
#16806=CARTESIAN_POINT('Origin',(0.,0.0118212256101176,-0.012175853286568));
#16807=CARTESIAN_POINT('Origin',(0.,0.0154212256101276,-0.012175853286558));
#16808=CARTESIAN_POINT('',(-0.0079,0.0154212256101276,-0.012175853286558));
#16809=CARTESIAN_POINT('Origin',(0.,0.00807122561012792,-0.012175853286558));
#16810=CARTESIAN_POINT('',(0.00210000000001,0.00712122561011792,-0.012175853286568));
#16811=CARTESIAN_POINT('',(-0.0021,0.00712122561012792,-0.012175853286558));
#16812=CARTESIAN_POINT('Origin',(0.,0.00712122561011792,-0.012175853286568));
#16813=CARTESIAN_POINT('',(-0.00305,0.00807122561012792,-0.012175853286558));
#16814=CARTESIAN_POINT('Origin',(0.,0.00712122561011792,-0.012175853286568));
#16815=CARTESIAN_POINT('Origin',(0.,0.0155212256101279,-0.012175853286558));
#16816=CARTESIAN_POINT('',(0.0021,-0.00853591724703519,-0.012175853286558));
#16817=CARTESIAN_POINT('',(0.0021,0.0155212256101279,-0.012175853286558));
#16818=CARTESIAN_POINT('',(-0.00210000000001,-0.00853591724702519,-0.012175853286568));
#16819=CARTESIAN_POINT('Origin',(0.,-0.00853591724702519,-0.012175853286568));
#16820=CARTESIAN_POINT('Origin',(0.,-0.00853591724702519,-0.012175853286568));
#16821=CARTESIAN_POINT('Origin',(3.42660592399111E-19,-0.0131787743898721,
-0.012175853286558));
#16822=CARTESIAN_POINT('Ctrl Pts',(0.00251750000000276,-0.0131787743898705,
-0.0121758532865581));
#16823=CARTESIAN_POINT('Ctrl Pts',(0.00252678255386265,-0.0131787743898701,
-0.0120910805509574));
#16824=CARTESIAN_POINT('Ctrl Pts',(0.00253138326894594,-0.0131787743898702,
-0.0120060302520078));
#16825=CARTESIAN_POINT('Ctrl Pts',(0.00253153840791565,-0.0131787743898704,
-0.011920995628507));
#16826=CARTESIAN_POINT('Ctrl Pts',(0.00253173885754197,-0.0131787743898706,
-0.0118111253713033));
#16827=CARTESIAN_POINT('Ctrl Pts',(0.00252452176116332,-0.0131787743898709,
-0.0117012808905388));
#16828=CARTESIAN_POINT('Ctrl Pts',(0.00251027895179543,-0.0131787743898711,
-0.01159205956687));
#16829=CARTESIAN_POINT('Ctrl Pts',(0.00250787645068956,-0.0131787743898711,
-0.0115736359297827));
#16830=CARTESIAN_POINT('Ctrl Pts',(0.0025052735027393,-0.0131787743898712,
-0.0115552290376494));
#16831=CARTESIAN_POINT('Ctrl Pts',(0.00250247449001427,-0.0131787743898712,
-0.0115368584649061));
#16832=CARTESIAN_POINT('Ctrl Pts',(0.0024778848322329,-0.0131787743898716,
-0.0113754708109787));
#16833=CARTESIAN_POINT('Ctrl Pts',(0.00243817399752059,-0.0131787743898719,
-0.0112165929618383));
#16834=CARTESIAN_POINT('Ctrl Pts',(0.00238459006941217,-0.0131787743898722,
-0.0110621287890247));
#16835=CARTESIAN_POINT('Ctrl Pts',(0.00237038445925664,-0.0131787743898723,
-0.0110211788643095));
#16836=CARTESIAN_POINT('Ctrl Pts',(0.00235519109693126,-0.0131787743898724,
-0.0109805154528752));
#16837=CARTESIAN_POINT('Ctrl Pts',(0.00233906126070756,-0.0131787743898725,
-0.0109402583288236));
#16838=CARTESIAN_POINT('Ctrl Pts',(0.00223492121084125,-0.0131787743898731,
-0.0106803437923044));
#16839=CARTESIAN_POINT('Ctrl Pts',(0.00209239429727179,-0.0131787743898737,
-0.0104379417852556));
#16840=CARTESIAN_POINT('Ctrl Pts',(0.0019166248406654,-0.0131787743898743,
-0.0102221995812248));
#16841=CARTESIAN_POINT('Ctrl Pts',(0.00188608523662504,-0.0131787743898744,
-0.0101847147894236));
#16842=CARTESIAN_POINT('Ctrl Pts',(0.0018545322737917,-0.0131787743898745,
-0.0101480373230837));
#16843=CARTESIAN_POINT('Ctrl Pts',(0.00182198107674273,-0.0131787743898746,
-0.0101122201309508));
#16844=CARTESIAN_POINT('Ctrl Pts',(0.00180781807866736,-0.0131787743898747,
-0.0100966361011997));
#16845=CARTESIAN_POINT('Ctrl Pts',(0.00179346144536564,-0.0131787743898747,
-0.0100812103074837));
#16846=CARTESIAN_POINT('Ctrl Pts',(0.00177893734013724,-0.0131787743898748,
-0.0100659730452282));
#16847=CARTESIAN_POINT('Ctrl Pts',(0.00171287262328748,-0.013178774389875,
-0.0099966644440688));
#16848=CARTESIAN_POINT('Ctrl Pts',(0.00164327513476541,-0.0131787743898752,
-0.00993117167958241));
#16849=CARTESIAN_POINT('Ctrl Pts',(0.00157035138407573,-0.0131787743898754,
-0.00986983987978509));
#16850=CARTESIAN_POINT('Ctrl Pts',(0.00155126698510032,-0.0131787743898755,
-0.00985378913464181));
#16851=CARTESIAN_POINT('Ctrl Pts',(0.00153195451165503,-0.0131787743898756,
-0.00983802345570631));
#16852=CARTESIAN_POINT('Ctrl Pts',(0.00151241711792581,-0.0131787743898756,
-0.00982254925039919));
#16853=CARTESIAN_POINT('Ctrl Pts',(0.00133945071125891,-0.0131787743898762,
-0.00968555463765327));
#16854=CARTESIAN_POINT('Ctrl Pts',(0.00114895456192055,-0.0131787743898767,
-0.00957130583923114));
#16855=CARTESIAN_POINT('Ctrl Pts',(0.000945893407857157,-0.0131787743898771,
-0.00947984027712986));
#16856=CARTESIAN_POINT('Ctrl Pts',(0.00092821365265431,-0.0131787743898771,
-0.00947187672174231));
#16857=CARTESIAN_POINT('Ctrl Pts',(0.000910433722123745,-0.0131787743898772,
-0.00946408495197249));
#16858=CARTESIAN_POINT('Ctrl Pts',(0.0008925836998557,-0.0131787743898772,
-0.00945647668080864));
#16859=CARTESIAN_POINT('Ctrl Pts',(0.000622478384141858,-0.0131787743898778,
-0.0093413488420928));
#16860=CARTESIAN_POINT('Ctrl Pts',(0.000335493839089116,-0.0131787743898777,
-0.00926745536012451));
#16861=CARTESIAN_POINT('Ctrl Pts',(4.26963611125967E-5,-0.0131787743898794,
-0.00923485885680396));
#16862=CARTESIAN_POINT('Ctrl Pts',(-1.2995058917788E-5,-0.0131787743898797,
-0.00922865885272438));
#16863=CARTESIAN_POINT('Ctrl Pts',(-6.890315766291E-5,-0.0131787743898796,
-0.00922396320906305));
#16864=CARTESIAN_POINT('Ctrl Pts',(-0.000124958449797895,-0.0131787743898795,
-0.00922078757979583));
#16865=CARTESIAN_POINT('Ctrl Pts',(-0.000141877207563949,-0.0131787743898795,
-0.00921982910290131));
#16866=CARTESIAN_POINT('Ctrl Pts',(-0.00015880937860213,-0.0131787743898795,
-0.00921900913120467));
#16867=CARTESIAN_POINT('Ctrl Pts',(-0.000175753060180348,-0.0131787743898794,
-0.00921832819105194));
#16868=CARTESIAN_POINT('Ctrl Pts',(-0.000190844981741937,-0.0131787743898794,
-0.00921772167024798));
#16869=CARTESIAN_POINT('Ctrl Pts',(-0.000205937547985643,-0.0131787743898794,
-0.00921722581492978));
#16870=CARTESIAN_POINT('Ctrl Pts',(-0.000221025143038285,-0.0131787743898794,
-0.00921684070026162));
#16871=CARTESIAN_POINT('Ctrl Pts',(-0.000581851158293263,-0.0131787743898789,
-0.00920763052523738));
#16872=CARTESIAN_POINT('Ctrl Pts',(-0.000940457786385863,-0.0131787743898784,
-0.00926106964733248));
#16873=CARTESIAN_POINT('Ctrl Pts',(-0.00127835860631399,-0.0131787743898775,
-0.00937986338687581));
#16874=CARTESIAN_POINT('Ctrl Pts',(-0.00129490141823496,-0.0131787743898775,
-0.00938567924281564));
#16875=CARTESIAN_POINT('Ctrl Pts',(-0.0013113946141123,-0.0131787743898372,
-0.00939165340181671));
#16876=CARTESIAN_POINT('Ctrl Pts',(-0.00132783707045352,-0.0131787743898773,
-0.00939778432924211));
#16877=CARTESIAN_POINT('Ctrl Pts',(-0.00289832479094294,-0.0131787743898724,
-0.0131986512412907));
#16878=CARTESIAN_POINT('Ctrl Pts',(-0.00285634487132818,-0.0131787743898806,
-0.0132905010317887));
#16879=CARTESIAN_POINT('Ctrl Pts',(-0.00280954766287239,-0.0131787743898807,
-0.0133799217860521));
#16880=CARTESIAN_POINT('Ctrl Pts',(-0.00275827179947781,-0.0131787743898807,
-0.0134666993224125));
#16881=CARTESIAN_POINT('Ctrl Pts',(-0.00269168072014957,-0.0131787743898808,
-0.0135793958120498));
#16882=CARTESIAN_POINT('Ctrl Pts',(-0.0026175373870451,-0.0131787743898809,
-0.0136876390597102));
#16883=CARTESIAN_POINT('Ctrl Pts',(-0.00253649519800816,-0.0131787743898809,
-0.0137908693804752));
#16884=CARTESIAN_POINT('Ctrl Pts',(-0.00252207060914627,-0.013178774389881,
-0.0138092432046871));
#16885=CARTESIAN_POINT('Ctrl Pts',(-0.00250742540379288,-0.013178774389881,
-0.0138274599974619));
#16886=CARTESIAN_POINT('Ctrl Pts',(-0.0024925785367831,-0.013178774389881,
-0.0138454979317755));
#16887=CARTESIAN_POINT('Ctrl Pts',(-0.00235107495916407,-0.013178774389881,
-0.0140174151609494));
#16888=CARTESIAN_POINT('Ctrl Pts',(-0.00219103071556285,-0.013178774389881,
-0.0141735316821853));
#16889=CARTESIAN_POINT('Ctrl Pts',(-0.0020156919207918,-0.013178774389881,
-0.0143109630813275));
#16890=CARTESIAN_POINT('Ctrl Pts',(-0.00200226753649631,-0.013178774389881,
-0.0143214851789543));
#16891=CARTESIAN_POINT('Ctrl Pts',(-0.00198875967272646,-0.013178774389881,
-0.0143318921255368));
#16892=CARTESIAN_POINT('Ctrl Pts',(-0.00197517451207161,-0.013178774389881,
-0.0143421793166972));
#16893=CARTESIAN_POINT('Ctrl Pts',(-0.00170331817561905,-0.0131787743898808,
-0.0145480390906311));
#16894=CARTESIAN_POINT('Ctrl Pts',(-0.00140009528713672,-0.0131787743898807,
-0.0147070178556508));
#16895=CARTESIAN_POINT('Ctrl Pts',(-0.00107703637109689,-0.0131787743898803,
-0.0148072378106216));
#16896=CARTESIAN_POINT('Ctrl Pts',(-0.00105976329426689,-0.0131787743898803,
-0.0148125962975605));
#16897=CARTESIAN_POINT('Ctrl Pts',(-0.00104243331187472,-0.0131787743898803,
-0.0148177848787372));
#16898=CARTESIAN_POINT('Ctrl Pts',(-0.00102504817405061,-0.0131787743898803,
-0.0148228010530932));
#16899=CARTESIAN_POINT('Ctrl Pts',(-0.0010118795244946,-0.0131787743898803,
-0.0148266006342569));
#16900=CARTESIAN_POINT('Ctrl Pts',(-0.000998688467597784,-0.0131787743898803,
-0.0148302986272678));
#16901=CARTESIAN_POINT('Ctrl Pts',(-0.000985476138224112,-0.0131787743898802,
-0.0148338942747791));
#16902=CARTESIAN_POINT('Ctrl Pts',(-0.000895925317347755,-0.0131787743898801,
-0.0148582649347222));
#16903=CARTESIAN_POINT('Ctrl Pts',(-0.00080539262624515,-0.01317877438988,
-0.0148779396012878));
#16904=CARTESIAN_POINT('Ctrl Pts',(-0.000714119979602021,-0.0131787743898799,
-0.0148926845173722));
#16905=CARTESIAN_POINT('Ctrl Pts',(-0.00069085444230266,-0.0131787743898799,
-0.0148964430190455));
#16906=CARTESIAN_POINT('Ctrl Pts',(-0.000667540798596598,-0.0131787743898798,
-0.0148998809501044));
#16907=CARTESIAN_POINT('Ctrl Pts',(-0.000644183020312907,-0.0131787743898798,
-0.0149029938915827));
#16908=CARTESIAN_POINT('Ctrl Pts',(-0.000452732095770299,-0.0131787743898795,
-0.0149285089691225));
#16909=CARTESIAN_POINT('Ctrl Pts',(-0.000258294496493731,-0.0131787743898793,
-0.0149322619746447));
#16910=CARTESIAN_POINT('Ctrl Pts',(-6.4245464843163E-5,-0.0131787743898789,
-0.0149152588842441));
#16911=CARTESIAN_POINT('Ctrl Pts',(-3.38914616751708E-5,-0.0131787743898788,
-0.0149125991860457));
#16912=CARTESIAN_POINT('Ctrl Pts',(-3.54767595355644E-6,-0.0131787743898787,
-0.0149094299724371));
#16913=CARTESIAN_POINT('Ctrl Pts',(2.6772004479569E-5,-0.0131787743898794,
-0.0149057533493354));
#16914=CARTESIAN_POINT('Ctrl Pts',(4.04780385078073E-5,-0.0131787743898798,
-0.0149040913291353));
#16915=CARTESIAN_POINT('Ctrl Pts',(5.41779522435996E-5,-0.0131787743898798,
-0.0149023256959705));
#16916=CARTESIAN_POINT('Ctrl Pts',(6.78581592279457E-5,-0.0131787743898798,
-0.0149004585336354));
#16917=CARTESIAN_POINT('Ctrl Pts',(0.000342411697294035,-0.0131787743898801,
-0.0148629857069577));
#16918=CARTESIAN_POINT('Ctrl Pts',(0.000610525518463131,-0.0131787743898805,
-0.014784763374177));
#16919=CARTESIAN_POINT('Ctrl Pts',(0.000862044456775896,-0.0131787743898807,
-0.0146687404422175));
#16920=CARTESIAN_POINT('Ctrl Pts',(0.000905520526633452,-0.0131787743898807,
-0.0146486854072814));
#16921=CARTESIAN_POINT('Ctrl Pts',(0.000948494845706522,-0.0131787743898808,
-0.0146274928944177));
#16922=CARTESIAN_POINT('Ctrl Pts',(0.000990905948759799,-0.0131787743898808,
-0.0146051688505092));
#16923=CARTESIAN_POINT('Ctrl Pts',(0.00100229353986641,-0.0131787743898808,
-0.0145991747342148));
#16924=CARTESIAN_POINT('Ctrl Pts',(0.00101364138349185,-0.0131787743898808,
-0.0145930985492073));
#16925=CARTESIAN_POINT('Ctrl Pts',(0.0010249455256613,-0.0131787743898808,
-0.0145869418657868));
#16926=CARTESIAN_POINT('Ctrl Pts',(0.00130440311096153,-0.013178774389881,
-0.0144347381995232));
#16927=CARTESIAN_POINT('Ctrl Pts',(0.00155385690165563,-0.013178774389881,
-0.0142359025658652));
#16928=CARTESIAN_POINT('Ctrl Pts',(0.00175560804622792,-0.0131787743898811,
-0.0139933321990506));
#16929=CARTESIAN_POINT('Ctrl Pts',(0.00176494058753933,-0.0131787743898811,
-0.0139821114549303));
#16930=CARTESIAN_POINT('Ctrl Pts',(0.00177416959711849,-0.0131787743898811,
-0.0139707962998009));
#16931=CARTESIAN_POINT('Ctrl Pts',(0.00178329441874934,-0.013178774389881,
-0.0139593884000934));
#16932=CARTESIAN_POINT('Ctrl Pts',(0.00177804161491497,-0.0271768105190238,
-0.0139532084980533));
#16933=CARTESIAN_POINT('Ctrl Pts',(0.00118560412354709,-0.0271237595111731,
-0.0145458929746017));
#16934=CARTESIAN_POINT('Ctrl Pts',(-0.000628566750056487,-0.0270176677375825,
-0.0150813178871608));
#16935=CARTESIAN_POINT('Ctrl Pts',(-0.00278856526638462,-0.0268585351982525,
-0.0132141579990934));
#16936=CARTESIAN_POINT('Ctrl Pts',(-0.00237858331883447,-0.0266994129010339,
-0.0103922510069768));
#16937=CARTESIAN_POINT('Ctrl Pts',(0.00021399493011458,-0.0265402906038154,
-0.0092099097251141));
#16938=CARTESIAN_POINT('Ctrl Pts',(0.00261164118167257,-0.0263811683065968,
-0.010753240507375));
#16939=CARTESIAN_POINT('Ctrl Pts',(0.00260817343599891,-0.0262220460093783,
-0.0136041152219484));
#16940=CARTESIAN_POINT('Ctrl Pts',(0.000208113514731238,-0.0260629237121599,
-0.01514229898489));
#16941=CARTESIAN_POINT('Ctrl Pts',(-0.0023834422823124,-0.0259038014149411,
-0.01395419390056));
#16942=CARTESIAN_POINT('Ctrl Pts',(-0.00278437835194816,-0.0257446791177227,
-0.0111316924551894));
#16943=CARTESIAN_POINT('Ctrl Pts',(-0.000626390273332243,-0.025585556820504,
-0.00926883337176216));
#16944=CARTESIAN_POINT('Ctrl Pts',(0.00210731212168579,-0.0254264345232856,
-0.01007766841686));
#16945=CARTESIAN_POINT('Ctrl Pts',(0.00290427350329033,-0.025267312226067,
-0.0128148422875521));
#16946=CARTESIAN_POINT('Ctrl Pts',(0.00103206954891863,-0.0251081899288485,
-0.014964752376489));
#16947=CARTESIAN_POINT('Ctrl Pts',(-0.00178866211946724,-0.0249490676316299,
-0.0145515245945));
#16948=CARTESIAN_POINT('Ctrl Pts',(-0.00296552147177021,-0.0247899453344113,
-0.0119549353984463));
#16949=CARTESIAN_POINT('Ctrl Pts',(-0.00141691873677219,-0.0246308230371928,
-0.0095613809395787));
#16950=CARTESIAN_POINT('Ctrl Pts',(0.00143390397998829,-0.0244717007399742,
-0.00957065777503687));
#16951=CARTESIAN_POINT('Ctrl Pts',(0.00296689668155396,-0.0243125784427557,
-0.0119742401091903));
#16952=CARTESIAN_POINT('Ctrl Pts',(0.00177316251331238,-0.0241534561455371,
-0.0145631150614389));
#16953=CARTESIAN_POINT('Ctrl Pts',(-0.00105019709697634,-0.0239943338483186,
-0.0149579765952903));
#16954=CARTESIAN_POINT('Ctrl Pts',(-0.0029083728138988,-0.0238352115511001,
-0.0127959271259884));
#16955=CARTESIAN_POINT('Ctrl Pts',(-0.00209360791553675,-0.0236760892538814,
-0.0100639986687876));
#16956=CARTESIAN_POINT('Ctrl Pts',(0.000645287777636742,-0.023516966956663,
-0.00927297063177001));
#16957=CARTESIAN_POINT('Ctrl Pts',(0.00279113160131327,-0.0233578446594443,
-0.0111498374965911));
#16958=CARTESIAN_POINT('Ctrl Pts',(0.00237178535469283,-0.0231987223622259,
-0.0139696643841129));
#16959=CARTESIAN_POINT('Ctrl Pts',(-0.000227350711525737,-0.0230396000650072,
-0.0151408888133467));
#16960=CARTESIAN_POINT('Ctrl Pts',(-0.00261754005891038,-0.0228804777677888,
-0.0135870967313543));
#16961=CARTESIAN_POINT('Ctrl Pts',(-0.00260207867671947,-0.0227213554705702,
-0.0107363010709901));
#16962=CARTESIAN_POINT('Ctrl Pts',(-0.000195176350967375,-0.0225622331733517,
-0.00920852617061793));
#16963=CARTESIAN_POINT('Ctrl Pts',(0.00239110284023198,-0.0224031108761331,
-0.0104078738668982));
#16964=CARTESIAN_POINT('Ctrl Pts',(0.00277983847401713,-0.0222439885789146,
-0.0132320834127006));
#16965=CARTESIAN_POINT('Ctrl Pts',(0.000613762986085649,-0.022084866281696,
-0.0150855644436793));
#16966=CARTESIAN_POINT('Ctrl Pts',(-0.00211639150052274,-0.0219257439844774,
-0.0142648748368236));
#16967=CARTESIAN_POINT('Ctrl Pts',(-0.00290147594298247,-0.0217666216872589,
-0.0115242695442317));
#16968=CARTESIAN_POINT('Ctrl Pts',(-0.00101995832285557,-0.0216074993900403,
-0.00938250242413448));
#16969=CARTESIAN_POINT('Ctrl Pts',(0.00179895220381959,-0.0214483770928218,
-0.00980796498907916));
#16970=CARTESIAN_POINT('Ctrl Pts',(0.00296453533731221,-0.0212892547956032,
-0.0124096357811838));
#16971=CARTESIAN_POINT('Ctrl Pts',(0.00140556165888287,-0.0211301324983847,
-0.0147964487234853));
#16972=CARTESIAN_POINT('Ctrl Pts',(-0.00144519375143724,-0.0209710102011662,
-0.0147748028901041));
#16973=CARTESIAN_POINT('Ctrl Pts',(-0.00296774354704725,-0.0208118879039476,
-0.0123645918886645));
#16974=CARTESIAN_POINT('Ctrl Pts',(-0.00176278802491834,-0.0206527656067291,
-0.00978092063611248));
#16975=CARTESIAN_POINT('Ctrl Pts',(0.00106225819433125,-0.0204936433095104,
-0.00939831272888084));
#16976=CARTESIAN_POINT('Ctrl Pts',(0.00291103580144525,-0.020334521012292,
-0.0115684040428596));
#16977=CARTESIAN_POINT('Ctrl Pts',(0.00208442535608753,-0.0201753987150733,
-0.0142967717092857));
#16978=CARTESIAN_POINT('Ctrl Pts',(-0.00065787664180178,-0.0200162764178549,
-0.0150759088627734));
#16979=CARTESIAN_POINT('Ctrl Pts',(-0.00279555697663806,-0.0198571541206363,
-0.0131897493420468));
#16980=CARTESIAN_POINT('Ctrl Pts',(-0.0023639800967097,-0.0196980318234177,
-0.010371768442842));
#16981=CARTESIAN_POINT('Ctrl Pts',(0.000240213177657409,-0.0195389095261993,
-0.00921183209057361));
#16982=CARTESIAN_POINT('Ctrl Pts',(0.00262363848165746,-0.0193797872289806,
-0.0107759800285337));
#16983=CARTESIAN_POINT('Ctrl Pts',(0.0025958082990893,-0.0192206649317622,
-0.013626681772405));
#16984=CARTESIAN_POINT('Ctrl Pts',(0.000182299964970184,-0.0190615426345435,
-0.0151439992977471));
#16985=CARTESIAN_POINT('Ctrl Pts',(-0.00239875118947593,-0.018902420337325,
-0.013933441620598));
#16986=CARTESIAN_POINT('Ctrl Pts',(-0.00277522956952002,-0.0187432980401064,
-0.0111075720233));
#16987=CARTESIAN_POINT('Ctrl Pts',(-0.000601132642494807,-0.018584175742888,
-0.00926350654087479));
#16988=CARTESIAN_POINT('Ctrl Pts',(0.00212543536334061,-0.0184250534456693,
-0.0100960339344926));
#16989=CARTESIAN_POINT('Ctrl Pts',(0.00289862156103897,-0.0182659311484509,
-0.0128400197316981));
#16990=CARTESIAN_POINT('Ctrl Pts',(0.00100782901646378,-0.0181068088512323,
-0.0149736032207967));
#16991=CARTESIAN_POINT('Ctrl Pts',(-0.0018092089931206,-0.0179476865540137,
-0.0145359140569992));
#16992=CARTESIAN_POINT('Ctrl Pts',(-0.00296349310521268,-0.0177885642567952,
-0.0119292105563712));
#16993=CARTESIAN_POINT('Ctrl Pts',(-0.00139417826899081,-0.0176294419595766,
-0.00954918410769673));
#16994=CARTESIAN_POINT('Ctrl Pts',(0.00145645639226353,-0.0174703196623581,
-0.00958319850845797));
#16995=CARTESIAN_POINT('Ctrl Pts',(0.00296853450650743,-0.0173111973651395,
-0.0119999928166982));
#16996=CARTESIAN_POINT('Ctrl Pts',(0.0017523803714217,-0.017152075067921,
-0.0145784117258758));
#16997=CARTESIAN_POINT('Ctrl Pts',(-0.00107429930442917,-0.0169929527707024,
-0.014948758807064));
#16998=CARTESIAN_POINT('Ctrl Pts',(-0.00291364398395591,-0.0168338304734839,
-0.0127706664985865));
#16999=CARTESIAN_POINT('Ctrl Pts',(-0.00207520355930568,-0.0166747081762654,
-0.0100459109858006));
#17000=CARTESIAN_POINT('Ctrl Pts',(0.000670453121618061,-0.0165155858790467,
-0.00927867938167256));
#17001=CARTESIAN_POINT('Ctrl Pts',(0.00279992972710902,-0.0163564635818283,
-0.0111740960535678));
#17002=CARTESIAN_POINT('Ctrl Pts',(0.00235613033278755,-0.0161973412846097,
-0.013990177911836));
#17003=CARTESIAN_POINT('Ctrl Pts',(-0.000253071113445288,-0.0160382189873912,
-0.0151388043592267));
#17004=CARTESIAN_POINT('Ctrl Pts',(-0.00262968753099502,-0.0158790966901726,
-0.0135643299949519));
#17005=CARTESIAN_POINT('Ctrl Pts',(-0.00258948902257005,-0.015719974392954,
-0.0107137758623792));
#17006=CARTESIAN_POINT('Ctrl Pts',(-0.000169420211623477,-0.0155608520957355,
-0.00920694421604582));
#17007=CARTESIAN_POINT('Ctrl Pts',(0.00240635450886322,-0.0154017297985169,
-0.0104286892022747));
#17008=CARTESIAN_POINT('Ctrl Pts',(0.00277056817242066,-0.0152426075012984,
-0.0132561654242236));
#17009=CARTESIAN_POINT('Ctrl Pts',(0.000588491471565203,-0.0150834852040798,
-0.0150907810950793));
#17010=CARTESIAN_POINT('Ctrl Pts',(-0.00213444017556847,-0.0149243629068613,
-0.0142464306998757));
#17011=CARTESIAN_POINT('Ctrl Pts',(-0.00289571072485587,-0.0147652406096428,
-0.0114991177966801));
#17012=CARTESIAN_POINT('Ctrl Pts',(-0.000995684446481558,-0.0146061183124242,
-0.0093737546786092));
#17013=CARTESIAN_POINT('Ctrl Pts',(0.00181943901096383,-0.0144469960152056,
-0.00982366893049069));
#17014=CARTESIAN_POINT('Ctrl Pts',(0.00296238076824064,-0.0142878737179871,
-0.012435342848044));
#17015=CARTESIAN_POINT('Ctrl Pts',(0.00138279676337737,-0.0141287514207685,
-0.0148085639739896));
#17016=CARTESIAN_POINT('Ctrl Pts',(-0.00146774688362298,-0.01396962912355,
-0.0147621306115525));
#17017=CARTESIAN_POINT('Ctrl Pts',(-0.00296916099271162,-0.0138105068263315,
-0.0123388987639402));
#17018=CARTESIAN_POINT('Ctrl Pts',(-0.00174215309885327,-0.0136513845291129,
-0.00976558372456728));
#17019=CARTESIAN_POINT('Ctrl Pts',(0.00108673957578367,-0.0134922622318943,
-0.00940789155737695));
#17020=CARTESIAN_POINT('Ctrl Pts',(0.00291537148706041,-0.0133331399346758,
-0.0115931828919089));
#17021=CARTESIAN_POINT('Ctrl Pts',(0.00206758582828193,-0.0131740176374573,
-0.0143157742579136));
#17022=CARTESIAN_POINT('Ctrl Pts',(-0.000686797985030798,-0.0130148766356141,
-0.0150681813871851));
#17023=CARTESIAN_POINT('Ctrl Pts',(-0.00209243490244101,-0.0129087763995103,
-0.0138021198294159));
#17024=CARTESIAN_POINT('Ctrl Pts',(-0.00237105117954937,-0.0128557169291459,
-0.0130116402165948));
#17025=CARTESIAN_POINT('Ctrl Pts',(0.0019117872489877,-0.0272859922955674,
-0.0140869025003421));
#17026=CARTESIAN_POINT('Ctrl Pts',(0.00127478616176987,-0.0272329412877163,
-0.0147241691511522));
#17027=CARTESIAN_POINT('Ctrl Pts',(-0.000675848016050572,-0.0271268495141259,
-0.0152998691302945));
#17028=CARTESIAN_POINT('Ctrl Pts',(-0.00299832325324907,-0.0269677169747958,
-0.0132922600642947));
#17029=CARTESIAN_POINT('Ctrl Pts',(-0.00255750215375024,-0.0268085946775773,
-0.0102580870955053));
#17030=CARTESIAN_POINT('Ctrl Pts',(0.000230091790489749,-0.0266494723803588,
-0.00898680920883726));
#17031=CARTESIAN_POINT('Ctrl Pts',(0.00280809080517024,-0.0264903500831402,
-0.01064623049895));
#17032=CARTESIAN_POINT('Ctrl Pts',(0.00280436221304618,-0.0263312277859216,
-0.0137115501641726));
#17033=CARTESIAN_POINT('Ctrl Pts',(0.000223767970596245,-0.0261721054887031,
-0.0153654372722831));
#17034=CARTESIAN_POINT('Ctrl Pts',(-0.00256272661213327,-0.0260129831914847,
-0.01408796202557));
#17035=CARTESIAN_POINT('Ctrl Pts',(-0.00299382139594434,-0.0258538608942659,
-0.0110531498883035));
#17036=CARTESIAN_POINT('Ctrl Pts',(-0.0006735078231022,-0.0256947385970475,
-0.00905016513671916));
#17037=CARTESIAN_POINT('Ctrl Pts',(0.00226582573213212,-0.025535616299829,
-0.00991984136520626));
#17038=CARTESIAN_POINT('Ctrl Pts',(0.0031227351511842,-0.0253764940026104,
-0.0128629075231386));
#17039=CARTESIAN_POINT('Ctrl Pts',(0.00110970260040032,-0.0252173717053917,
-0.0151745354738127));
#17040=CARTESIAN_POINT('Ctrl Pts',(-0.0019232066359191,-0.0250582494081734,
-0.0147302243857556));
#17041=CARTESIAN_POINT('Ctrl Pts',(-0.0031885902381428,-0.0248991271109547,
-0.0119383177879384));
#17042=CARTESIAN_POINT('Ctrl Pts',(-0.0015235004350235,-0.0247400048137363,
-0.00936471835368694));
#17043=CARTESIAN_POINT('Ctrl Pts',(0.00154176332107131,-0.0245808825165175,
-0.00937469299971953));
#17044=CARTESIAN_POINT('Ctrl Pts',(0.00319006889224584,-0.0244217602192992,
-0.0119590746136147));
#17045=CARTESIAN_POINT('Ctrl Pts',(0.00190654113767505,-0.0242626379220806,
-0.0147426866963774));
#17046=CARTESIAN_POINT('Ctrl Pts',(-0.00112919371632327,-0.0241035156248619,
-0.0151672500132313));
#17047=CARTESIAN_POINT('Ctrl Pts',(-0.0031271428150348,-0.0239443933276435,
-0.0128425695488265));
#17048=CARTESIAN_POINT('Ctrl Pts',(-0.00225109068523927,-0.0237852710304249,
-0.00990514336835257));
#17049=CARTESIAN_POINT('Ctrl Pts',(0.000693826811962741,-0.0236261487332063,
-0.00905461360455169));
#17050=CARTESIAN_POINT('Ctrl Pts',(0.00300108262983063,-0.0234670264359878,
-0.0110726598134331));
#17051=CARTESIAN_POINT('Ctrl Pts',(0.00255019284160814,-0.0233079041387693,
-0.014104596210588));
#17052=CARTESIAN_POINT('Ctrl Pts',(-0.000244452203872613,-0.0231487818415506,
-0.0153639210265705));
#17053=CARTESIAN_POINT('Ctrl Pts',(-0.00281443340041212,-0.0229896595443322,
-0.013693251529854));
#17054=CARTESIAN_POINT('Ctrl Pts',(-0.00279780900136746,-0.0228305372471135,
-0.0106280168653581));
#17055=CARTESIAN_POINT('Ctrl Pts',(-0.000209857663596484,-0.022671414949895,
-0.00898532158232617));
#17056=CARTESIAN_POINT('Ctrl Pts',(0.00257096340300922,-0.0225122926526765,
-0.0102748851187573));
#17057=CARTESIAN_POINT('Ctrl Pts',(0.00298894002496421,-0.0223531703554579,
-0.0133115338410611));
#17058=CARTESIAN_POINT('Ctrl Pts',(0.000659930701765533,-0.0221940480582394,
-0.0153044351160038));
#17059=CARTESIAN_POINT('Ctrl Pts',(-0.00227558806870716,-0.0220349257610208,
-0.0144220126166641));
#17060=CARTESIAN_POINT('Ctrl Pts',(-0.00311972715627565,-0.0218758034638022,
-0.0114752569226835));
#17061=CARTESIAN_POINT('Ctrl Pts',(-0.00109668035875944,-0.0217166811665838,
-0.00917238446111915));
#17062=CARTESIAN_POINT('Ctrl Pts',(0.00193427074819341,-0.0215575588693652,
-0.00962985064175281));
#17063=CARTESIAN_POINT('Ctrl Pts',(0.00318752992590557,-0.0213984365721466,
-0.0124272210771164));
#17064=CARTESIAN_POINT('Ctrl Pts',(0.00151128906915194,-0.021239314274928,
-0.0149935718928306));
#17065=CARTESIAN_POINT('Ctrl Pts',(-0.00155390231766119,-0.0210801919777095,
-0.0149702978435032));
#17066=CARTESIAN_POINT('Ctrl Pts',(-0.00319097945960156,-0.020921069680491,
-0.0123787889489587));
#17067=CARTESIAN_POINT('Ctrl Pts',(-0.00189538627242324,-0.0207619473832725,
-0.00960077199211658));
#17068=CARTESIAN_POINT('Ctrl Pts',(0.00114216205853669,-0.0206028250860538,
-0.00918938402893757));
#17069=CARTESIAN_POINT('Ctrl Pts',(0.00313000611451711,-0.0204437027888353,
-0.0115227112516539));
#17070=CARTESIAN_POINT('Ctrl Pts',(0.00224121740672834,-0.0202845804916167,
-0.0144563087959796));
#17071=CARTESIAN_POINT('Ctrl Pts',(-0.000707362620004616,-0.0201254581943983,
-0.0152940532350047));
#17072=CARTESIAN_POINT('Ctrl Pts',(-0.00300584088523195,-0.0199663358971797,
-0.0132660153696177));
#17073=CARTESIAN_POINT('Ctrl Pts',(-0.0025418004662205,-0.0198072135999612,
-0.010236063817416));
#17074=CARTESIAN_POINT('Ctrl Pts',(0.000258282194427836,-0.0196480913027426,
-0.00898887617607948));
#17075=CARTESIAN_POINT('Ctrl Pts',(0.00282099055112725,-0.0194889690055241,
-0.0106706805040763));
#17076=CARTESIAN_POINT('Ctrl Pts',(0.00279106696119298,-0.0193298467083055,
-0.0137358141876099));
#17077=CARTESIAN_POINT('Ctrl Pts',(0.000196012706112937,-0.019170724411087,
-0.0153672654839583));
#17078=CARTESIAN_POINT('Ctrl Pts',(-0.00257918706686371,-0.0190116021138684,
-0.0140656487434252));
#17079=CARTESIAN_POINT('Ctrl Pts',(-0.00298398443518755,-0.0188524798166499,
-0.0110272150992978));
#17080=CARTESIAN_POINT('Ctrl Pts',(-0.000646350294184092,-0.0186933575194313,
-0.00904443761758662));
#17081=CARTESIAN_POINT('Ctrl Pts',(0.00228531221772131,-0.0185342352222128,
-0.00993958835095536));
#17082=CARTESIAN_POINT('Ctrl Pts',(0.0031166580655651,-0.0183751129249941,
-0.0128899788336617));
#17083=CARTESIAN_POINT('Ctrl Pts',(0.00108363867677383,-0.0182159906277757,
-0.0151840520853187));
#17084=CARTESIAN_POINT('Ctrl Pts',(-0.00194529906093746,-0.0180568683305571,
-0.014713439611826));
#17085=CARTESIAN_POINT('Ctrl Pts',(-0.00318640929631981,-0.0178977460333385,
-0.0119106579038002));
#17086=CARTESIAN_POINT('Ctrl Pts',(-0.00149904941206893,-0.0177386237361201,
-0.00935160406689274));
#17087=CARTESIAN_POINT('Ctrl Pts',(0.00156601214284244,-0.0175795014389015,
-0.00938817705658642));
#17088=CARTESIAN_POINT('Ctrl Pts',(0.00319182991563014,-0.0174203791416829,
-0.0119867644592445));
#17089=CARTESIAN_POINT('Ctrl Pts',(0.00188419574736476,-0.0172612568444644,
-0.0147591339874741));
#17090=CARTESIAN_POINT('Ctrl Pts',(-0.00115510891003655,-0.0171021345472458,
-0.0151573388560083));
#17091=CARTESIAN_POINT('Ctrl Pts',(-0.00313281048648741,-0.0169430122500273,
-0.0128154087979401));
#17092=CARTESIAN_POINT('Ctrl Pts',(-0.00223130193942295,-0.0167838899528087,
-0.00988569511618116));
#17093=CARTESIAN_POINT('Ctrl Pts',(0.000720885112137661,-0.0166247676555902,
-0.00906075177093641));
#17094=CARTESIAN_POINT('Ctrl Pts',(0.00301054255729814,-0.0164656453583716,
-0.0110987431173996));
#17095=CARTESIAN_POINT('Ctrl Pts',(0.00253336023712347,-0.0163065230611531,
-0.0141266527813699));
#17096=CARTESIAN_POINT('Ctrl Pts',(-0.000272107313863377,-0.0161474007639344,
-0.0153616797782363));
#17097=CARTESIAN_POINT('Ctrl Pts',(-0.00282749461452771,-0.015988278466716,
-0.0136687722623329));
#17098=CARTESIAN_POINT('Ctrl Pts',(-0.002784272343918,-0.0158291561694974,
-0.0106037972935313));
#17099=CARTESIAN_POINT('Ctrl Pts',(-0.000182164127985299,-0.0156700338722789,
-0.00898362063193561));
#17100=CARTESIAN_POINT('Ctrl Pts',(0.00258736231368171,-0.0155109115750603,
-0.0102972661993925));
#17101=CARTESIAN_POINT('Ctrl Pts',(0.00297897240427542,-0.0153517892778418,
-0.0133374273196913));
#17102=CARTESIAN_POINT('Ctrl Pts',(0.000632758244823287,-0.0151926669806233,
-0.0153100441678648));
#17103=CARTESIAN_POINT('Ctrl Pts',(-0.00229499437873055,-0.0150335446834047,
-0.0144021810977954));
#17104=CARTESIAN_POINT('Ctrl Pts',(-0.00311352827408435,-0.0148744223861861,
-0.011448213241672));
#17105=CARTESIAN_POINT('Ctrl Pts',(-0.00107058058305899,-0.0147153000889676,
-0.00916297870356417));
#17106=CARTESIAN_POINT('Ctrl Pts',(0.00195629858845448,-0.014556177791749,
-0.00964673584550599));
#17107=CARTESIAN_POINT('Ctrl Pts',(0.00318521328852005,-0.0143970554945306,
-0.0124548618489747));
#17108=CARTESIAN_POINT('Ctrl Pts',(0.00148681178100139,-0.0142379331973119,
-0.0150065984616343));
#17109=CARTESIAN_POINT('Ctrl Pts',(-0.00157815191349504,-0.0140788109000934,
-0.0149566723465815));
#17110=CARTESIAN_POINT('Ctrl Pts',(-0.00319250352660007,-0.0139196886028748,
-0.0123511631679746));
#17111=CARTESIAN_POINT('Ctrl Pts',(-0.0018731991716242,-0.0137605663056563,
-0.00958428142649361));
#17112=CARTESIAN_POINT('Ctrl Pts',(0.00116848494800438,-0.0136014440084377,
-0.00919968338415261));
#17113=CARTESIAN_POINT('Ctrl Pts',(0.00313466793368104,-0.0134423217112193,
-0.011549353984456));
#17114=CARTESIAN_POINT('Ctrl Pts',(0.0022231111969143,-0.0132831994140006,
-0.0144767407306771));
#17115=CARTESIAN_POINT('Ctrl Pts',(-0.000738459448529337,-0.0131240584121574,
-0.0152857444928626));
#17116=CARTESIAN_POINT('Ctrl Pts',(-0.00224982943721194,-0.0130179581760535,
-0.0139244488278607));
#17117=CARTESIAN_POINT('Ctrl Pts',(-0.00254940344125551,-0.0129648987056893,
-0.0130745087411389));
#17118=CARTESIAN_POINT('Ctrl Pts',(0.00204553288306044,-0.0273951740721106,
-0.0142205965026308));
#17119=CARTESIAN_POINT('Ctrl Pts',(0.00136396819999266,-0.0273421230642597,
-0.0149024453277029));
#17120=CARTESIAN_POINT('Ctrl Pts',(-0.000723129282044651,-0.0272360312906692,
-0.0155184203734285));
#17121=CARTESIAN_POINT('Ctrl Pts',(-0.00320808124011354,-0.0270768987513391,
-0.013370362129496));
#17122=CARTESIAN_POINT('Ctrl Pts',(-0.00273642098866601,-0.0269177764541206,
-0.0101239231840337));
#17123=CARTESIAN_POINT('Ctrl Pts',(0.000246188650864915,-0.026758654156902,
-0.00876370869256043));
#17124=CARTESIAN_POINT('Ctrl Pts',(0.00300454042866792,-0.0265995318596834,
-0.0105392204905252));
#17125=CARTESIAN_POINT('Ctrl Pts',(0.00300055099009345,-0.026440409562465,
-0.0138189851063969));
#17126=CARTESIAN_POINT('Ctrl Pts',(0.000239422426461252,-0.0262812872652464,
-0.0155885755596761));
#17127=CARTESIAN_POINT('Ctrl Pts',(-0.00274201094195411,-0.0261221649680278,
-0.01422173015058));
#17128=CARTESIAN_POINT('Ctrl Pts',(-0.00320326443994053,-0.0259630426708093,
-0.0109746073214176));
#17129=CARTESIAN_POINT('Ctrl Pts',(-0.000720625372872156,-0.0258039203735906,
-0.00883149690167625));
#17130=CARTESIAN_POINT('Ctrl Pts',(0.00242433934257846,-0.0256447980763722,
-0.0097620143135525));
#17131=CARTESIAN_POINT('Ctrl Pts',(0.00334119679907805,-0.0254856757791536,
-0.012910972758725));
#17132=CARTESIAN_POINT('Ctrl Pts',(0.001187335651882,-0.0253265534819351,
-0.0153843185711368));
#17133=CARTESIAN_POINT('Ctrl Pts',(-0.00205775115237095,-0.0251674311847165,
-0.0149089241770113));
#17134=CARTESIAN_POINT('Ctrl Pts',(-0.00341165900451537,-0.025008308887498,
-0.0119217001774306));
#17135=CARTESIAN_POINT('Ctrl Pts',(-0.00163008213327481,-0.0248491865902795,
-0.00916805576779518));
#17136=CARTESIAN_POINT('Ctrl Pts',(0.00164962266215434,-0.0246900642930608,
-0.0091787282244021));
#17137=CARTESIAN_POINT('Ctrl Pts',(0.00341324110293771,-0.0245309419958423,
-0.011943909118039));
#17138=CARTESIAN_POINT('Ctrl Pts',(0.00203991976203773,-0.0243718196986238,
-0.014922258331316));
#17139=CARTESIAN_POINT('Ctrl Pts',(-0.00120819033567019,-0.0242126974014052,
-0.0153765234311726));
#17140=CARTESIAN_POINT('Ctrl Pts',(-0.00334591281617079,-0.0240535751041867,
-0.0128892119716646));
#17141=CARTESIAN_POINT('Ctrl Pts',(-0.00240857345494178,-0.0238944528069681,
-0.00974628806791765));
#17142=CARTESIAN_POINT('Ctrl Pts',(0.000742365846288737,-0.0237353305097496,
-0.00883625657733327));
#17143=CARTESIAN_POINT('Ctrl Pts',(0.003211033658348,-0.023576208212531,
-0.0109954821302748));
#17144=CARTESIAN_POINT('Ctrl Pts',(0.00272860032852343,-0.0234170859153125,
-0.0142395280370631));
#17145=CARTESIAN_POINT('Ctrl Pts',(-0.000261553696219489,-0.0232579636180939,
-0.0155869532397943));
#17146=CARTESIAN_POINT('Ctrl Pts',(-0.00301132674191384,-0.0230988413208754,
-0.0137994063283536));
#17147=CARTESIAN_POINT('Ctrl Pts',(-0.00299353932601547,-0.0229397190236568,
-0.0105197326597259));
#17148=CARTESIAN_POINT('Ctrl Pts',(-0.000224538976225593,-0.0227805967264383,
-0.00876211699403452));
#17149=CARTESIAN_POINT('Ctrl Pts',(0.00275082396578644,-0.0226214744292197,
-0.0101418963706166));
#17150=CARTESIAN_POINT('Ctrl Pts',(0.0031980415759113,-0.0224623521320012,
-0.0133909842694217));
#17151=CARTESIAN_POINT('Ctrl Pts',(0.000706098417445418,-0.0223032298347826,
-0.0155233057883285));
#17152=CARTESIAN_POINT('Ctrl Pts',(-0.00243478463689158,-0.0221441075375641,
-0.0145791503965046));
#17153=CARTESIAN_POINT('Ctrl Pts',(-0.00333797836956883,-0.0219849852403455,
-0.011426244301135));
#17154=CARTESIAN_POINT('Ctrl Pts',(-0.0011734023946633,-0.021825862943127,
-0.00896226649810381));
#17155=CARTESIAN_POINT('Ctrl Pts',(0.00206958929256724,-0.0216667406459084,
-0.00945173629442646));
#17156=CARTESIAN_POINT('Ctrl Pts',(0.00341052451449892,-0.0215076183486899,
-0.0124448063730491));
#17157=CARTESIAN_POINT('Ctrl Pts',(0.00161701647942103,-0.0213484960514714,
-0.015190695062176));
#17158=CARTESIAN_POINT('Ctrl Pts',(-0.00166261088388514,-0.0211893737542528,
-0.0151657927969023));
#17159=CARTESIAN_POINT('Ctrl Pts',(-0.00341421537215588,-0.0210302514570342,
-0.0123929860092532));
#17160=CARTESIAN_POINT('Ctrl Pts',(-0.00202798451992814,-0.0208711291598156,
-0.00942062334812066));
#17161=CARTESIAN_POINT('Ctrl Pts',(0.00122206592274213,-0.0207120068625972,
-0.0089804553289943));
#17162=CARTESIAN_POINT('Ctrl Pts',(0.00334897642758895,-0.0205528845653786,
-0.0114770184604482));
#17163=CARTESIAN_POINT('Ctrl Pts',(0.00239800945736913,-0.02039376226816,
-0.0146158458826736));
#17164=CARTESIAN_POINT('Ctrl Pts',(-0.000756848598207453,-0.0202346399709415,
-0.0155121976072364));
#17165=CARTESIAN_POINT('Ctrl Pts',(-0.00321612479382583,-0.0200755176737229,
-0.0133422813971887));
#17166=CARTESIAN_POINT('Ctrl Pts',(-0.00271962083573129,-0.0199163953765044,
-0.01010035919199));
#17167=CARTESIAN_POINT('Ctrl Pts',(0.000276351211198263,-0.0197572730792858,
-0.00876592026158535));
#17168=CARTESIAN_POINT('Ctrl Pts',(0.00301834262059706,-0.0195981507820673,
-0.0105653809796189));
#17169=CARTESIAN_POINT('Ctrl Pts',(0.00298632562329664,-0.0194390284848487,
-0.0138449466028145));
#17170=CARTESIAN_POINT('Ctrl Pts',(0.000209725447255692,-0.0192799061876302,
-0.0155905316701697));
#17171=CARTESIAN_POINT('Ctrl Pts',(-0.00275962294425149,-0.0191207838904117,
-0.0141978558662525));
#17172=CARTESIAN_POINT('Ctrl Pts',(-0.00319273930085507,-0.018961661593193,
-0.0109468581752957));
#17173=CARTESIAN_POINT('Ctrl Pts',(-0.000691567945873381,-0.0188025392959746,
-0.00882536869429835));
#17174=CARTESIAN_POINT('Ctrl Pts',(0.00244518907210201,-0.018643416998756,
-0.00978314276741825));
#17175=CARTESIAN_POINT('Ctrl Pts',(0.00333469457009122,-0.0184842947015375,
-0.0129399379356254));
#17176=CARTESIAN_POINT('Ctrl Pts',(0.00115944833708388,-0.0183251724043189,
-0.0153945009498407));
#17177=CARTESIAN_POINT('Ctrl Pts',(-0.00208138912875434,-0.0181660501071004,
-0.0148909651666526));
#17178=CARTESIAN_POINT('Ctrl Pts',(-0.00340932548742695,-0.0180069278098818,
-0.0118921052512293));
#17179=CARTESIAN_POINT('Ctrl Pts',(-0.00160392055514706,-0.0178478055126632,
-0.00915402402608875));
#17180=CARTESIAN_POINT('Ctrl Pts',(0.00167556789342136,-0.0176886832154447,
-0.00919315560471498));
#17181=CARTESIAN_POINT('Ctrl Pts',(0.00341512532475283,-0.0175295609182261,
-0.0119735361017907));
#17182=CARTESIAN_POINT('Ctrl Pts',(0.00201601112330781,-0.0173704386210076,
-0.0149398562490724));
#17183=CARTESIAN_POINT('Ctrl Pts',(-0.00123591851564392,-0.0172113163237891,
-0.0153659189049525));
#17184=CARTESIAN_POINT('Ctrl Pts',(-0.0033519769890189,-0.0170521940265705,
-0.0128601510972937));
#17185=CARTESIAN_POINT('Ctrl Pts',(-0.00238740031954021,-0.016893071729352,
-0.00972547924656174));
#17186=CARTESIAN_POINT('Ctrl Pts',(0.000771317102657261,-0.0167339494321333,
-0.00884282416020026));
#17187=CARTESIAN_POINT('Ctrl Pts',(0.00322115538748726,-0.0165748271349149,
-0.0110233901812313));
#17188=CARTESIAN_POINT('Ctrl Pts',(0.00271059014145939,-0.0164157048376963,
-0.0142631276509039));
#17189=CARTESIAN_POINT('Ctrl Pts',(-0.000291143514281472,-0.0162565825404778,
-0.0155845551972457));
#17190=CARTESIAN_POINT('Ctrl Pts',(-0.00302530169806039,-0.0160974602432592,
-0.0137732145297137));
#17191=CARTESIAN_POINT('Ctrl Pts',(-0.00297905566526595,-0.0159383379460406,
-0.0104938187246836));
#17192=CARTESIAN_POINT('Ctrl Pts',(-0.000194908044347123,-0.0157792156488221,
-0.0087602970478254));
#17193=CARTESIAN_POINT('Ctrl Pts',(0.0027683701185002,-0.0156200933516036,
-0.0101658431965103));
#17194=CARTESIAN_POINT('Ctrl Pts',(0.00318737663613016,-0.015460971054385,
-0.0134186892151591));
#17195=CARTESIAN_POINT('Ctrl Pts',(0.000677025018081376,-0.0153018487571665,
-0.0155293072406504));
#17196=CARTESIAN_POINT('Ctrl Pts',(-0.00245554858189265,-0.0151427264599479,
-0.0145579314957151));
#17197=CARTESIAN_POINT('Ctrl Pts',(-0.00333134582331285,-0.0149836041627294,
-0.0113973086866639));
#17198=CARTESIAN_POINT('Ctrl Pts',(-0.00114547671963643,-0.0148244818655108,
-0.00895220272851903));
#17199=CARTESIAN_POINT('Ctrl Pts',(0.00209315816594511,-0.0146653595682923,
-0.00946980276052119));
#17200=CARTESIAN_POINT('Ctrl Pts',(0.00340804580879949,-0.0145062372710737,
-0.0124743808499052));
#17201=CARTESIAN_POINT('Ctrl Pts',(0.00159082679862542,-0.0143471149738551,
-0.015204632949279));
#17202=CARTESIAN_POINT('Ctrl Pts',(-0.00168855694336709,-0.0141879926766366,
-0.0151512140816105));
#17203=CARTESIAN_POINT('Ctrl Pts',(-0.00341584606048853,-0.0140288703794181,
-0.0123634275720089));
#17204=CARTESIAN_POINT('Ctrl Pts',(-0.00200424524439513,-0.0138697480821995,
-0.00940297912842001));
#17205=CARTESIAN_POINT('Ctrl Pts',(0.00125023032022508,-0.0137106257849809,
-0.00899147521092818));
#17206=CARTESIAN_POINT('Ctrl Pts',(0.00335396438030165,-0.0135515034877625,
-0.0115055250770028));
#17207=CARTESIAN_POINT('Ctrl Pts',(0.00237863656554669,-0.0133923811905438,
-0.0146377072034405));
#17208=CARTESIAN_POINT('Ctrl Pts',(-0.000790120912027881,-0.0132332401887006,
-0.0155033075985401));
#17209=CARTESIAN_POINT('Ctrl Pts',(-0.00240722397198286,-0.0131271399525968,
-0.0140467778263056));
#17210=CARTESIAN_POINT('Ctrl Pts',(-0.00272775570296166,-0.0130740804822326,
-0.0131373772656828));
#17211=CARTESIAN_POINT('Ctrl Pts',(0.00217927851713317,-0.0275043558486539,
-0.0143542905049196));
#17212=CARTESIAN_POINT('Ctrl Pts',(0.00145315023821544,-0.0274513048408029,
-0.0150807215042535));
#17213=CARTESIAN_POINT('Ctrl Pts',(-0.000770410548038733,-0.0273452130672124,
-0.0157369716165624));
#17214=CARTESIAN_POINT('Ctrl Pts',(-0.00341783922697799,-0.0271860805278823,
-0.0134484641946973));
#17215=CARTESIAN_POINT('Ctrl Pts',(-0.00291533982358178,-0.0270269582306638,
-0.00998975927256213));
#17216=CARTESIAN_POINT('Ctrl Pts',(0.000262285511240084,-0.0268678359334452,
-0.00854060817628358));
#17217=CARTESIAN_POINT('Ctrl Pts',(0.00320099005216559,-0.0267087136362267,
-0.0104322104821004));
#17218=CARTESIAN_POINT('Ctrl Pts',(0.00319673976714072,-0.0265495913390081,
-0.0139264200486212));
#17219=CARTESIAN_POINT('Ctrl Pts',(0.000255076882326259,-0.0263904690417896,
-0.0158117138470693));
#17220=CARTESIAN_POINT('Ctrl Pts',(-0.00292129527177496,-0.026231346744571,
-0.0143554982755902));
#17221=CARTESIAN_POINT('Ctrl Pts',(-0.00341270748393672,-0.0260722244473525,
-0.0108960647545318));
#17222=CARTESIAN_POINT('Ctrl Pts',(-0.000767742922642114,-0.0259131021501339,
-0.00861282866663324));
#17223=CARTESIAN_POINT('Ctrl Pts',(0.00258285295302481,-0.0257539798529154,
-0.00960418726189884));
#17224=CARTESIAN_POINT('Ctrl Pts',(0.00355965844697192,-0.0255948575556968,
-0.0129590379943115));
#17225=CARTESIAN_POINT('Ctrl Pts',(0.00126496870336369,-0.0254357352584783,
-0.0155941016684606));
#17226=CARTESIAN_POINT('Ctrl Pts',(-0.00219229566882281,-0.0252766129612597,
-0.0150876239682666));
#17227=CARTESIAN_POINT('Ctrl Pts',(-0.00363472777088795,-0.0251174906640412,
-0.0119050825669227));
#17228=CARTESIAN_POINT('Ctrl Pts',(-0.00173666383152611,-0.0249583683668226,
-0.00897139318190331));
#17229=CARTESIAN_POINT('Ctrl Pts',(0.00175748200323739,-0.0247992460696041,
-0.00898276344908466));
#17230=CARTESIAN_POINT('Ctrl Pts',(0.00363641331362957,-0.0246401237723855,
-0.0119287436224631));
#17231=CARTESIAN_POINT('Ctrl Pts',(0.00217329838640041,-0.024481001475167,
-0.0151018299662544));
#17232=CARTESIAN_POINT('Ctrl Pts',(-0.00128718695501713,-0.0243218791779484,
-0.0155857968491138));
#17233=CARTESIAN_POINT('Ctrl Pts',(-0.00356468281730678,-0.0241627568807299,
-0.0129358543945025));
#17234=CARTESIAN_POINT('Ctrl Pts',(-0.00256605622464431,-0.0240036345835113,
-0.00958743276748271));
#17235=CARTESIAN_POINT('Ctrl Pts',(0.000790904880614737,-0.0238445122862928,
-0.00861789955011497));
#17236=CARTESIAN_POINT('Ctrl Pts',(0.00342098468686536,-0.0236853899890742,
-0.0109183044471168));
#17237=CARTESIAN_POINT('Ctrl Pts',(0.00290700781543874,-0.0235262676918557,
-0.0143744598635381));
#17238=CARTESIAN_POINT('Ctrl Pts',(-0.000278655188566368,-0.0233671453946371,
-0.0158099854530181));
#17239=CARTESIAN_POINT('Ctrl Pts',(-0.00320822008341556,-0.0232080230974186,
-0.0139055611268533));
#17240=CARTESIAN_POINT('Ctrl Pts',(-0.00318926965066348,-0.0230489008002001,
-0.0104114484540937));
#17241=CARTESIAN_POINT('Ctrl Pts',(-0.000239220288854699,-0.0228897785029815,
-0.00853891240574276));
#17242=CARTESIAN_POINT('Ctrl Pts',(0.00293068452856366,-0.022730656205763,
-0.0100089076224755));
#17243=CARTESIAN_POINT('Ctrl Pts',(0.00340714312685838,-0.0225715339085444,
-0.0134704346977821));
#17244=CARTESIAN_POINT('Ctrl Pts',(0.000752266133125304,-0.0224124116113258,
-0.0157421764606531));
#17245=CARTESIAN_POINT('Ctrl Pts',(-0.002593981205076,-0.0222532893141073,
-0.0147362881763453));
#17246=CARTESIAN_POINT('Ctrl Pts',(-0.00355622958286202,-0.0220941670168887,
-0.0113772316795867));
#17247=CARTESIAN_POINT('Ctrl Pts',(-0.00125012443056717,-0.0219350447196702,
-0.00875214853508845));
#17248=CARTESIAN_POINT('Ctrl Pts',(0.00220490783694106,-0.0217759224224516,
-0.00927362194710001));
#17249=CARTESIAN_POINT('Ctrl Pts',(0.00363351910309228,-0.0216168001252331,
-0.0124623916689818));
#17250=CARTESIAN_POINT('Ctrl Pts',(0.00172274388969011,-0.0214576778280145,
-0.0153878182315213));
#17251=CARTESIAN_POINT('Ctrl Pts',(-0.00177131945010908,-0.021298555530796,
-0.0153612877503014));
#17252=CARTESIAN_POINT('Ctrl Pts',(-0.00363745128471018,-0.0211394332335774,
-0.0124071830695474));
#17253=CARTESIAN_POINT('Ctrl Pts',(-0.00216058276743305,-0.0209803109363589,
-0.00924047470412463));
#17254=CARTESIAN_POINT('Ctrl Pts',(0.00130196978694757,-0.0208211886391403,
-0.00877152662905103));
#17255=CARTESIAN_POINT('Ctrl Pts',(0.00356794674066081,-0.0206620663419218,
-0.0114313256692425));
#17256=CARTESIAN_POINT('Ctrl Pts',(0.00255480150800994,-0.0205029440447033,
-0.0147753829693676));
#17257=CARTESIAN_POINT('Ctrl Pts',(-0.000806334576410288,-0.0203438217474846,
-0.0157303419794677));
#17258=CARTESIAN_POINT('Ctrl Pts',(-0.00342640870241972,-0.0201846994502662,
-0.0134185474247594));
#17259=CARTESIAN_POINT('Ctrl Pts',(-0.00289744120524209,-0.0200255771530476,
-0.00996465456656415));
#17260=CARTESIAN_POINT('Ctrl Pts',(0.00029442022796869,-0.0198664548558291,
-0.00854296434709121));
#17261=CARTESIAN_POINT('Ctrl Pts',(0.00321569469006684,-0.0197073325586105,
-0.0104600814551616));
#17262=CARTESIAN_POINT('Ctrl Pts',(0.00318158428540032,-0.019548210261392,
-0.0139540790180195));
#17263=CARTESIAN_POINT('Ctrl Pts',(0.000223438188398445,-0.0193890879641734,
-0.0158137978563808));
#17264=CARTESIAN_POINT('Ctrl Pts',(-0.00294005882163927,-0.0192299656669548,
-0.0143300629890799));
#17265=CARTESIAN_POINT('Ctrl Pts',(-0.0034014941665226,-0.0190708433697363,
-0.0108665012512935));
#17266=CARTESIAN_POINT('Ctrl Pts',(-0.000736785597562666,-0.0189117210725177,
-0.00860629977101019));
#17267=CARTESIAN_POINT('Ctrl Pts',(0.00260506592648272,-0.0187525987752992,
-0.00962669718388102));
#17268=CARTESIAN_POINT('Ctrl Pts',(0.00355273107461734,-0.0185934764780806,
-0.012989897037589));
#17269=CARTESIAN_POINT('Ctrl Pts',(0.00123525799739393,-0.0184343541808621,
-0.0156049498143626));
#17270=CARTESIAN_POINT('Ctrl Pts',(-0.0022174791965712,-0.0182752318836436,
-0.0150684907214794));
#17271=CARTESIAN_POINT('Ctrl Pts',(-0.0036322416785341,-0.018116109586425,
-0.0118735525986582));
#17272=CARTESIAN_POINT('Ctrl Pts',(-0.00170879169822517,-0.0179569872892065,
-0.00895644398528475));
#17273=CARTESIAN_POINT('Ctrl Pts',(0.00178512364400027,-0.0177978649919879,
-0.00899813415284341));
#17274=CARTESIAN_POINT('Ctrl Pts',(0.00363842073387552,-0.0176387426947694,
-0.011960307744337));
#17275=CARTESIAN_POINT('Ctrl Pts',(0.00214782649925085,-0.0174796203975508,
-0.0151205785106708));
#17276=CARTESIAN_POINT('Ctrl Pts',(-0.00131672812125129,-0.0173204981003323,
-0.0155744989538967));
#17277=CARTESIAN_POINT('Ctrl Pts',(-0.00357114349155041,-0.0171613758031137,
-0.0129048933966471));
#17278=CARTESIAN_POINT('Ctrl Pts',(-0.0025434986996575,-0.0170022535058952,
-0.00956526337694232));
#17279=CARTESIAN_POINT('Ctrl Pts',(0.000821749093176863,-0.0168431312086766,
-0.0086248965494641));
#17280=CARTESIAN_POINT('Ctrl Pts',(0.00343176821767638,-0.016684008911458,
-0.0109480372450631));
#17281=CARTESIAN_POINT('Ctrl Pts',(0.00288782004579531,-0.0165248866142396,
-0.014399602520438));
#17282=CARTESIAN_POINT('Ctrl Pts',(-0.000310179714699567,-0.0163657643170209,
-0.0158074306162551));
#17283=CARTESIAN_POINT('Ctrl Pts',(-0.00322310878159308,-0.0162066420198024,
-0.0138776567970947));
#17284=CARTESIAN_POINT('Ctrl Pts',(-0.00317383898661389,-0.0160475197225839,
-0.0103838401558357));
#17285=CARTESIAN_POINT('Ctrl Pts',(-0.000207651960708945,-0.0158883974253653,
-0.00853697346371519));
#17286=CARTESIAN_POINT('Ctrl Pts',(0.00294937792331869,-0.0157292751281468,
-0.0100344201936282));
#17287=CARTESIAN_POINT('Ctrl Pts',(0.00339578086798491,-0.0155701528309282,
-0.0134999511106268));
#17288=CARTESIAN_POINT('Ctrl Pts',(0.000721291791339459,-0.0154110305337097,
-0.0157485703134361));
#17289=CARTESIAN_POINT('Ctrl Pts',(-0.00261610278505474,-0.0152519082364911,
-0.0147136818936349));
#17290=CARTESIAN_POINT('Ctrl Pts',(-0.00354916337254134,-0.0150927859392726,
-0.0113464041316556));
#17291=CARTESIAN_POINT('Ctrl Pts',(-0.00122037285621386,-0.0149336636420541,
-0.0087414267534739));
#17292=CARTESIAN_POINT('Ctrl Pts',(0.00223001774343573,-0.0147745413448354,
-0.00929286967553652));
#17293=CARTESIAN_POINT('Ctrl Pts',(0.00363087832907891,-0.014615419047617,
-0.0124938998508358));
#17294=CARTESIAN_POINT('Ctrl Pts',(0.00169484181624943,-0.0144562967503983,
-0.0154026674369236));
#17295=CARTESIAN_POINT('Ctrl Pts',(-0.00179896197323913,-0.0142971744531799,
-0.0153457558166395));
#17296=CARTESIAN_POINT('Ctrl Pts',(-0.00363918859437698,-0.0141380521559613,
-0.0123756919760434));
#17297=CARTESIAN_POINT('Ctrl Pts',(-0.00213529131716607,-0.0139789298587427,
-0.00922167683034632));
#17298=CARTESIAN_POINT('Ctrl Pts',(0.00133197569244577,-0.0138198075615242,
-0.00878326703770384));
#17299=CARTESIAN_POINT('Ctrl Pts',(0.00357326082692228,-0.0136606852643056,
-0.0114616961695499));
#17300=CARTESIAN_POINT('Ctrl Pts',(0.00253416193417905,-0.0135015629670871,
-0.014798673676204));
#17301=CARTESIAN_POINT('Ctrl Pts',(-0.000841782375526419,-0.0133424219652438,
-0.0157208707042176));
#17302=CARTESIAN_POINT('Ctrl Pts',(-0.00256461850675379,-0.01323632172914,
-0.0141691068247504));
#17303=CARTESIAN_POINT('Ctrl Pts',(-0.00290610796466779,-0.0131832622587755,
-0.0132002457902267));
#17304=CARTESIAN_POINT('Ctrl Pts',(0.00178014132164786,-0.0271787743898808,
-0.0139559946082058));
#17305=CARTESIAN_POINT('Ctrl Pts',(0.00159188778177753,-0.027178774389881,
-0.0141905448606472));
#17306=CARTESIAN_POINT('Ctrl Pts',(0.00136108477584615,-0.0271787743898809,
-0.0143859446782764));
#17307=CARTESIAN_POINT('Ctrl Pts',(0.00110253657449065,-0.0271787743898808,
-0.0145397492409188));
#17308=CARTESIAN_POINT('Ctrl Pts',(0.00108435986445509,-0.0271787743898808,
-0.014550562160609));
#17309=CARTESIAN_POINT('Ctrl Pts',(0.00106604363144548,-0.0271787743898808,
-0.0145611678146568));
#17310=CARTESIAN_POINT('Ctrl Pts',(0.00104759204748925,-0.0271787743898808,
-0.0145715645217343));
#17311=CARTESIAN_POINT('Ctrl Pts',(0.00102977915444992,-0.0271787743898808,
-0.0145816013528038));
#17312=CARTESIAN_POINT('Ctrl Pts',(0.00101183438704971,-0.0271787743898808,
-0.0145914463741348));
#17313=CARTESIAN_POINT('Ctrl Pts',(0.000993792858541382,-0.0271787743898807,
-0.0146010815780363));
#17314=CARTESIAN_POINT('Ctrl Pts',(0.000750757191878033,-0.0271787743898806,
-0.0147308764677853));
#17315=CARTESIAN_POINT('Ctrl Pts',(0.000489586583346331,-0.0271787743898804,
-0.0148233339409982));
#17316=CARTESIAN_POINT('Ctrl Pts',(0.000220202998773276,-0.02717877438988,
-0.0148759520475625));
#17317=CARTESIAN_POINT('Ctrl Pts',(0.000185586155698519,-0.02717877438988,
-0.0148827136798301));
#17318=CARTESIAN_POINT('Ctrl Pts',(0.000150830466630735,-0.0271787743898799,
-0.0148888130189507));
#17319=CARTESIAN_POINT('Ctrl Pts',(0.000115954661106575,-0.0271787743898799,
-0.0148942405572793));
#17320=CARTESIAN_POINT('Ctrl Pts',(9.56456236842798E-5,-0.0271787743898799,
-0.0148974011460418));
#17321=CARTESIAN_POINT('Ctrl Pts',(7.52958492378998E-5,-0.0271787743898798,
-0.0149003339054926));
#17322=CARTESIAN_POINT('Ctrl Pts',(5.49090021173358E-5,-0.0271787743898798,
-0.0149030367816552));
#17323=CARTESIAN_POINT('Ctrl Pts',(4.02446667567445E-5,-0.0271787743898798,
-0.014904980970585));
#17324=CARTESIAN_POINT('Ctrl Pts',(2.55602201095934E-5,-0.0271787743898798,
-0.0149068062467938));
#17325=CARTESIAN_POINT('Ctrl Pts',(1.08737028632742E-5,-0.0271787743898796,
-0.0149085100975743));
#17326=CARTESIAN_POINT('Ctrl Pts',(-8.37418793519446E-5,-0.0271787743898786,
-0.0149194868887972));
#17327=CARTESIAN_POINT('Ctrl Pts',(-0.000178600902109579,-0.0271787743898791,
-0.0149254498948637));
#17328=CARTESIAN_POINT('Ctrl Pts',(-0.000273310347805921,-0.0271787743898792,
-0.0149263099508221));
#17329=CARTESIAN_POINT('Ctrl Pts',(-0.000367683085058819,-0.0271787743898794,
-0.014927166949133));
#17330=CARTESIAN_POINT('Ctrl Pts',(-0.000461908229692522,-0.0271787743898795,
-0.0149229576474026));
#17331=CARTESIAN_POINT('Ctrl Pts',(-0.000555618552463728,-0.0271787743898797,
-0.0149135474060006));
#17332=CARTESIAN_POINT('Ctrl Pts',(-0.000568622442957223,-0.0271787743898797,
-0.0149122415760227));
#17333=CARTESIAN_POINT('Ctrl Pts',(-0.000581616441170821,-0.0271787743898797,
-0.0149108355161016));
#17334=CARTESIAN_POINT('Ctrl Pts',(-0.000594599583223318,-0.0271787743898797,
-0.0149093287881527));
#17335=CARTESIAN_POINT('Ctrl Pts',(-0.000686222435460218,-0.0271787743898799,
-0.0148986957139969));
#17336=CARTESIAN_POINT('Ctrl Pts',(-0.000777304615406129,-0.02717877438988,
-0.0148830535254043));
#17337=CARTESIAN_POINT('Ctrl Pts',(-0.000867587973888055,-0.0271787743898801,
-0.014862658476978));
#17338=CARTESIAN_POINT('Ctrl Pts',(-0.000904118649592721,-0.0271787743898802,
-0.0148544061820637));
#17339=CARTESIAN_POINT('Ctrl Pts',(-0.00094051853516899,-0.0271787743898802,
-0.0148453751478637));
#17340=CARTESIAN_POINT('Ctrl Pts',(-0.000976770333537329,-0.0271787743898803,
-0.0148355799669997));
#17341=CARTESIAN_POINT('Ctrl Pts',(-0.000991818294032867,-0.0271787743898803,
-0.0148315140309269));
#17342=CARTESIAN_POINT('Ctrl Pts',(-0.00100684073583925,-0.0271787743898803,
-0.0148273164133904));
#17343=CARTESIAN_POINT('Ctrl Pts',(-0.00102183640859416,-0.0271787743898803,
-0.014822988092282));
#17344=CARTESIAN_POINT('Ctrl Pts',(-0.001313021104889,-0.0271787743898808,
-0.014738941121665));
#17345=CARTESIAN_POINT('Ctrl Pts',(-0.00158953777575494,-0.0271787743898808,
-0.014607373158194));
#17346=CARTESIAN_POINT('Ctrl Pts',(-0.0018425581172716,-0.027178774389881,
-0.0144374263141347));
#17347=CARTESIAN_POINT('Ctrl Pts',(-0.00187516285324282,-0.027178774389881,
-0.0144155266046233));
#17348=CARTESIAN_POINT('Ctrl Pts',(-0.00190737673303968,-0.027178774389881,
-0.0143929827017157));
#17349=CARTESIAN_POINT('Ctrl Pts',(-0.00193917946553789,-0.027178774389881,
-0.0143698084371997));
#17350=CARTESIAN_POINT('Ctrl Pts',(-0.00196084834500122,-0.027178774389881,
-0.0143540185881836));
#17351=CARTESIAN_POINT('Ctrl Pts',(-0.00198232634019788,-0.027178774389881,
-0.0143379360750785));
#17352=CARTESIAN_POINT('Ctrl Pts',(-0.00200360683979679,-0.027178774389881,
-0.0143215649815428));
#17353=CARTESIAN_POINT('Ctrl Pts',(-0.002016225356077,-0.027178774389881,
-0.0143118575538884));
#17354=CARTESIAN_POINT('Ctrl Pts',(-0.00202877384413721,-0.027178774389881,
-0.0143020490191849));
#17355=CARTESIAN_POINT('Ctrl Pts',(-0.00204124055375976,-0.027178774389881,
-0.0142921487089482));
#17356=CARTESIAN_POINT('Ctrl Pts',(-0.00218907523485341,-0.0271787743898811,
-0.0141747473054594));
#17357=CARTESIAN_POINT('Ctrl Pts',(-0.00232581856094753,-0.0271787743898811,
-0.0140441925400865));
#17358=CARTESIAN_POINT('Ctrl Pts',(-0.0024493802750837,-0.0271787743898811,
-0.0139022590018999));
#17359=CARTESIAN_POINT('Ctrl Pts',(-0.0024731161684946,-0.027178774389881,
-0.0138749939274602));
#17360=CARTESIAN_POINT('Ctrl Pts',(-0.00249636476998995,-0.027178774389881,
-0.013847307320566));
#17361=CARTESIAN_POINT('Ctrl Pts',(-0.00251910979700554,-0.027178774389881,
-0.01381920955006));
#17362=CARTESIAN_POINT('Ctrl Pts',(-0.00253166456181397,-0.027178774389881,
-0.0138037001861844));
#17363=CARTESIAN_POINT('Ctrl Pts',(-0.0025440610497504,-0.027178774389881,
-0.013788071445362));
#17364=CARTESIAN_POINT('Ctrl Pts',(-0.00255629300276171,-0.027178774389881,
-0.0137723303642783));
#17365=CARTESIAN_POINT('Ctrl Pts',(-0.00268294210004683,-0.0271787743898809,
-0.0136093479110518));
#17366=CARTESIAN_POINT('Ctrl Pts',(-0.00279213110827008,-0.0271787743898808,
-0.0134342130497224));
#17367=CARTESIAN_POINT('Ctrl Pts',(-0.00288099910591139,-0.0271787743898807,
-0.0132489814220675));
#17368=CARTESIAN_POINT('Ctrl Pts',(-0.00288859728608324,-0.0271787743898807,
-0.0132331441879922));
#17369=CARTESIAN_POINT('Ctrl Pts',(-0.00289604652716329,-0.0271787743899213,
-0.0132172327756286));
#17370=CARTESIAN_POINT('Ctrl Pts',(-0.00290334727505161,-0.027178774389873,
-0.0132012491818455));
#17371=CARTESIAN_POINT('Ctrl Pts',(-0.00133026104482802,-0.0271737656056343,
-0.00939549384111197));
#17372=CARTESIAN_POINT('Ctrl Pts',(-0.000403564519673555,-0.0271207189867622,
-0.00895210654872306));
#17373=CARTESIAN_POINT('Ctrl Pts',(0.00191213026985457,-0.0270146316021502,
-0.00907331532630318));
#17374=CARTESIAN_POINT('Ctrl Pts',(0.00364752743133458,-0.0268555034517987,
-0.0121131487462191));
#17375=CARTESIAN_POINT('Ctrl Pts',(0.00202223804807116,-0.0266963811545802,
-0.0152083353095718));
#17376=CARTESIAN_POINT('Ctrl Pts',(-0.00145746560947327,-0.0265372588573616,
-0.0155175293308395));
#17377=CARTESIAN_POINT('Ctrl Pts',(-0.00359977297117066,-0.026378136560143,
-0.0127550489129778));
#17378=CARTESIAN_POINT('Ctrl Pts',(-0.00243264631344909,-0.0262190142629245,
-0.00946051572784691));
#17379=CARTESIAN_POINT('Ctrl Pts',(0.000969663846264036,-0.0260598919657059,
-0.00866138325036077));
#17380=CARTESIAN_POINT('Ctrl Pts',(0.00348107948700157,-0.0259007696684874,
-0.0110922917925086));
#17381=CARTESIAN_POINT('Ctrl Pts',(0.00279306816967889,-0.0257416473712688,
-0.0145190138345622));
#17382=CARTESIAN_POINT('Ctrl Pts',(-0.000461841671043204,-0.0255825250740504,
-0.0157922709603413));
#17383=CARTESIAN_POINT('Ctrl Pts',(-0.00329233215877127,-0.0254234027768317,
-0.0137418498867445));
#17384=CARTESIAN_POINT('Ctrl Pts',(-0.00309698560073088,-0.0252642804796132,
-0.0102522037919197));
#17385=CARTESIAN_POINT('Ctrl Pts',(-5.5363207118422E-5,-0.0251051581823947,
-0.00853048588183138));
#17386=CARTESIAN_POINT('Ctrl Pts',(0.0030371455487437,-0.0249460358851761,
-0.0101590447958442));
#17387=CARTESIAN_POINT('Ctrl Pts',(0.00333836262133237,-0.0247869135879575,
-0.0136411513774764));
#17388=CARTESIAN_POINT('Ctrl Pts',(0.000571458082834102,-0.024627791290739,
-0.0157765757479082));
#17389=CARTESIAN_POINT('Ctrl Pts',(-0.00272064575727319,-0.0244686689935204,
-0.0146027552459517));
#17390=CARTESIAN_POINT('Ctrl Pts',(-0.00351233923191389,-0.0243095466963019,
-0.0111984900766984));
#17391=CARTESIAN_POINT('Ctrl Pts',(-0.00107601677663968,-0.0241504243990833,
-0.00869247072691854));
#17392=CARTESIAN_POINT('Ctrl Pts',(0.00234921920222027,-0.0239913021018648,
-0.00938785485574907));
#17393=CARTESIAN_POINT('Ctrl Pts',(0.00361540474722111,-0.0238321798046462,
-0.0126455495059498));
#17394=CARTESIAN_POINT('Ctrl Pts',(0.0015588518368198,-0.0236730575074277,
-0.0154715697542866));
#17395=CARTESIAN_POINT('Ctrl Pts',(-0.00193036418608369,-0.0235139352102091,
-0.0152686611019598));
#17396=CARTESIAN_POINT('Ctrl Pts',(-0.00364547860084178,-0.0233548129129906,
-0.0122233067916808));
#17397=CARTESIAN_POINT('Ctrl Pts',(-0.00201021516003761,-0.0231956906157721,
-0.00913434032706003));
#17398=CARTESIAN_POINT('Ctrl Pts',(0.00147253693880004,-0.0230365683185534,
-0.00884067697422658));
#17399=CARTESIAN_POINT('Ctrl Pts',(0.00360195366021276,-0.022877446021335,
-0.0116122080975127));
#17400=CARTESIAN_POINT('Ctrl Pts',(0.00242099412922516,-0.0227183237241164,
-0.0149017574478925));
#17401=CARTESIAN_POINT('Ctrl Pts',(-0.000984980554711353,-0.0225592014268979,
-0.015686064017702));
#17402=CARTESIAN_POINT('Ctrl Pts',(-0.0034857086570125,-0.0224000791296793,
-0.0132443106926007));
#17403=CARTESIAN_POINT('Ctrl Pts',(-0.0027828955007027,-0.0222409568324608,
-0.00982059136855261));
#17404=CARTESIAN_POINT('Ctrl Pts',(0.000477538338332731,-0.0220818345352422,
-0.00856147599501673));
#17405=CARTESIAN_POINT('Ctrl Pts',(0.00329909046922294,-0.0219227122380236,
-0.0106241548151851));
#17406=CARTESIAN_POINT('Ctrl Pts',(0.00308861282535697,-0.0217635899408051,
-0.0141129224348428));
#17407=CARTESIAN_POINT('Ctrl Pts',(3.95449286407195E-5,-0.0216044676435865,
-0.0158214262550787));
#17408=CARTESIAN_POINT('Ctrl Pts',(-0.00304586674288027,-0.021445345346368,
-0.014179465488259));
#17409=CARTESIAN_POINT('Ctrl Pts',(-0.00333197395745346,-0.0212862230491495,
-0.0106960845150796));
#17410=CARTESIAN_POINT('Ctrl Pts',(-0.000555829820637072,-0.0211271007519309,
-0.00857268533589575));
#17411=CARTESIAN_POINT('Ctrl Pts',(0.00273114982723726,-0.0209679784547124,
-0.00976077840337707));
#17412=CARTESIAN_POINT('Ctrl Pts',(0.00350806566426024,-0.0208088561574938,
-0.0131684465393202));
#17413=CARTESIAN_POINT('Ctrl Pts',(0.0010608930305098,-0.0206497338602753,
-0.0156638716420152));
#17414=CARTESIAN_POINT('Ctrl Pts',(-0.00236129356128513,-0.0204906115630567,
-0.0149536327572187));
#17415=CARTESIAN_POINT('Ctrl Pts',(-0.00361333281957622,-0.0203314892658382,
-0.011690475078185));
#17416=CARTESIAN_POINT('Ctrl Pts',(-0.00154453780633458,-0.0201723669686196,
-0.00887340434145793));
#17417=CARTESIAN_POINT('Ctrl Pts',(0.00194376499571779,-0.020013244671401,
-0.00909144998743974));
#17418=CARTESIAN_POINT('Ctrl Pts',(0.0036456501783873,-0.0198541223741825,
-0.0121442171203124));
#17419=CARTESIAN_POINT('Ctrl Pts',(0.00199699981425714,-0.019695000076964,
-0.0152260594782847));
#17420=CARTESIAN_POINT('Ctrl Pts',(-0.00148699364019134,-0.0195358777797454,
-0.0155046092079528));
#17421=CARTESIAN_POINT('Ctrl Pts',(-0.00360436528356685,-0.0193767554825269,
-0.0127238651229339));
#17422=CARTESIAN_POINT('Ctrl Pts',(-0.00240914427122477,-0.0192176331853083,
-0.00943947064690133));
#17423=CARTESIAN_POINT('Ctrl Pts',(0.00100020127943993,-0.0190585108880898,
-0.00866994919905135));
#17424=CARTESIAN_POINT('Ctrl Pts',(0.00349031163837243,-0.0188993885908712,
-0.0111225296244144));
#17425=CARTESIAN_POINT('Ctrl Pts',(0.0027726503676781,-0.0187402662936527,
-0.0145431673782673));
#17426=CARTESIAN_POINT('Ctrl Pts',(-0.000493215794101875,-0.0185811439964341,
-0.0157881246288907));
#17427=CARTESIAN_POINT('Ctrl Pts',(-0.00330579187879757,-0.0184220216992156,
-0.0137132231588611));
#17428=CARTESIAN_POINT('Ctrl Pts',(-0.00308017925688279,-0.018262899401997,
-0.0102254015912665));
#17429=CARTESIAN_POINT('Ctrl Pts',(-2.3727254960886E-5,-0.0181037771047785,
-0.00853014305567693));
#17430=CARTESIAN_POINT('Ctrl Pts',(0.00305453128551212,-0.0179446548075599,
-0.0101854752581386));
#17431=CARTESIAN_POINT('Ctrl Pts',(0.0033255222193557,-0.0177855325103414,
-0.0136700647972919));
#17432=CARTESIAN_POINT('Ctrl Pts',(0.000540191273020311,-0.0176264102131228,
-0.0157813989399443));
#17433=CARTESIAN_POINT('Ctrl Pts',(-0.00274160257393495,-0.0174672879159043,
-0.0145790556077934));
#17434=CARTESIAN_POINT('Ctrl Pts',(-0.00350372601109839,-0.0173081656186857,
-0.0111680486876026));
#17435=CARTESIAN_POINT('Ctrl Pts',(-0.00104574933649522,-0.0171490433214672,
-0.00868326479166292));
#17436=CARTESIAN_POINT('Ctrl Pts',(0.00237332348080628,-0.0169899210242486,
-0.009408345070505));
#17437=CARTESIAN_POINT('Ctrl Pts',(0.00361119286507359,-0.0168307987270301,
-0.0126769043455143));
#17438=CARTESIAN_POINT('Ctrl Pts',(0.0015301947024884,-0.0166716764298115,
-0.0154849725405016));
#17439=CARTESIAN_POINT('Ctrl Pts',(-0.00195712921450782,-0.016512554132593,
-0.0152517940063453));
#17440=CARTESIAN_POINT('Ctrl Pts',(-0.00364575312774022,-0.0163534318353744,
-0.0121916715160949));
#17441=CARTESIAN_POINT('Ctrl Pts',(-0.00198374687138292,-0.0161943095381559,
-0.00911701128752997));
#17442=CARTESIAN_POINT('Ctrl Pts',(0.00150142234134212,-0.0160351872409373,
-0.00885358041046971));
#17443=CARTESIAN_POINT('Ctrl Pts',(0.00360670906987409,-0.0158760649437188,
-0.0116434851379063));
#17444=CARTESIAN_POINT('Ctrl Pts',(0.00239724903111026,-0.0157169426465002,
-0.0149226628552886));
#17445=CARTESIAN_POINT('Ctrl Pts',(-0.00101540311647332,-0.0155578203492816,
-0.0156773848040705));
#17446=CARTESIAN_POINT('Ctrl Pts',(-0.00349484903028939,-0.0153986980520632,
-0.0132140232339141));
#17447=CARTESIAN_POINT('Ctrl Pts',(-0.00276235281219855,-0.0152395757548446,
-0.0097965318648716));
#17448=CARTESIAN_POINT('Ctrl Pts',(0.00050888351868074,-0.0150804534576261,
-0.0085657553464899));
#17449=CARTESIAN_POINT('Ctrl Pts',(0.0033124319335464,-0.0149213311604074,
-0.0106528420306022));
#17450=CARTESIAN_POINT('Ctrl Pts',(0.00307168598205126,-0.014762208863189,
-0.0141396486977521));
#17451=CARTESIAN_POINT('Ctrl Pts',(7.91251657260586E-6,-0.0146030865659703,
-0.0158216363008853));
#17452=CARTESIAN_POINT('Ctrl Pts',(-0.00306314496881806,-0.0144439642687519,
-0.0141529515189099));
#17453=CARTESIAN_POINT('Ctrl Pts',(-0.00331899483268342,-0.0142848419715333,
-0.0106672431795996));
#17454=CARTESIAN_POINT('Ctrl Pts',(-0.000524568178194816,-0.0141257196743148,
-0.00856796635198887));
#17455=CARTESIAN_POINT('Ctrl Pts',(0.00275205403218279,-0.0139665973770961,
-0.00978463054201357));
#17456=CARTESIAN_POINT('Ctrl Pts',(0.003499221564516,-0.0138074750798777,
-0.0131987289322313));
#17457=CARTESIAN_POINT('Ctrl Pts',(0.0010307800885073,-0.0136483527826591,
-0.0156731844728732));
#17458=CARTESIAN_POINT('Ctrl Pts',(-0.00238569018355137,-0.0134892304854405,
-0.0149325700177128));
#17459=CARTESIAN_POINT('Ctrl Pts',(-0.00360823372354723,-0.013330108188222,
-0.0116600593943641));
#17460=CARTESIAN_POINT('Ctrl Pts',(-0.00151732056346516,-0.0131709858910035,
-0.00885830501571057));
#17461=CARTESIAN_POINT('Ctrl Pts',(0.00197391249517797,-0.0130118514625948,
-0.00911217318149874));
#17462=CARTESIAN_POINT('Ctrl Pts',(0.00308245941021202,-0.0129057577999257,
-0.0111491278697729));
#17463=CARTESIAN_POINT('Ctrl Pts',(0.00308220579556829,-0.0128527049029959,
-0.0121765580884125));
#17464=CARTESIAN_POINT('Ctrl Pts',(-0.00124852020439948,-0.0272831116917783,
-0.00956633919409565));
#17465=CARTESIAN_POINT('Ctrl Pts',(-0.000378766602653055,-0.0272300650729058,
-0.00915019681732398));
#17466=CARTESIAN_POINT('Ctrl Pts',(0.00179463518430394,-0.0271239776882938,
-0.00926395765272372));
#17467=CARTESIAN_POINT('Ctrl Pts',(0.00342339701807277,-0.0269648495379425,
-0.0121170017657793));
#17468=CARTESIAN_POINT('Ctrl Pts',(0.00189797714586813,-0.0268057272407237,
-0.0150219977255996));
#17469=CARTESIAN_POINT('Ctrl Pts',(-0.00136790840242943,-0.0266466049435053,
-0.015312192634436));
#17470=CARTESIAN_POINT('Ctrl Pts',(-0.00337857693663336,-0.0264874826462867,
-0.0127194589530521));
#17471=CARTESIAN_POINT('Ctrl Pts',(-0.00228316696509127,-0.0263283603490681,
-0.00962736566678117));
#17472=CARTESIAN_POINT('Ctrl Pts',(0.000910080700508586,-0.0261692380518497,
-0.00887733765685602));
#17473=CARTESIAN_POINT('Ctrl Pts',(0.00326717683686211,-0.026010115754631,
-0.011158873631858));
#17474=CARTESIAN_POINT('Ctrl Pts',(0.00262144190094663,-0.0258509934574125,
-0.0143750331375423));
#17475=CARTESIAN_POINT('Ctrl Pts',(-0.000433462785197627,-0.0256918711601939,
-0.0155700521551341));
#17476=CARTESIAN_POINT('Ctrl Pts',(-0.00309002750685791,-0.0255327488629754,
-0.0136456237522536));
#17477=CARTESIAN_POINT('Ctrl Pts',(-0.00290668445135645,-0.0253736265657569,
-0.0103704067017869));
#17478=CARTESIAN_POINT('Ctrl Pts',(-5.19612920610198E-5,-0.0252145042685382,
-0.00875448356746734));
#17479=CARTESIAN_POINT('Ctrl Pts',(0.0028505214040893,-0.0250553819713197,
-0.0102829720668527));
#17480=CARTESIAN_POINT('Ctrl Pts',(0.00313322952555102,-0.0248962596741012,
-0.0135511128862376));
#17481=CARTESIAN_POINT('Ctrl Pts',(0.000536343573436004,-0.0247371373768827,
-0.0155553213698408));
#17482=CARTESIAN_POINT('Ctrl Pts',(-0.00255346964430465,-0.0245780150796641,
-0.0144536288721698));
#17483=CARTESIAN_POINT('Ctrl Pts',(-0.00329651575741394,-0.0244188927824455,
-0.0112585463269271));
#17484=CARTESIAN_POINT('Ctrl Pts',(-0.0010098985391857,-0.024259770485227,
-0.0089065148944645));
#17485=CARTESIAN_POINT('Ctrl Pts',(0.00220486621775386,-0.0241006481880085,
-0.00955916960313173));
#17486=CARTESIAN_POINT('Ctrl Pts',(0.003393248183533,-0.02394152589079,
-0.0126166879799594));
#17487=CARTESIAN_POINT('Ctrl Pts',(0.00146306472816122,-0.0237824035935714,
-0.015269057146003));
#17488=CARTESIAN_POINT('Ctrl Pts',(-0.00181174867710741,-0.0236232812963528,
-0.0150786166658714));
#17489=CARTESIAN_POINT('Ctrl Pts',(-0.00342147408251391,-0.0234641589991344,
-0.0122203909058064));
#17490=CARTESIAN_POINT('Ctrl Pts',(-0.00188669303085664,-0.0233050367019156,
-0.00932123283695521));
#17491=CARTESIAN_POINT('Ctrl Pts',(0.0013820536404974,-0.0231459144046971,
-0.00904561428018408));
#17492=CARTESIAN_POINT('Ctrl Pts',(0.0033806236284005,-0.0229867921074786,
-0.011646842526323));
#17493=CARTESIAN_POINT('Ctrl Pts',(0.00227223077517162,-0.02282766981026,
-0.0147342582206233));
#17494=CARTESIAN_POINT('Ctrl Pts',(-0.000924456239832787,-0.0226685475130416,
-0.0154703713336528));
#17495=CARTESIAN_POINT('Ctrl Pts',(-0.00327152155725417,-0.022509425215823,
-0.0131786569574399));
#17496=CARTESIAN_POINT('Ctrl Pts',(-0.00261189431417872,-0.0223503029186044,
-0.00996531566109326));
#17497=CARTESIAN_POINT('Ctrl Pts',(0.000448194935950225,-0.0221911806213858,
-0.00878356942441171));
#17498=CARTESIAN_POINT('Ctrl Pts',(0.00309637053793389,-0.0220320583241672,
-0.0107195023694375));
#17499=CARTESIAN_POINT('Ctrl Pts',(0.00289882615973626,-0.0218729360269489,
-0.0139938949245925));
#17500=CARTESIAN_POINT('Ctrl Pts',(3.71150027894397E-5,-0.0217138137297301,
-0.0155974159381194));
#17501=CARTESIAN_POINT('Ctrl Pts',(-0.00285870670510849,-0.0215546914325116,
-0.0140563490924984));
#17502=CARTESIAN_POINT('Ctrl Pts',(-0.00312723342729426,-0.0213955691352931,
-0.0107870121893814));
#17503=CARTESIAN_POINT('Ctrl Pts',(-0.000521675624473279,-0.0212364468380746,
-0.00879408998247798));
#17504=CARTESIAN_POINT('Ctrl Pts',(0.00256332826839168,-0.021077324540856,
-0.00990917803622847));
#17505=CARTESIAN_POINT('Ctrl Pts',(0.00329250478860355,-0.0209182022436374,
-0.0131074544453246));
#17506=CARTESIAN_POINT('Ctrl Pts',(0.000995704105181346,-0.0207590799464189,
-0.015449542617713));
#17507=CARTESIAN_POINT('Ctrl Pts',(-0.00221619864104495,-0.0205999576492002,
-0.0147829459365079));
#17508=CARTESIAN_POINT('Ctrl Pts',(-0.00339130357007781,-0.020440835351982,
-0.011720300218771));
#17509=CARTESIAN_POINT('Ctrl Pts',(-0.00144963025502779,-0.0202817130547632,
-0.00907633064174633));
#17510=CARTESIAN_POINT('Ctrl Pts',(0.00182432604427043,-0.0201225907575447,
-0.00928097798938392));
#17511=CARTESIAN_POINT('Ctrl Pts',(0.00342163511709659,-0.0199634684603261,
-0.0121461610747165));
#17512=CARTESIAN_POINT('Ctrl Pts',(0.0018742897313094,-0.0198043461631076,
-0.0150386327934535));
#17513=CARTESIAN_POINT('Ctrl Pts',(-0.00139562201780662,-0.0196452238658891,
-0.0153000664171568));
#17514=CARTESIAN_POINT('Ctrl Pts',(-0.0033828870642086,-0.0194861015686706,
-0.0126901913201535));
#17515=CARTESIAN_POINT('Ctrl Pts',(-0.00226110905797912,-0.0193269792714519,
-0.00960761374751241));
#17516=CARTESIAN_POINT('Ctrl Pts',(0.000938741693370724,-0.0191678569742334,
-0.00888537725182994));
#17517=CARTESIAN_POINT('Ctrl Pts',(0.00327584169821501,-0.0190087346770149,
-0.0111872534331147));
#17518=CARTESIAN_POINT('Ctrl Pts',(0.00260227871607661,-0.0188496123797963,
-0.0143977025131817));
#17519=CARTESIAN_POINT('Ctrl Pts',(-0.000462909055676917,-0.0186904900825777,
-0.0155661606042158));
#17520=CARTESIAN_POINT('Ctrl Pts',(-0.00310266016453344,-0.0185313677853593,
-0.0136187560571594));
#17521=CARTESIAN_POINT('Ctrl Pts',(-0.0028909108105827,-0.0183722454881406,
-0.0103452514218003));
#17522=CARTESIAN_POINT('Ctrl Pts',(-2.22692811525819E-5,-0.0182131231909222,
-0.00875416180702642));
#17523=CARTESIAN_POINT('Ctrl Pts',(0.00286683883570031,-0.0180540008937035,
-0.0103077784507683));
#17524=CARTESIAN_POINT('Ctrl Pts',(0.00312117813055393,-0.017894878596485,
-0.0135782496568423));
#17525=CARTESIAN_POINT('Ctrl Pts',(0.000506998022101241,-0.0177357562992665,
-0.0155598481901445));
#17526=CARTESIAN_POINT('Ctrl Pts',(-0.00257313872288425,-0.0175766340020479,
-0.0144313855108441));
#17527=CARTESIAN_POINT('Ctrl Pts',(-0.00328843179505563,-0.0174175117048294,
-0.0112299754765036));
#17528=CARTESIAN_POINT('Ctrl Pts',(-0.000981490949034324,-0.0172583894076109,
-0.00889787463831949));
#17529=CARTESIAN_POINT('Ctrl Pts',(0.00222748935547867,-0.0170992671103922,
-0.00957840075119452));
#17530=CARTESIAN_POINT('Ctrl Pts',(0.00338929510982602,-0.0169401448131737,
-0.0126461161518617));
#17531=CARTESIAN_POINT('Ctrl Pts',(0.00143616849501057,-0.0167810225159553,
-0.0152816363682914));
#17532=CARTESIAN_POINT('Ctrl Pts',(-0.00183686906899497,-0.0166219002187365,
-0.015062786006358));
#17533=CARTESIAN_POINT('Ctrl Pts',(-0.00342173174049819,-0.0164627779215181,
-0.012190699529896));
#17534=CARTESIAN_POINT('Ctrl Pts',(-0.00186185114490522,-0.0163036556242994,
-0.00930496861869497));
#17535=CARTESIAN_POINT('Ctrl Pts',(0.00140916411541224,-0.016144533327081,
-0.00905772483616733));
#17536=CARTESIAN_POINT('Ctrl Pts',(0.00338508683136765,-0.0159854110298623,
-0.0116761976795967));
#17537=CARTESIAN_POINT('Ctrl Pts',(0.00224994474727718,-0.0158262887326441,
-0.0147538790488936));
#17538=CARTESIAN_POINT('Ctrl Pts',(-0.000953009419809811,-0.0156671664354252,
-0.0154622254335535));
#17539=CARTESIAN_POINT('Ctrl Pts',(-0.00328010028002164,-0.0155080441382069,
-0.0131502305788299));
#17540=CARTESIAN_POINT('Ctrl Pts',(-0.00259261391673356,-0.0153489218409881,
-0.00994273454698003));
#17541=CARTESIAN_POINT('Ctrl Pts',(0.000477614042167904,-0.0151897995437698,
-0.00878758582164199));
#17542=CARTESIAN_POINT('Ctrl Pts',(0.00310889220639052,-0.015030677246551,
-0.0107464268352748));
#17543=CARTESIAN_POINT('Ctrl Pts',(0.00288293942386135,-0.0148715549493327,
-0.0140189789329983));
#17544=CARTESIAN_POINT('Ctrl Pts',(7.42631444178104E-6,-0.0147124326521141,
-0.0155976130771956));
#17545=CARTESIAN_POINT('Ctrl Pts',(-0.0028749232321303,-0.0145533103548955,
-0.0140314643328042));
#17546=CARTESIAN_POINT('Ctrl Pts',(-0.0031150518336335,-0.0143941880576769,
-0.0107599430737303));
#17547=CARTESIAN_POINT('Ctrl Pts',(-0.000492334922989443,-0.0142350657604584,
-0.00878966096700406));
#17548=CARTESIAN_POINT('Ctrl Pts',(0.00258294796809865,-0.0140759434632399,
-0.00993156452730224));
#17549=CARTESIAN_POINT('Ctrl Pts',(0.00328420413418439,-0.0139168211660213,
-0.013135876069437));
#17550=CARTESIAN_POINT('Ctrl Pts',(0.000967441519690922,-0.0137576988688027,
-0.0154582832010229));
#17551=CARTESIAN_POINT('Ctrl Pts',(-0.00223909615874415,-0.0135985765715841,
-0.0147631774437484));
#17552=CARTESIAN_POINT('Ctrl Pts',(-0.00338651779931415,-0.0134394542743657,
-0.0116917534941046));
#17553=CARTESIAN_POINT('Ctrl Pts',(-0.00142408543601453,-0.013280331977147,
-0.00906215912755997));
#17554=CARTESIAN_POINT('Ctrl Pts',(0.0018526210637589,-0.0131211975487384,
-0.00930042780081984));
#17555=CARTESIAN_POINT('Ctrl Pts',(0.00289305085483324,-0.0130151038860693,
-0.011212217290292));
#17556=CARTESIAN_POINT('Ctrl Pts',(0.00289281282410381,-0.0129620509891397,
-0.0121765147802993));
#17557=CARTESIAN_POINT('Ctrl Pts',(-0.00116677936397096,-0.0273924577779218,
-0.00973718454707944));
#17558=CARTESIAN_POINT('Ctrl Pts',(-0.000353968685632551,-0.0273394111590494,
-0.00934828708592501));
#17559=CARTESIAN_POINT('Ctrl Pts',(0.00167714009875331,-0.0272333237744374,
-0.00945459997914426));
#17560=CARTESIAN_POINT('Ctrl Pts',(0.00319926660481094,-0.0270741956240859,
-0.0121208547853397));
#17561=CARTESIAN_POINT('Ctrl Pts',(0.00177371624366508,-0.0269150733268674,
-0.0148356601416275));
#17562=CARTESIAN_POINT('Ctrl Pts',(-0.00127835119538558,-0.0267559510296487,
-0.0151068559380321));
#17563=CARTESIAN_POINT('Ctrl Pts',(-0.00315738090209607,-0.0265968287324303,
-0.0126838689931265));
#17564=CARTESIAN_POINT('Ctrl Pts',(-0.00213368761673345,-0.0264377064352117,
-0.00979421560571543));
#17565=CARTESIAN_POINT('Ctrl Pts',(0.000850497554753141,-0.0262785841379932,
-0.00909329206335137));
#17566=CARTESIAN_POINT('Ctrl Pts',(0.00305327418672263,-0.0261194618407746,
-0.0112254554712075));
#17567=CARTESIAN_POINT('Ctrl Pts',(0.00244981563221435,-0.0259603395435561,
-0.0142310524405224));
#17568=CARTESIAN_POINT('Ctrl Pts',(-0.000405083899352055,-0.0258012172463375,
-0.0153478333499265));
#17569=CARTESIAN_POINT('Ctrl Pts',(-0.00288772285494454,-0.025642094949119,
-0.013549397617763));
#17570=CARTESIAN_POINT('Ctrl Pts',(-0.00271638330198203,-0.0254829726519004,
-0.0104886096116541));
#17571=CARTESIAN_POINT('Ctrl Pts',(-4.85593770036155E-5,-0.0253238503546819,
-0.00897848125310329));
#17572=CARTESIAN_POINT('Ctrl Pts',(0.00266389725943493,-0.0251647280574633,
-0.0104068993378612));
#17573=CARTESIAN_POINT('Ctrl Pts',(0.00292809642976967,-0.0250056057602447,
-0.0134610743949989));
#17574=CARTESIAN_POINT('Ctrl Pts',(0.000501229064037909,-0.0248464834630263,
-0.0153340669917736));
#17575=CARTESIAN_POINT('Ctrl Pts',(-0.0023862935313361,-0.0246873611658076,
-0.0143045024983878));
#17576=CARTESIAN_POINT('Ctrl Pts',(-0.00308069228291397,-0.0245282388685892,
-0.011318602577156));
#17577=CARTESIAN_POINT('Ctrl Pts',(-0.000943780301731716,-0.0243691165713705,
-0.00912055906201046));
#17578=CARTESIAN_POINT('Ctrl Pts',(0.00206051323328746,-0.0242099942741521,
-0.00973048435051448));
#17579=CARTESIAN_POINT('Ctrl Pts',(0.00317109161984489,-0.0240508719769334,
-0.0125878264539693));
#17580=CARTESIAN_POINT('Ctrl Pts',(0.00136727761950265,-0.023891749679715,
-0.0150665445377193));
#17581=CARTESIAN_POINT('Ctrl Pts',(-0.00169313316813111,-0.0237326273824963,
-0.0148885722297828));
#17582=CARTESIAN_POINT('Ctrl Pts',(-0.00319746956418605,-0.0235735050852778,
-0.0122174750199319));
#17583=CARTESIAN_POINT('Ctrl Pts',(-0.00176317090167569,-0.0234143827880593,
-0.00950812534685026));
#17584=CARTESIAN_POINT('Ctrl Pts',(0.00129157034219474,-0.0232552604908407,
-0.0092505515861417));
#17585=CARTESIAN_POINT('Ctrl Pts',(0.00315929359658823,-0.0230961381936222,
-0.0116814769551331));
#17586=CARTESIAN_POINT('Ctrl Pts',(0.00212346742111806,-0.0229370158964036,
-0.0145667589933541));
#17587=CARTESIAN_POINT('Ctrl Pts',(-0.000863931924954216,-0.0227778935991851,
-0.0152546786496038));
#17588=CARTESIAN_POINT('Ctrl Pts',(-0.00305733445749584,-0.0226187713019664,
-0.013113003222279));
#17589=CARTESIAN_POINT('Ctrl Pts',(-0.00244089312765475,-0.022459649004748,
-0.0101100399536339));
#17590=CARTESIAN_POINT('Ctrl Pts',(0.000418851533567719,-0.0223005267075294,
-0.00900566285380667));
#17591=CARTESIAN_POINT('Ctrl Pts',(0.00289365060664484,-0.0221414044103109,
-0.0108148499236899));
#17592=CARTESIAN_POINT('Ctrl Pts',(0.00270903949411558,-0.0219822821130924,
-0.0138748674143422));
#17593=CARTESIAN_POINT('Ctrl Pts',(3.46850769381592E-5,-0.0218231598158738,
-0.0153734056211602));
#17594=CARTESIAN_POINT('Ctrl Pts',(-0.00267154666733671,-0.0216640375186552,
-0.0139332326967378));
#17595=CARTESIAN_POINT('Ctrl Pts',(-0.00292249289713507,-0.0215049152214367,
-0.0108779398636833));
#17596=CARTESIAN_POINT('Ctrl Pts',(-0.000487521428309481,-0.0213457929242181,
-0.00901549462906021));
#17597=CARTESIAN_POINT('Ctrl Pts',(0.00239550670954607,-0.0211866706269996,
-0.0100575776690799));
#17598=CARTESIAN_POINT('Ctrl Pts',(0.00307694391294687,-0.021027548329781,
-0.0130464623513294));
#17599=CARTESIAN_POINT('Ctrl Pts',(0.000930515179852897,-0.0208684260325625,
-0.0152352135934109));
#17600=CARTESIAN_POINT('Ctrl Pts',(-0.0020711037208048,-0.0207093037353439,
-0.0146122591157974));
#17601=CARTESIAN_POINT('Ctrl Pts',(-0.00316927432057939,-0.0205501814381254,
-0.011750125359357));
#17602=CARTESIAN_POINT('Ctrl Pts',(-0.00135472270372102,-0.0203910591409068,
-0.00927925694203484));
#17603=CARTESIAN_POINT('Ctrl Pts',(0.00170488709282307,-0.0202319368436883,
-0.00947050599132809));
#17604=CARTESIAN_POINT('Ctrl Pts',(0.00319762005580587,-0.0200728145464697,
-0.0121481050291209));
#17605=CARTESIAN_POINT('Ctrl Pts',(0.00175157964836166,-0.0199136922492512,
-0.0148512061086225));
#17606=CARTESIAN_POINT('Ctrl Pts',(-0.00130425039542191,-0.0197545699520326,
-0.0150955236263609));
#17607=CARTESIAN_POINT('Ctrl Pts',(-0.00316140884485033,-0.0195954476548141,
-0.0126565175173729));
#17608=CARTESIAN_POINT('Ctrl Pts',(-0.00211307384473349,-0.0194363253575955,
-0.00977575684812358));
#17609=CARTESIAN_POINT('Ctrl Pts',(0.000877282107301528,-0.019277203060377,
-0.00910080530460862));
#17610=CARTESIAN_POINT('Ctrl Pts',(0.00306137175805757,-0.0191180807631584,
-0.0112519772418149));
#17611=CARTESIAN_POINT('Ctrl Pts',(0.00243190706447511,-0.0189589584659399,
-0.014252237648096));
#17612=CARTESIAN_POINT('Ctrl Pts',(-0.000432602317251961,-0.0187998361687213,
-0.015344196579541));
#17613=CARTESIAN_POINT('Ctrl Pts',(-0.0028995284502693,-0.0186407138715028,
-0.0135242889554577));
#17614=CARTESIAN_POINT('Ctrl Pts',(-0.00270164236428262,-0.0184815915742842,
-0.010465101252334));
#17615=CARTESIAN_POINT('Ctrl Pts',(-2.08113073442808E-5,-0.0183224692770657,
-0.0089781805583758));
#17616=CARTESIAN_POINT('Ctrl Pts',(0.0026791463858885,-0.0181633469798471,
-0.0104300816433981));
#17617=CARTESIAN_POINT('Ctrl Pts',(0.00291683404175214,-0.0180042246826286,
-0.0134864345163929));
#17618=CARTESIAN_POINT('Ctrl Pts',(0.000473804771182178,-0.0178451023854101,
-0.0153382974403444));
#17619=CARTESIAN_POINT('Ctrl Pts',(-0.00240467487183354,-0.0176859800881915,
-0.0142837154138948));
#17620=CARTESIAN_POINT('Ctrl Pts',(-0.00307313757901286,-0.017526857790973,
-0.0112919022654047));
#17621=CARTESIAN_POINT('Ctrl Pts',(-0.00091723256157343,-0.0173677354937544,
-0.00911248448497608));
#17622=CARTESIAN_POINT('Ctrl Pts',(0.00208165523015107,-0.0172086131965359,
-0.00974845643188416));
#17623=CARTESIAN_POINT('Ctrl Pts',(0.00316739735457846,-0.0170494908993173,
-0.012615327958209));
#17624=CARTESIAN_POINT('Ctrl Pts',(0.00134214228753273,-0.0168903686020988,
-0.0150783001960814));
#17625=CARTESIAN_POINT('Ctrl Pts',(-0.00171660892348211,-0.0167312463048801,
-0.014873778006371));
#17626=CARTESIAN_POINT('Ctrl Pts',(-0.00319771035325614,-0.0165721240076617,
-0.0121897275436972));
#17627=CARTESIAN_POINT('Ctrl Pts',(-0.0017399554184275,-0.016413001710443,
-0.00949292594985999));
#17628=CARTESIAN_POINT('Ctrl Pts',(0.00131690588948234,-0.0162538794132246,
-0.00926186926186496));
#17629=CARTESIAN_POINT('Ctrl Pts',(0.00316346459286122,-0.016094757116006,
-0.0117089102212872));
#17630=CARTESIAN_POINT('Ctrl Pts',(0.0021026404634441,-0.0159356348187875,
-0.0145850952424985));
#17631=CARTESIAN_POINT('Ctrl Pts',(-0.000890615723146306,-0.0157765125215689,
-0.0152470660630366));
#17632=CARTESIAN_POINT('Ctrl Pts',(-0.00306535152975389,-0.0156173902243503,
-0.0130864379237458));
#17633=CARTESIAN_POINT('Ctrl Pts',(-0.00242287502126856,-0.0154582679271319,
-0.0100889372290884));
#17634=CARTESIAN_POINT('Ctrl Pts',(0.000446344565655069,-0.0152991456299132,
-0.00900941629679401));
#17635=CARTESIAN_POINT('Ctrl Pts',(0.00290535247923465,-0.0151400233326947,
-0.0108400116399476));
#17636=CARTESIAN_POINT('Ctrl Pts',(0.00269419286567144,-0.0149809010354761,
-0.0138983091682443));
#17637=CARTESIAN_POINT('Ctrl Pts',(6.94011231095411E-6,-0.0148217787382576,
-0.0153735898535058));
#17638=CARTESIAN_POINT('Ctrl Pts',(-0.00268670149544254,-0.0146626564410391,
-0.0139099771466985));
#17639=CARTESIAN_POINT('Ctrl Pts',(-0.0029111088345836,-0.0145035341438205,
-0.010852642967861));
#17640=CARTESIAN_POINT('Ctrl Pts',(-0.00046010166778407,-0.014344411846602,
-0.00901135558201923));
#17641=CARTESIAN_POINT('Ctrl Pts',(0.00241384190401448,-0.0141852895493834,
-0.0100784985125909));
#17642=CARTESIAN_POINT('Ctrl Pts',(0.00306918670385278,-0.0140261672521649,
-0.0130730232066427));
#17643=CARTESIAN_POINT('Ctrl Pts',(0.00090410295087455,-0.0138670449549463,
-0.0152433819291725));
#17644=CARTESIAN_POINT('Ctrl Pts',(-0.00209250213393695,-0.0137079226577278,
-0.014593784869784));
#17645=CARTESIAN_POINT('Ctrl Pts',(-0.00316480187508107,-0.0135488003605092,
-0.0117234475938452));
#17646=CARTESIAN_POINT('Ctrl Pts',(-0.00133085030856392,-0.0133896780632907,
-0.00926601323940937));
#17647=CARTESIAN_POINT('Ctrl Pts',(0.00173132963233982,-0.013230543634882,
-0.00948868242014083));
#17648=CARTESIAN_POINT('Ctrl Pts',(0.00270364229945445,-0.0131244499722128,
-0.0112753067108111));
#17649=CARTESIAN_POINT('Ctrl Pts',(0.00270341985263931,-0.0130713970752832,
-0.0121764714721861));
#17650=CARTESIAN_POINT('Ctrl Pts',(-0.00108503852354243,-0.0275018038640655,
-0.00990802990006322));
#17651=CARTESIAN_POINT('Ctrl Pts',(-0.000329170768612048,-0.027448757245193,
-0.00954637735452592));
#17652=CARTESIAN_POINT('Ctrl Pts',(0.00155964501320267,-0.027342669860581,
-0.0096452423055648));
#17653=CARTESIAN_POINT('Ctrl Pts',(0.00297513619154912,-0.0271835417102296,
-0.0121247078048999));
#17654=CARTESIAN_POINT('Ctrl Pts',(0.00164945534146205,-0.027024419413011,
-0.0146493225576553));
#17655=CARTESIAN_POINT('Ctrl Pts',(-0.00118879398834175,-0.0268652971157925,
-0.0149015192416286));
#17656=CARTESIAN_POINT('Ctrl Pts',(-0.00293618486755879,-0.0267061748185738,
-0.0126482790332008));
#17657=CARTESIAN_POINT('Ctrl Pts',(-0.00198420826837562,-0.0265470525213553,
-0.0099610655446497));
#17658=CARTESIAN_POINT('Ctrl Pts',(0.000790914408997691,-0.0263879302241368,
-0.00930924646984662));
#17659=CARTESIAN_POINT('Ctrl Pts',(0.00283937153658315,-0.0262288079269182,
-0.0112920373105569));
#17660=CARTESIAN_POINT('Ctrl Pts',(0.00227818936348208,-0.0260696856296996,
-0.0140870717435024));
#17661=CARTESIAN_POINT('Ctrl Pts',(-0.000376705013506482,-0.0259105633324811,
-0.0151256145447191));
#17662=CARTESIAN_POINT('Ctrl Pts',(-0.00268541820303118,-0.0257514410352626,
-0.0134531714832721));
#17663=CARTESIAN_POINT('Ctrl Pts',(-0.0025260821526076,-0.025592318738044,
-0.0106068125215213));
#17664=CARTESIAN_POINT('Ctrl Pts',(-4.51574619462108E-5,-0.0254331964408255,
-0.00920247893873924));
#17665=CARTESIAN_POINT('Ctrl Pts',(0.00247727311478055,-0.0252740741436069,
-0.0105308266088694));
#17666=CARTESIAN_POINT('Ctrl Pts',(0.00272296333398834,-0.0251149518463884,
-0.01337103590376));
#17667=CARTESIAN_POINT('Ctrl Pts',(0.000466114554639811,-0.0249558295491698,
-0.0151128126137062));
#17668=CARTESIAN_POINT('Ctrl Pts',(-0.00221911741836756,-0.0247967072519513,
-0.014155376124606));
#17669=CARTESIAN_POINT('Ctrl Pts',(-0.00286486880841401,-0.0246375849547327,
-0.0113786588273848));
#17670=CARTESIAN_POINT('Ctrl Pts',(-0.000877662064277731,-0.0244784626575142,
-0.0093346032295564));
#17671=CARTESIAN_POINT('Ctrl Pts',(0.00191616024882105,-0.0243193403602956,
-0.00990179909789713));
#17672=CARTESIAN_POINT('Ctrl Pts',(0.0029489350561568,-0.0241602180630771,
-0.0125589649279788));
#17673=CARTESIAN_POINT('Ctrl Pts',(0.00127149051084408,-0.0240010957658585,
-0.0148640319294356));
#17674=CARTESIAN_POINT('Ctrl Pts',(-0.00157451765915481,-0.02384197346864,
-0.0146985277936943));
#17675=CARTESIAN_POINT('Ctrl Pts',(-0.00297346504585819,-0.0236828511714214,
-0.0122145591340574));
#17676=CARTESIAN_POINT('Ctrl Pts',(-0.00163964877249473,-0.0235237288742029,
-0.00969501785674544));
#17677=CARTESIAN_POINT('Ctrl Pts',(0.0012010870438921,-0.0233646065769843,
-0.00945548889209919));
#17678=CARTESIAN_POINT('Ctrl Pts',(0.00293796356477596,-0.0232054842797658,
-0.0117161113839433));
#17679=CARTESIAN_POINT('Ctrl Pts',(0.00197470406706451,-0.0230463619825472,
-0.0143992597660848));
#17680=CARTESIAN_POINT('Ctrl Pts',(-0.00080340761007565,-0.0228872396853287,
-0.0150389859655547));
#17681=CARTESIAN_POINT('Ctrl Pts',(-0.00284314735773751,-0.0227281173881101,
-0.0130473494871182));
#17682=CARTESIAN_POINT('Ctrl Pts',(-0.00226989194113077,-0.0225689950908916,
-0.0102547642461744));
#17683=CARTESIAN_POINT('Ctrl Pts',(0.000389508131185215,-0.022409872793673,
-0.00922775628320164));
#17684=CARTESIAN_POINT('Ctrl Pts',(0.00269093067535579,-0.0222507504964545,
-0.0109101974779424));
#17685=CARTESIAN_POINT('Ctrl Pts',(0.00251925282849487,-0.0220916281992359,
-0.0137558399040919));
#17686=CARTESIAN_POINT('Ctrl Pts',(3.22551510868797E-5,-0.0219325059020174,
-0.0151493953042011));
#17687=CARTESIAN_POINT('Ctrl Pts',(-0.00248438662956492,-0.0217733836047988,
-0.0138101163009774));
#17688=CARTESIAN_POINT('Ctrl Pts',(-0.00271775236697587,-0.0216142613075803,
-0.0109688675379851));
#17689=CARTESIAN_POINT('Ctrl Pts',(-0.000453367232145684,-0.0214551390103618,
-0.00923689927564244));
#17690=CARTESIAN_POINT('Ctrl Pts',(0.00222768515070049,-0.0212960167131432,
-0.0102059773019314));
#17691=CARTESIAN_POINT('Ctrl Pts',(0.00286138303729019,-0.0211368944159246,
-0.012985470257334));
#17692=CARTESIAN_POINT('Ctrl Pts',(0.000865326254524445,-0.0209777721187061,
-0.0150208845691086));
#17693=CARTESIAN_POINT('Ctrl Pts',(-0.00192600880056463,-0.0208186498214876,
-0.0144415722950867));
#17694=CARTESIAN_POINT('Ctrl Pts',(-0.00294724507108097,-0.020659527524269,
-0.0117799504999432));
#17695=CARTESIAN_POINT('Ctrl Pts',(-0.00125981515241424,-0.0205004052270504,
-0.00948218324232324));
#17696=CARTESIAN_POINT('Ctrl Pts',(0.00158544814137571,-0.0203412829298319,
-0.00966003399327228));
#17697=CARTESIAN_POINT('Ctrl Pts',(0.00297360499451516,-0.0201821606326133,
-0.0121500489835251));
#17698=CARTESIAN_POINT('Ctrl Pts',(0.00162886956541392,-0.0200230383353948,
-0.0146637794237914));
#17699=CARTESIAN_POINT('Ctrl Pts',(-0.00121287877303721,-0.0198639160381762,
-0.0148909808355651));
#17700=CARTESIAN_POINT('Ctrl Pts',(-0.00293993062549207,-0.0197047937409577,
-0.0126228437145923));
#17701=CARTESIAN_POINT('Ctrl Pts',(-0.00196503863148784,-0.0195456714437391,
-0.00994389994873465));
#17702=CARTESIAN_POINT('Ctrl Pts',(0.00081582252123233,-0.0193865491465206,
-0.00931623335738731));
#17703=CARTESIAN_POINT('Ctrl Pts',(0.00284690181790013,-0.0192274268493021,
-0.0113167010505152));
#17704=CARTESIAN_POINT('Ctrl Pts',(0.00226153541287361,-0.0190683045520835,
-0.0141067727830104));
#17705=CARTESIAN_POINT('Ctrl Pts',(-0.000402295578827005,-0.018909182254865,
-0.0151222325548662));
#17706=CARTESIAN_POINT('Ctrl Pts',(-0.00269639673600516,-0.0187500599576464,
-0.013429821853756));
#17707=CARTESIAN_POINT('Ctrl Pts',(-0.00251237391798254,-0.0185909376604278,
-0.0105849510828679));
#17708=CARTESIAN_POINT('Ctrl Pts',(-1.93533335359779E-5,-0.0184318153632094,
-0.00920219930972517));
#17709=CARTESIAN_POINT('Ctrl Pts',(0.00249145393607667,-0.0182726930659907,
-0.010552384836028));
#17710=CARTESIAN_POINT('Ctrl Pts',(0.00271248995295037,-0.0181135707687723,
-0.0133946193759434));
#17711=CARTESIAN_POINT('Ctrl Pts',(0.000440611520263108,-0.0179544484715537,
-0.0151167466905447));
#17712=CARTESIAN_POINT('Ctrl Pts',(-0.00223621102078284,-0.0177953261743351,
-0.0141360453169456));
#17713=CARTESIAN_POINT('Ctrl Pts',(-0.0028578433629701,-0.0176362038771165,
-0.0113538290543058));
#17714=CARTESIAN_POINT('Ctrl Pts',(-0.000852974174112536,-0.017477081579898,
-0.00932709433163266));
#17715=CARTESIAN_POINT('Ctrl Pts',(0.00193582110482348,-0.0173179592826795,
-0.00991851211257368));
#17716=CARTESIAN_POINT('Ctrl Pts',(0.00294549959933089,-0.0171588369854609,
-0.0125845397645564));
#17717=CARTESIAN_POINT('Ctrl Pts',(0.0012481160800549,-0.0169997146882424,
-0.0148749640238712));
#17718=CARTESIAN_POINT('Ctrl Pts',(-0.00159634877796926,-0.0168405923910238,
-0.0146847700063838));
#17719=CARTESIAN_POINT('Ctrl Pts',(-0.00297368896601409,-0.0166814700938053,
-0.0121887555574983));
#17720=CARTESIAN_POINT('Ctrl Pts',(-0.0016180596919498,-0.0165223477965867,
-0.00968088328102499));
#17721=CARTESIAN_POINT('Ctrl Pts',(0.00122464766355246,-0.0163632254993682,
-0.00946601368756258));
#17722=CARTESIAN_POINT('Ctrl Pts',(0.00294184235435476,-0.0162041032021496,
-0.0117416227629777));
#17723=CARTESIAN_POINT('Ctrl Pts',(0.00195533617961103,-0.016044980904931,
-0.0144163114361035));
#17724=CARTESIAN_POINT('Ctrl Pts',(-0.000828222026482802,-0.0158858586077125,
-0.0150319066925196));
#17725=CARTESIAN_POINT('Ctrl Pts',(-0.00285060277948614,-0.015726736310494,
-0.0130226452686618));
#17726=CARTESIAN_POINT('Ctrl Pts',(-0.00225313612580357,-0.0155676140132754,
-0.0102351399111969));
#17727=CARTESIAN_POINT('Ctrl Pts',(0.000415075089142231,-0.0154084917160569,
-0.00923124677194611));
#17728=CARTESIAN_POINT('Ctrl Pts',(0.00270181275207879,-0.0152493694188383,
-0.0109335964446202));
#17729=CARTESIAN_POINT('Ctrl Pts',(0.00250544630748153,-0.0150902471216198,
-0.0137776394034903));
#17730=CARTESIAN_POINT('Ctrl Pts',(6.45391018013059E-6,-0.0149311248244012,
-0.0151495666298162));
#17731=CARTESIAN_POINT('Ctrl Pts',(-0.00249847975875477,-0.0147720025271827,
-0.0137884899605927));
#17732=CARTESIAN_POINT('Ctrl Pts',(-0.0027071658355337,-0.0146128802299641,
-0.0109453428619918));
#17733=CARTESIAN_POINT('Ctrl Pts',(-0.0004278684125787,-0.0144537579327456,
-0.00923305019703428));
#17734=CARTESIAN_POINT('Ctrl Pts',(0.00224473583993033,-0.014294635635527,
-0.0102254324978796));
#17735=CARTESIAN_POINT('Ctrl Pts',(0.00285416927352115,-0.0141355133383085,
-0.0130101703438483));
#17736=CARTESIAN_POINT('Ctrl Pts',(0.000840764382058176,-0.0139763910410899,
-0.0150284806573225));
#17737=CARTESIAN_POINT('Ctrl Pts',(-0.00194590810912974,-0.0138172687438714,
-0.0144243922958196));
#17738=CARTESIAN_POINT('Ctrl Pts',(-0.00294308595084797,-0.0136581464466527,
-0.0117551416935859));
#17739=CARTESIAN_POINT('Ctrl Pts',(-0.0012376151811133,-0.0134990241494343,
-0.00946986735125886));
#17740=CARTESIAN_POINT('Ctrl Pts',(0.00161003820092075,-0.0133398897210256,
-0.00967693703946193));
#17741=CARTESIAN_POINT('Ctrl Pts',(0.00251423374407564,-0.0132337960583565,
-0.0113383961313303));
#17742=CARTESIAN_POINT('Ctrl Pts',(0.00251402688117483,-0.0131807431614265,
-0.0121764281640729));
#17743=CARTESIAN_POINT('Ctrl Pts',(-0.00132619774418405,-0.0271787743898765,
-0.0094032008032357));
#17744=CARTESIAN_POINT('Ctrl Pts',(-0.00123334707548279,-0.0271787743898774,
-0.00936860122999075));
#17745=CARTESIAN_POINT('Ctrl Pts',(-0.00113896878046653,-0.0271787743898777,
-0.00933897076543453));
#17746=CARTESIAN_POINT('Ctrl Pts',(-0.00104343428160282,-0.0271787743898779,
-0.0093141943241909));
#17747=CARTESIAN_POINT('Ctrl Pts',(-0.00076805930112476,-0.0271787743898785,
-0.00924277706545265));
#17748=CARTESIAN_POINT('Ctrl Pts',(-0.000483025747473507,-0.027178774389879,
-0.00921146057988075));
#17749=CARTESIAN_POINT('Ctrl Pts',(-0.000197232514694447,-0.0271787743898794,
-0.00921970998708291));
#17750=CARTESIAN_POINT('Ctrl Pts',(-0.000179613012251587,-0.0271787743898794,
-0.00922021857312932));
#17751=CARTESIAN_POINT('Ctrl Pts',(-0.000161988828498365,-0.0271787743898794,
-0.00922087869898021));
#17752=CARTESIAN_POINT('Ctrl Pts',(-0.000144384552395993,-0.0271787743898794,
-0.00922168930787544));
#17753=CARTESIAN_POINT('Ctrl Pts',(-4.51942574374791E-5,-0.0271787743898796,
-0.0092262566377075));
#17754=CARTESIAN_POINT('Ctrl Pts',(5.35197260388724E-5,-0.0271787743898787,
-0.00923560020302817));
#17755=CARTESIAN_POINT('Ctrl Pts',(0.000151386361355854,-0.0271787743898786,
-0.0092496540195405));
#17756=CARTESIAN_POINT('Ctrl Pts',(0.000344058415070921,-0.0271787743898783,
-0.00927732205657064));
#17757=CARTESIAN_POINT('Ctrl Pts',(0.000533476473635147,-0.027178774389878,
-0.00932320440058446));
#17758=CARTESIAN_POINT('Ctrl Pts',(0.000716581926211375,-0.0271787743898776,
-0.00938734742840202));
#17759=CARTESIAN_POINT('Ctrl Pts',(0.0007556805873622,-0.0271787743898775,
-0.00940104394303083));
#17760=CARTESIAN_POINT('Ctrl Pts',(0.000794489703590543,-0.0271787743898774,
-0.00941557553850965));
#17761=CARTESIAN_POINT('Ctrl Pts',(0.000832976258181437,-0.0271787743898773,
-0.00943094658771291));
#17762=CARTESIAN_POINT('Ctrl Pts',(0.000855095263786809,-0.0271787743898773,
-0.00943978064228344));
#17763=CARTESIAN_POINT('Ctrl Pts',(0.00087710770065419,-0.0271787743898772,
-0.00944889199559381));
#17764=CARTESIAN_POINT('Ctrl Pts',(0.000899007079087444,-0.0271787743898772,
-0.00945828167060659));
#17765=CARTESIAN_POINT('Ctrl Pts',(0.000915403294136593,-0.0271787743898772,
-0.00946531178478176));
#17766=CARTESIAN_POINT('Ctrl Pts',(0.000931738600316675,-0.0271787743898771,
-0.00947249914463924));
#17767=CARTESIAN_POINT('Ctrl Pts',(0.000947988260384964,-0.0271787743898771,
-0.00947983398932806));
#17768=CARTESIAN_POINT('Ctrl Pts',(0.00111836097776595,-0.0271787743898767,
-0.00955673759321582));
#17769=CARTESIAN_POINT('Ctrl Pts',(0.00127987164207508,-0.0271787743898763,
-0.00965001320728162));
#17770=CARTESIAN_POINT('Ctrl Pts',(0.00142972751227199,-0.0271787743898758,
-0.00975968542682677));
#17771=CARTESIAN_POINT('Ctrl Pts',(0.0014442192240037,-0.0271787743898758,
-0.00977029120548955));
#17772=CARTESIAN_POINT('Ctrl Pts',(0.00145860151389945,-0.0271787743898758,
-0.00978105080560855));
#17773=CARTESIAN_POINT('Ctrl Pts',(0.00147287155736277,-0.0271787743898757,
-0.00979196455368879));
#17774=CARTESIAN_POINT('Ctrl Pts',(0.00154855896912941,-0.0271787743898755,
-0.00984985038613137));
#17775=CARTESIAN_POINT('Ctrl Pts',(0.00162109245549692,-0.0271787743898753,
-0.00991207085484757));
#17776=CARTESIAN_POINT('Ctrl Pts',(0.00169026613585085,-0.0271787743898751,
-0.00997826337560861));
#17777=CARTESIAN_POINT('Ctrl Pts',(0.00171603724734808,-0.027178774389875,
-0.0100029238364094));
#17778=CARTESIAN_POINT('Ctrl Pts',(0.00174134154940518,-0.0271787743898749,
-0.0100281358260087));
#17779=CARTESIAN_POINT('Ctrl Pts',(0.00176616664819554,-0.0271787743898748,
-0.0100538811973334));
#17780=CARTESIAN_POINT('Ctrl Pts',(0.00177607355662899,-0.0271787743898748,
-0.0100641553573057));
#17781=CARTESIAN_POINT('Ctrl Pts',(0.00178590413828819,-0.0271787743898747,
-0.01007451446367));
#17782=CARTESIAN_POINT('Ctrl Pts',(0.00179565756092862,-0.0271787743898747,
-0.0100849573712734));
#17783=CARTESIAN_POINT('Ctrl Pts',(0.00180578442604608,-0.0271787743898747,
-0.0100958001205966));
#17784=CARTESIAN_POINT('Ctrl Pts',(0.00181582268481298,-0.0271787743898746,
-0.0101067274469139));
#17785=CARTESIAN_POINT('Ctrl Pts',(0.00182576793439398,-0.0271787743898746,
-0.0101177335422781));
#17786=CARTESIAN_POINT('Ctrl Pts',(0.00201260976483294,-0.027178774389874,
-0.0103245055279476));
#17787=CARTESIAN_POINT('Ctrl Pts',(0.00216737989308834,-0.0271787743898734,
-0.0105594160048695));
#17788=CARTESIAN_POINT('Ctrl Pts',(0.00228510901854104,-0.0271787743898728,
-0.0108129813847881));
#17789=CARTESIAN_POINT('Ctrl Pts',(0.00230305828244781,-0.0271787743898727,
-0.0108516405687774));
#17790=CARTESIAN_POINT('Ctrl Pts',(0.00232013895398843,-0.0271787743898726,
-0.010890735204995));
#17791=CARTESIAN_POINT('Ctrl Pts',(0.00233632486912502,-0.0271787743898725,
-0.0109302325471785));
#17792=CARTESIAN_POINT('Ctrl Pts',(0.00234257114675687,-0.0271787743898725,
-0.0109454748960304));
#17793=CARTESIAN_POINT('Ctrl Pts',(0.0023486848303271,-0.0271787743898725,
-0.0109607789757957));
#17794=CARTESIAN_POINT('Ctrl Pts',(0.00235466215265408,-0.0271787743898725,
-0.0109761373101646));
#17795=CARTESIAN_POINT('Ctrl Pts',(0.00242919330983191,-0.027178774389872,
-0.011167640188915));
#17796=CARTESIAN_POINT('Ctrl Pts',(0.0024822151522778,-0.0271787743898716,
-0.01136648020721));
#17797=CARTESIAN_POINT('Ctrl Pts',(0.00251112044339404,-0.0271787743898712,
-0.0115688122023905));
#17798=CARTESIAN_POINT('Ctrl Pts',(0.00251367237767708,-0.0271787743898712,
-0.0115866752971776));
#17799=CARTESIAN_POINT('Ctrl Pts',(0.00251603423918924,-0.0271787743898712,
-0.0116045574678031));
#17800=CARTESIAN_POINT('Ctrl Pts',(0.00251820375128431,-0.0271787743898711,
-0.0116224513576578));
#17801=CARTESIAN_POINT('Ctrl Pts',(0.00253875013258885,-0.0271787743898708,
-0.0117919155818088));
#17802=CARTESIAN_POINT('Ctrl Pts',(0.00254212787993046,-0.0271787743898705,
-0.011962581473446));
#17803=CARTESIAN_POINT('Ctrl Pts',(0.00252655408384864,-0.0271787743898702,
-0.0121321046600801));
#17804=CARTESIAN_POINT('Ctrl Pts',(0.00252521873542723,-0.0271787743898702,
-0.0121466401348273));
#17805=CARTESIAN_POINT('Ctrl Pts',(0.00252374357338409,-0.0271787743898702,
-0.0121611670509537));
#17806=CARTESIAN_POINT('Ctrl Pts',(0.00252212942997833,-0.0271787743898701,
-0.0121756837992191));
#17807=CARTESIAN_POINT('Origin',(0.,-0.00867877438987209,-0.012175853286558));
#17808=CARTESIAN_POINT('',(-0.0023,-0.00867877438987209,-0.012175853286558));
#17809=CARTESIAN_POINT('Origin',(0.,-0.0261787743898721,-0.0121758532865581));
#17810=CARTESIAN_POINT('',(-0.01115,-0.0261787743898724,-0.0121758532865581));
#17811=CARTESIAN_POINT('Origin',(0.,-0.0261787743898824,-0.0121758532865681));
#17812=CARTESIAN_POINT('',(0.00601982559920929,-0.0261787743898934,-0.012175853286558));
#17813=CARTESIAN_POINT('Origin',(0.,-0.0261787743898824,-0.0121758532865681));
#17814=CARTESIAN_POINT('Origin',(0.,-0.0236787743898721,-0.0121758532865581));
#17815=CARTESIAN_POINT('',(-0.01115,-0.0236787743898724,-0.0121758532865581));
#17816=CARTESIAN_POINT('Origin',(0.,-0.0236787743898824,-0.0121758532865681));
#17817=CARTESIAN_POINT('',(0.00588880615100169,-0.0236787743898934,-0.012175853286558));
#17818=CARTESIAN_POINT('Origin',(0.,-0.0236787743898824,-0.0121758532865681));
#17819=CARTESIAN_POINT('Origin',(0.,-0.0246787743898721,-0.0121758532865581));
#17820=CARTESIAN_POINT('',(-0.01115,-0.0246787743898924,-0.0121758532865581));
#17821=CARTESIAN_POINT('Origin',(0.,-0.0246787743898824,-0.0121758532865681));
#17822=CARTESIAN_POINT('',(0.00594121393028363,-0.0246787743898724,-0.012175853286558));
#17823=CARTESIAN_POINT('Origin',(0.,-0.0246787743898824,-0.0121758532865681));
#17824=CARTESIAN_POINT('Origin',(0.,-0.0211787743898721,-0.012175853286558));
#17825=CARTESIAN_POINT('',(-0.01115,-0.0211787743898724,-0.0121758532865581));
#17826=CARTESIAN_POINT('Origin',(0.,-0.0211787743898824,-0.012175853286568));
#17827=CARTESIAN_POINT('',(0.00575778670279409,-0.0211787743898934,-0.012175853286558));
#17828=CARTESIAN_POINT('Origin',(0.,-0.0211787743898824,-0.012175853286568));
#17829=CARTESIAN_POINT('Origin',(0.,-0.0221787743898721,-0.0121758532865581));
#17830=CARTESIAN_POINT('',(-0.01115,-0.0221787743898924,-0.0121758532865581));
#17831=CARTESIAN_POINT('Origin',(0.,-0.0221787743898824,-0.0121758532865681));
#17832=CARTESIAN_POINT('',(0.00581019448207603,-0.0221787743898724,-0.012175853286558));
#17833=CARTESIAN_POINT('Origin',(0.,-0.0221787743898824,-0.0121758532865681));
#17834=CARTESIAN_POINT('Origin',(0.,-0.0186787743898721,-0.012175853286558));
#17835=CARTESIAN_POINT('',(-0.01115,-0.0186787743898724,-0.012175853286558));
#17836=CARTESIAN_POINT('Origin',(0.,-0.0186787743898824,-0.012175853286568));
#17837=CARTESIAN_POINT('',(0.00562676725458648,-0.0186787743898934,-0.012175853286558));
#17838=CARTESIAN_POINT('Origin',(0.,-0.0186787743898824,-0.012175853286568));
#17839=CARTESIAN_POINT('Origin',(0.,-0.0196787743898721,-0.012175853286558));
#17840=CARTESIAN_POINT('',(-0.01115,-0.0196787743898924,-0.012175853286558));
#17841=CARTESIAN_POINT('Origin',(0.,-0.0196787743898824,-0.012175853286568));
#17842=CARTESIAN_POINT('',(0.00567917503386843,-0.0196787743898724,-0.012175853286558));
#17843=CARTESIAN_POINT('Origin',(0.,-0.0196787743898824,-0.012175853286568));
#17844=CARTESIAN_POINT('Origin',(0.,-0.0161787743898721,-0.012175853286558));
#17845=CARTESIAN_POINT('',(-0.01115,-0.0161787743898724,-0.012175853286558));
#17846=CARTESIAN_POINT('Origin',(0.,-0.0161787743898824,-0.012175853286568));
#17847=CARTESIAN_POINT('',(0.00549574780637888,-0.0161787743898934,-0.012175853286558));
#17848=CARTESIAN_POINT('Origin',(0.,-0.0161787743898824,-0.012175853286568));
#17849=CARTESIAN_POINT('Origin',(0.,-0.0171787743898721,-0.012175853286558));
#17850=CARTESIAN_POINT('',(-0.01115,-0.0171787743898924,-0.012175853286558));
#17851=CARTESIAN_POINT('Origin',(0.,-0.0171787743898824,-0.012175853286568));
#17852=CARTESIAN_POINT('',(0.00554815558566082,-0.0171787743898724,-0.012175853286558));
#17853=CARTESIAN_POINT('Origin',(0.,-0.0171787743898824,-0.012175853286568));
#17854=CARTESIAN_POINT('Origin',(0.,-0.0136787743898721,-0.012175853286558));
#17855=CARTESIAN_POINT('',(-0.01115,-0.0136787743898724,-0.012175853286558));
#17856=CARTESIAN_POINT('Origin',(0.,-0.0136787743898824,-0.012175853286568));
#17857=CARTESIAN_POINT('',(0.00536472835817128,-0.0136787743898934,-0.012175853286558));
#17858=CARTESIAN_POINT('Origin',(0.,-0.0136787743898824,-0.012175853286568));
#17859=CARTESIAN_POINT('Origin',(0.,-0.0146787743898721,-0.012175853286558));
#17860=CARTESIAN_POINT('',(-0.01115,-0.0146787743898924,-0.012175853286558));
#17861=CARTESIAN_POINT('Origin',(0.,-0.0146787743898824,-0.012175853286568));
#17862=CARTESIAN_POINT('',(0.00541713613745322,-0.0146787743898724,-0.012175853286558));
#17863=CARTESIAN_POINT('Origin',(0.,-0.0146787743898824,-0.012175853286568));
#17864=CARTESIAN_POINT('Origin',(0.,-0.0111787743898721,-0.012175853286558));
#17865=CARTESIAN_POINT('',(0.01115,-0.0111787743898724,-0.012175853286558));
#17866=CARTESIAN_POINT('Origin',(0.,-0.0111787743898824,-0.012175853286568));
#17867=CARTESIAN_POINT('',(0.00523370890996368,-0.0111787743898934,-0.012175853286558));
#17868=CARTESIAN_POINT('Origin',(0.,-0.0111787743898824,-0.012175853286568));
#17869=CARTESIAN_POINT('Origin',(0.,-0.0121787743898721,-0.012175853286558));
#17870=CARTESIAN_POINT('',(0.01115,-0.0121787743898924,-0.012175853286558));
#17871=CARTESIAN_POINT('Origin',(0.,-0.0121787743898824,-0.012175853286568));
#17872=CARTESIAN_POINT('',(0.00528611668924562,-0.0121787743898724,-0.012175853286558));
#17873=CARTESIAN_POINT('Origin',(0.,-0.0121787743898824,-0.012175853286568));
#17874=CARTESIAN_POINT('Origin',(0.,-0.00967877438987209,-0.012175853286558));
#17875=CARTESIAN_POINT('',(0.01115,-0.00967877438989238,-0.012175853286558));
#17876=CARTESIAN_POINT('Origin',(0.,-0.00967877438988238,-0.012175853286568));
#17877=CARTESIAN_POINT('',(0.00515509724103801,-0.00967877438987238,-0.012175853286558));
#17878=CARTESIAN_POINT('Origin',(0.,-0.00967877438988238,-0.012175853286568));
#17879=CARTESIAN_POINT('Origin',(0.,-0.00867877438987209,-0.012175853286558));
#17880=CARTESIAN_POINT('',(0.01115,-0.00867877438987238,-0.012175853286558));
#17881=CARTESIAN_POINT('Origin',(0.,-0.00867877438988238,-0.012175853286568));
#17882=CARTESIAN_POINT('',(0.00510268946175607,-0.00867877438989337,-0.012175853286558));
#17883=CARTESIAN_POINT('Origin',(0.,-0.00867877438988238,-0.012175853286568));
#17884=CARTESIAN_POINT('Origin',(0.,-0.0266787743898721,-0.0121758532865581));
#17885=CARTESIAN_POINT('',(-0.01115,-0.0271787743898924,-0.0121758532865581));
#17886=CARTESIAN_POINT('Origin',(0.,-0.0271787743898824,-0.0121758532865681));
#17887=CARTESIAN_POINT('',(-0.01115,-0.0266787743898721,-0.0121758532865581));
#17888=CARTESIAN_POINT('Origin',(0.,-0.0241787743898721,-0.0121758532865581));
#17889=CARTESIAN_POINT('',(-0.01115,-0.0241787743898721,-0.0121758532865581));
#17890=CARTESIAN_POINT('Origin',(0.,-0.0216787743898721,-0.0121758532865581));
#17891=CARTESIAN_POINT('',(-0.01115,-0.0216787743898721,-0.0121758532865581));
#17892=CARTESIAN_POINT('Origin',(0.,-0.0191787743898721,-0.012175853286558));
#17893=CARTESIAN_POINT('',(-0.01115,-0.0191787743898721,-0.012175853286558));
#17894=CARTESIAN_POINT('Origin',(0.,-0.0166787743898721,-0.012175853286558));
#17895=CARTESIAN_POINT('',(-0.01115,-0.0166787743898721,-0.012175853286558));
#17896=CARTESIAN_POINT('Origin',(0.,-0.0141787743898721,-0.012175853286558));
#17897=CARTESIAN_POINT('',(-0.01115,-0.0141787743898721,-0.012175853286558));
#17898=CARTESIAN_POINT('Origin',(0.,-0.0111787743898721,-0.012175853286558));
#17899=CARTESIAN_POINT('',(0.01115,-0.0111787743898721,-0.012175853286558));
#17900=CARTESIAN_POINT('Origin',(0.,-0.00867877438987209,-0.012175853286558));
#17901=CARTESIAN_POINT('',(0.01115,-0.00867877438987209,-0.012175853286558));
#17902=CARTESIAN_POINT('Origin',(0.,0.00282122561012762,-0.012175853286558));
#17903=CARTESIAN_POINT('',(0.00502407779283041,-0.00717877438987238,-0.012175853286558));
#17904=CARTESIAN_POINT('',(0.0045,0.00282122561012762,-0.012175853286558));
#17905=CARTESIAN_POINT('Origin',(0.,-0.00717877438988238,-0.012175853286568));
#17906=CARTESIAN_POINT('Origin',(0.,0.00282122561012762,-0.012175853286558));
#17907=CARTESIAN_POINT('',(0.0045,0.00282122561012762,-0.012175853286558));
#17908=CARTESIAN_POINT('Origin',(0.,0.00282122561012762,-0.012175853286558));
#17909=CARTESIAN_POINT('',(0.0045,0.00282122561012762,-0.012175853286558));
#17910=CARTESIAN_POINT('Origin',(0.,0.00282122561012762,-0.012175853286558));
#17911=CARTESIAN_POINT('',(0.0045,0.00282122561012762,-0.012175853286558));
#17912=CARTESIAN_POINT('Origin',(0.,0.00282122561012762,-0.012175853286558));
#17913=CARTESIAN_POINT('',(0.0045,0.00282122561012762,-0.012175853286558));
#17914=CARTESIAN_POINT('Origin',(0.,0.00282122561012762,-0.012175853286558));
#17915=CARTESIAN_POINT('',(0.0045,0.00282122561012762,-0.012175853286558));
#17916=CARTESIAN_POINT('Origin',(0.,0.00282122561012762,-0.012175853286558));
#17917=CARTESIAN_POINT('',(0.0045,0.00282122561012762,-0.012175853286558));
#17918=CARTESIAN_POINT('Origin',(0.,-0.0271787743898721,-0.0121758532865581));
#17919=CARTESIAN_POINT('Origin',(0.,0.00282122561012762,-0.012175853286558));
#17920=CARTESIAN_POINT('',(0.00470963111713326,-0.00117877438989337,-0.012175853286558));
#17921=CARTESIAN_POINT('Origin',(0.,-0.00117877438988238,-0.012175853286568));
#17922=CARTESIAN_POINT('',(0.0046310194482076,0.000321225610127617,-0.012175853286558));
#17923=CARTESIAN_POINT('',(0.0045,0.00282122561012762,-0.012175853286558));
#17924=CARTESIAN_POINT('Origin',(0.,0.000321225610117618,-0.012175853286568));
#17925=CARTESIAN_POINT('Origin',(0.,0.00282122561012762,-0.012175853286558));
#17926=CARTESIAN_POINT('',(0.00457861166892566,0.00132122561010662,-0.012175853286558));
#17927=CARTESIAN_POINT('Origin',(0.,0.00132122561011761,-0.012175853286568));
#17928=CARTESIAN_POINT('',(0.0045,0.00282122561012761,-0.012175853286558));
#17929=CARTESIAN_POINT('',(0.0045,0.00282122561012762,-0.012175853286558));
#17930=CARTESIAN_POINT('Origin',(0.,0.00282122561011761,-0.012175853286568));
#17931=CARTESIAN_POINT('Origin',(0.,0.00282122561012762,-0.012175853286558));
#17932=CARTESIAN_POINT('',(0.00484065056534087,-0.00367877438989337,-0.012175853286558));
#17933=CARTESIAN_POINT('Origin',(0.,-0.00367877438988238,-0.012175853286568));
#17934=CARTESIAN_POINT('',(0.0047620388964152,-0.00217877438987238,-0.012175853286558));
#17935=CARTESIAN_POINT('',(0.0045,0.00282122561012762,-0.012175853286558));
#17936=CARTESIAN_POINT('Origin',(0.,-0.00217877438988238,-0.012175853286568));
#17937=CARTESIAN_POINT('Origin',(0.,0.00282122561012762,-0.012175853286558));
#17938=CARTESIAN_POINT('',(0.00497167001354847,-0.00617877438989337,-0.012175853286558));
#17939=CARTESIAN_POINT('Origin',(0.,-0.00617877438988238,-0.012175853286568));
#17940=CARTESIAN_POINT('',(0.00489305834462281,-0.00467877438987239,-0.012175853286558));
#17941=CARTESIAN_POINT('',(0.0045,0.00282122561012762,-0.012175853286558));
#17942=CARTESIAN_POINT('Origin',(0.,-0.00467877438988239,-0.012175853286568));
#17943=CARTESIAN_POINT('Origin',(0.,0.00282122561012762,-0.012175853286558));
#17944=CARTESIAN_POINT('',(0.0045,0.00282122561012762,-0.012175853286558));
#17945=CARTESIAN_POINT('Origin',(0.,-0.00617877438987208,-0.012175853286558));
#17946=CARTESIAN_POINT('',(0.01115,-0.00617877438987238,-0.012175853286558));
#17947=CARTESIAN_POINT('Origin',(0.,-0.00617877438988238,-0.012175853286568));
#17948=CARTESIAN_POINT('Origin',(0.,-0.00617877438987208,-0.012175853286558));
#17949=CARTESIAN_POINT('',(0.01115,-0.00717877438989238,-0.012175853286558));
#17950=CARTESIAN_POINT('Origin',(0.,-0.00717877438988238,-0.012175853286568));
#17951=CARTESIAN_POINT('',(0.01115,-0.00617877438987208,-0.012175853286558));
#17952=CARTESIAN_POINT('Origin',(0.,-0.00717877438987209,-0.012175853286558));
#17953=CARTESIAN_POINT('Origin',(0.,-0.00367877438987208,-0.012175853286558));
#17954=CARTESIAN_POINT('',(0.01115,-0.00367877438987238,-0.012175853286558));
#17955=CARTESIAN_POINT('Origin',(0.,-0.00367877438988238,-0.012175853286568));
#17956=CARTESIAN_POINT('Origin',(0.,-0.00367877438987208,-0.012175853286558));
#17957=CARTESIAN_POINT('',(0.01115,-0.00467877438989239,-0.012175853286558));
#17958=CARTESIAN_POINT('Origin',(0.,-0.00467877438988239,-0.012175853286568));
#17959=CARTESIAN_POINT('',(0.01115,-0.00367877438987208,-0.012175853286558));
#17960=CARTESIAN_POINT('Origin',(0.,-0.00467877438987209,-0.012175853286558));
#17961=CARTESIAN_POINT('Origin',(0.,-0.00117877438987208,-0.012175853286558));
#17962=CARTESIAN_POINT('',(0.01115,-0.00117877438987238,-0.012175853286558));
#17963=CARTESIAN_POINT('Origin',(0.,-0.00117877438988238,-0.012175853286568));
#17964=CARTESIAN_POINT('Origin',(0.,-0.00117877438987208,-0.012175853286558));
#17965=CARTESIAN_POINT('',(0.01115,-0.00217877438989238,-0.012175853286558));
#17966=CARTESIAN_POINT('Origin',(0.,-0.00217877438988238,-0.012175853286568));
#17967=CARTESIAN_POINT('',(0.01115,-0.00117877438987208,-0.012175853286558));
#17968=CARTESIAN_POINT('Origin',(0.,-0.00217877438987208,-0.012175853286558));
#17969=CARTESIAN_POINT('Origin',(0.,0.00132122561012792,-0.012175853286558));
#17970=CARTESIAN_POINT('',(0.008,0.00132122561012761,-0.012175853286558));
#17971=CARTESIAN_POINT('Origin',(0.,0.00132122561011761,-0.012175853286568));
#17972=CARTESIAN_POINT('Origin',(0.,0.00132122561012792,-0.012175853286558));
#17973=CARTESIAN_POINT('',(0.008,0.000321225610107618,-0.012175853286558));
#17974=CARTESIAN_POINT('Origin',(0.,0.000321225610117618,-0.012175853286568));
#17975=CARTESIAN_POINT('',(0.008,0.00132122561012792,-0.012175853286558));
#17976=CARTESIAN_POINT('Origin',(0.,0.000321225610127919,-0.012175853286558));
#17977=CARTESIAN_POINT('Origin',(0.,0.00582122561012762,-0.012175853286558));
#17978=CARTESIAN_POINT('',(0.008,0.00582122561012762,-0.012175853286558));
#17979=CARTESIAN_POINT('Origin',(0.,0.00582122561011762,-0.012175853286568));
#17980=CARTESIAN_POINT('',(0.006,0.00582122561010762,-0.012175853286558));
#17981=CARTESIAN_POINT('Origin',(0.,0.00582122561011762,-0.012175853286568));
#17982=CARTESIAN_POINT('Origin',(0.,0.00582122561012762,-0.012175853286558));
#17983=CARTESIAN_POINT('',(0.008,0.00282122561010761,-0.012175853286558));
#17984=CARTESIAN_POINT('Origin',(0.,0.00282122561011761,-0.012175853286568));
#17985=CARTESIAN_POINT('',(0.008,0.00582122561012762,-0.012175853286558));
#17986=CARTESIAN_POINT('Origin',(0.,0.00282122561012762,-0.012175853286558));
#17987=CARTESIAN_POINT('Origin',(0.,0.0118212256101276,-0.012175853286558));
#17988=CARTESIAN_POINT('',(0.006,0.0118212256101276,-0.012175853286558));
#50043=UNCERTAINTY_MEASURE_WITH_UNIT(LENGTH_MEASURE(1.E-5),#50082,
'DISTANCE_ACCURACY_VALUE',
'Maximum model space distance between geometric entities at asserted c
onnectivities');
#50059=UNCERTAINTY_MEASURE_WITH_UNIT(LENGTH_MEASURE(1.E-5),#50082,
'DISTANCE_ACCURACY_VALUE',
'Maximum model space distance between geometric entities at asserted c
onnectivities');
#50065=(
GEOMETRIC_REPRESENTATION_CONTEXT(3)
GLOBAL_UNCERTAINTY_ASSIGNED_CONTEXT((#50043))
GLOBAL_UNIT_ASSIGNED_CONTEXT((#50082,#50083,#50084))
REPRESENTATION_CONTEXT('','3D')
);
#50081=(
GEOMETRIC_REPRESENTATION_CONTEXT(3)
GLOBAL_UNCERTAINTY_ASSIGNED_CONTEXT((#50059))
GLOBAL_UNIT_ASSIGNED_CONTEXT((#50082,#50083,#50084))
REPRESENTATION_CONTEXT('','3D')
);
#50082=(
LENGTH_UNIT()
NAMED_UNIT(*)
SI_UNIT($,.METRE.)
);
#50083=(
NAMED_UNIT(*)
PLANE_ANGLE_UNIT()
SI_UNIT($,.RADIAN.)
);
#50084=(
NAMED_UNIT(*)
SI_UNIT($,.STERADIAN.)
SOLID_ANGLE_UNIT()
);
#50090=SHAPE_DEFINITION_REPRESENTATION(#50111,#50152);
#50111=PRODUCT_DEFINITION_SHAPE('',$,#50174);
#50152=SHAPE_REPRESENTATION('',(#10265),#50065);
#50168=PRODUCT_DEFINITION_CONTEXT('part definition',#50233,'design');
#50174=PRODUCT_DEFINITION('Heatsink','Heatsink',#50195,#50168);
#50195=PRODUCT_DEFINITION_FORMATION('',$,#50240);
#50233=APPLICATION_CONTEXT('Managed model based 3d engineering');
#50234=PRODUCT_CONTEXT('part definition',#50233,'mechanical');
#50240=PRODUCT('Heatsink','Heatsink',
'LEGAL AND USAGE DISCLAIMER: this Data/Model is provided \X2\201C\X0\A
S IS\X2\201D\X0\ for informational and representational only. It is a 
geometric approximation and is NOT engineered, certified, or guarantee
d for dimensional accuracy, exact tolerances, or production-level prec
ision. Vendor disclaims all implied warranties including fitness for a
 particular purpose. DO NOT USE FOR DIRECT PHYSICAL MANUFACTURING, AUT
OMATED PRODUCTION, OR SAFETY-CRITICAL SYSTEMS without independent engi
neering verification and resolution of any design discrepancies.',(#50234));
#50261=PRESENTATION_STYLE_ASSIGNMENT((#50268));
#50268=SURFACE_STYLE_USAGE(.BOTH.,#50275);
#50275=SURFACE_SIDE_STYLE('',(#50282));
#50282=SURFACE_STYLE_FILL_AREA(#50289);
#50289=FILL_AREA_STYLE('Opaque(179,179,179)',(#50296));
#50296=FILL_AREA_STYLE_COLOUR('Opaque(179,179,179)',#50303);
#50303=COLOUR_RGB('Opaque(179,179,179)',0.701960784313725,0.701960784313725,
0.701960784313725);
ENDSEC;
END-ISO-10303-21;
